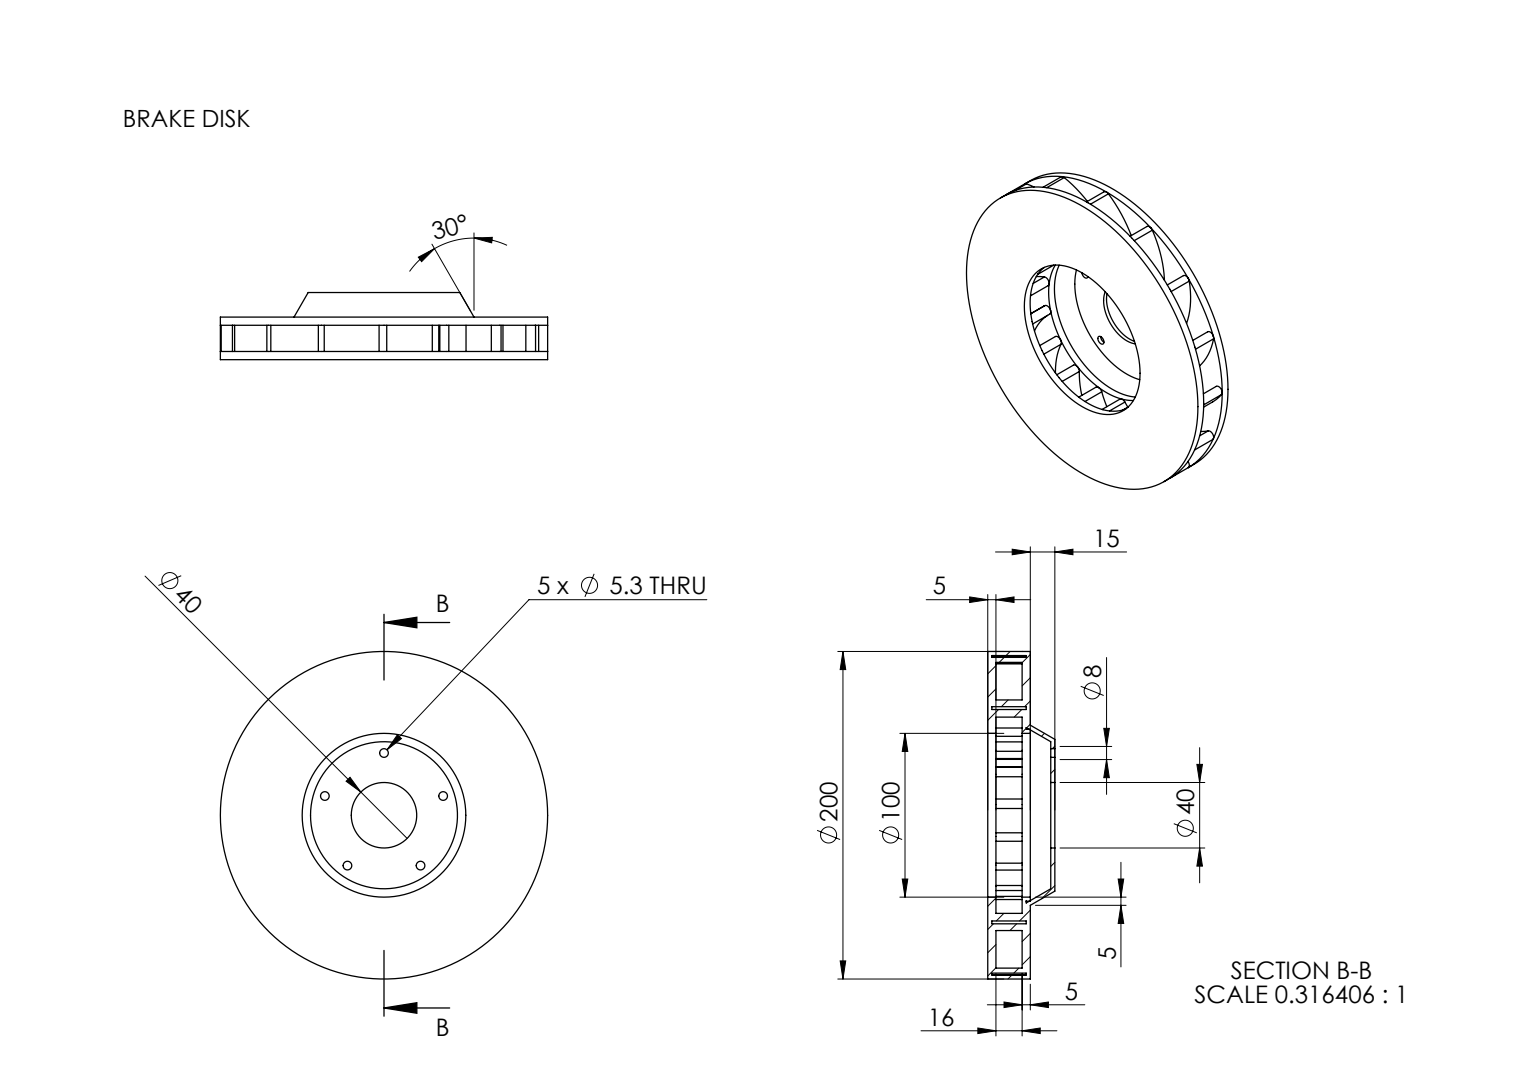
ISO-10303-21;
HEADER;
FILE_DESCRIPTION (('STEP AP214'),
    '1' );
FILE_NAME ('brake disk.step',
    '2026-10-02T06:35:35',
    ( '' ),
    ( '' ),
    'SwSTEP 2.0',
    'SolidWorks 2026',
    '' );
FILE_SCHEMA (( 'AUTOMOTIVE_DESIGN' ));
ENDSEC;

DATA;
#3=DIRECTION ( 'NONE',  ( -1.000000000000000000, 0.000000000000000000, 0.000000000000000000 ) ) ;
#4=ORIENTED_EDGE ( 'NONE', *, *, #5380, .F. ) ;
#6=CIRCLE ( 'NONE', #12861, 63.00000000000000000 ) ;
#7=CARTESIAN_POINT ( 'NONE',  ( 53.06332297728253877, -7.252293700256950082, -10.50000000000000000 ) ) ;
#8=FACE_OUTER_BOUND ( 'NONE', #11130, .T. ) ;
#10=CIRCLE ( 'NONE', #12379, 59.50000000000000711 ) ;
#11=CARTESIAN_POINT ( 'NONE',  ( 0.000000000000000000, 0.000000000000000000, -10.50000000000000000 ) ) ;
#12=AXIS2_PLACEMENT_3D ( 'NONE', #10324, #12760, #3495 ) ;
#13=DIRECTION ( 'NONE',  ( -1.000000000000000000, 0.000000000000000000, 0.000000000000000000 ) ) ;
#14=VERTEX_POINT ( 'NONE', #5600 ) ;
#16=CARTESIAN_POINT ( 'NONE',  ( -9.706953719245875689, -57.06275842387046993, 10.49999999999999822 ) ) ;
#18=AXIS2_PLACEMENT_3D ( 'NONE', #11160, #14736, #14806 ) ;
#19=DIRECTION ( 'NONE',  ( 0.000000000000000000, 0.000000000000000000, 1.000000000000000000 ) ) ;
#20=CIRCLE ( 'NONE', #4639, 50.00000000000000000 ) ;
#25=CARTESIAN_POINT ( 'NONE',  ( -57.06275842387042729, 9.706953719246069312, 10.49999999999999822 ) ) ;
#29=DIRECTION ( 'NONE',  ( 1.000000000000000000, 0.000000000000000000, 0.000000000000000000 ) ) ;
#30=AXIS2_PLACEMENT_3D ( 'NONE', #3946, #7114, #5981 ) ;
#31=DIRECTION ( 'NONE',  ( 1.000000000000000000, 0.000000000000000000, 0.000000000000000000 ) ) ;
#32=DIRECTION ( 'NONE',  ( -1.000000000000000000, 0.000000000000000000, 0.000000000000000000 ) ) ;
#33=AXIS2_PLACEMENT_3D ( 'NONE', #14453, #639, #4058 ) ;
#34=EDGE_LOOP ( 'NONE', ( #1936, #8130, #14973, #10499, #11470, #9709, #14107 ) ) ;
#38=DIRECTION ( 'NONE',  ( -0.000000000000000000, -0.000000000000000000, -1.000000000000000000 ) ) ;
#39=ORIENTED_EDGE ( 'NONE', *, *, #13925, .F. ) ;
#40=AXIS2_PLACEMENT_3D ( 'NONE', #3441, #1165, #12924 ) ;
#41=EDGE_LOOP ( 'NONE', ( #8481, #11440, #8445, #13506, #14760, #3452, #6224, #9398, #1796 ) ) ;
#42=EDGE_CURVE ( 'NONE', #5654, #12729, #7938, .T. ) ;
#43=EDGE_CURVE ( 'NONE', #8906, #2094, #9864, .T. ) ;
#45=AXIS2_PLACEMENT_3D ( 'NONE', #573, #4845, #14470 ) ;
#46=CYLINDRICAL_SURFACE ( 'NONE', #4967, 3.000000000000002665 ) ;
#50=DIRECTION ( 'NONE',  ( 0.000000000000000000, 0.000000000000000000, 1.000000000000000000 ) ) ;
#51=EDGE_LOOP ( 'NONE', ( #11368, #1318, #14890, #12577, #3403 ) ) ;
#53=DIRECTION ( 'NONE',  ( 1.000000000000000000, 0.000000000000000000, 0.000000000000000000 ) ) ;
#54=AXIS2_PLACEMENT_3D ( 'NONE', #13528, #11036, #940 ) ;
#55=ORIENTED_EDGE ( 'NONE', *, *, #8567, .F. ) ;
#56=ORIENTED_EDGE ( 'NONE', *, *, #8508, .F. ) ;
#57=DIRECTION ( 'NONE',  ( 0.000000000000000000, 0.000000000000000000, 1.000000000000000000 ) ) ;
#58=ORIENTED_EDGE ( 'NONE', *, *, #13027, .F. ) ;
#59=AXIS2_PLACEMENT_3D ( 'NONE', #11530, #114, #4460 ) ;
#60=CARTESIAN_POINT ( 'NONE',  ( -69.16568774265545017, 71.53347797788843820, -13.00000000000000178 ) ) ;
#61=CARTESIAN_POINT ( 'NONE',  ( 0.000000000000000000, 0.000000000000000000, -10.50000000000000000 ) ) ;
#62=EDGE_CURVE ( 'NONE', #7405, #1485, #13775, .T. ) ;
#65=CARTESIAN_POINT ( 'NONE',  ( 0.000000000000000000, 0.000000000000000000, -13.00000000000000178 ) ) ;
#66=VECTOR ( 'NONE', #7777, 1000.000000000000000 ) ;
#67=CARTESIAN_POINT ( 'NONE',  ( 66.70695371924546180, 57.06275842387054098, 8.000000000000000000 ) ) ;
#68=CARTESIAN_POINT ( 'NONE',  ( 50.84834283436990177, 14.07862063237912054, -13.00000000000000178 ) ) ;
#70=ORIENTED_EDGE ( 'NONE', *, *, #7162, .T. ) ;
#72=AXIS2_PLACEMENT_3D ( 'NONE', #14916, #10416, #5859 ) ;
#74=LINE ( 'NONE', #12542, #3120 ) ;
#77=AXIS2_PLACEMENT_3D ( 'NONE', #3248, #7868, #12355 ) ;
#78=DIRECTION ( 'NONE',  ( 1.000000000000000000, 0.000000000000000000, 0.000000000000000000 ) ) ;
#79=EDGE_LOOP ( 'NONE', ( #12586, #8672, #6412, #11812, #13520, #7331 ) ) ;
#80=CYLINDRICAL_SURFACE ( 'NONE', #13351, 59.50000000000000000 ) ;
#81=EDGE_CURVE ( 'NONE', #7416, #8383, #7204, .T. ) ;
#83=EDGE_CURVE ( 'NONE', #7502, #10004, #12318, .T. ) ;
#84=DIRECTION ( 'NONE',  ( 0.000000000000000000, 0.000000000000000000, 1.000000000000000000 ) ) ;
#85=CYLINDRICAL_SURFACE ( 'NONE', #14315, 56.99999999999999289 ) ;
#90=ORIENTED_EDGE ( 'NONE', *, *, #1930, .F. ) ;
#96=DIRECTION ( 'NONE',  ( 0.000000000000000000, 0.000000000000000000, -1.000000000000000000 ) ) ;
#98=CIRCLE ( 'NONE', #1556, 2.649999999999992806 ) ;
#100=FACE_OUTER_BOUND ( 'NONE', #3263, .T. ) ;
#102=ORIENTED_EDGE ( 'NONE', *, *, #4360, .F. ) ;
#106=DIRECTION ( 'NONE',  ( -0.000000000000000000, -0.000000000000000000, 1.000000000000000000 ) ) ;
#108=EDGE_LOOP ( 'NONE', ( #5288, #10008 ) ) ;
#109=CIRCLE ( 'NONE', #11524, 3.000000000000004441 ) ;
#110=AXIS2_PLACEMENT_3D ( 'NONE', #13113, #9527, #4007 ) ;
#112=DIRECTION ( 'NONE',  ( 0.000000000000000000, 0.000000000000000000, -1.000000000000000000 ) ) ;
#113=AXIS2_PLACEMENT_3D ( 'NONE', #5450, #3170, #7481 ) ;
#114=DIRECTION ( 'NONE',  ( -0.000000000000000000, -0.000000000000000000, -1.000000000000000000 ) ) ;
#115=ORIENTED_EDGE ( 'NONE', *, *, #13152, .T. ) ;
#116=ORIENTED_EDGE ( 'NONE', *, *, #9973, .T. ) ;
#117=STYLED_ITEM ( 'NONE', ( #11100 ), #4169 ) ;
#118=ORIENTED_EDGE ( 'NONE', *, *, #6384, .T. ) ;
#119=AXIS2_PLACEMENT_3D ( 'NONE', #2152, #13621, #8984 ) ;
#120=DIRECTION ( 'NONE',  ( -1.000000000000000000, 0.000000000000000000, 0.000000000000000000 ) ) ;
#124=CARTESIAN_POINT ( 'NONE',  ( 7.417888187663120192, 52.54657765281190507, -13.00000000000000178 ) ) ;
#125=EDGE_CURVE ( 'NONE', #6463, #5657, #11381, .T. ) ;
#129=ADVANCED_FACE ( 'NONE', ( #13654 ), #8723, .F. ) ;
#130=ORIENTED_EDGE ( 'NONE', *, *, #424, .F. ) ;
#131=EDGE_CURVE ( 'NONE', #9943, #5635, #9786, .T. ) ;
#132=VERTEX_POINT ( 'NONE', #14438 ) ;
#133=EDGE_CURVE ( 'NONE', #4919, #1677, #14989, .T. ) ;
#136=CIRCLE ( 'NONE', #11783, 63.00000000000000000 ) ;
#139=CIRCLE ( 'NONE', #6147, 3.000000000000002665 ) ;
#140=EDGE_LOOP ( 'NONE', ( #7272, #903, #5586, #9223, #6785, #6818 ) ) ;
#142=EDGE_CURVE ( 'NONE', #2335, #4523, #8651, .T. ) ;
#144=VECTOR ( 'NONE', #4829, 1000.000000000000000 ) ;
#145=DIRECTION ( 'NONE',  ( -0.000000000000000000, -0.000000000000000000, 1.000000000000000000 ) ) ;
#146=DIRECTION ( 'NONE',  ( -1.000000000000000000, 0.000000000000000000, 0.000000000000000000 ) ) ;
#147=CIRCLE ( 'NONE', #10081, 0.5000000000000004441 ) ;
#148=DIRECTION ( 'NONE',  ( 1.000000000000000000, 0.000000000000000000, 0.000000000000000000 ) ) ;
#149=SURFACE_STYLE_FILL_AREA ( #5069 ) ;
#151=DIRECTION ( 'NONE',  ( 0.000000000000000000, 0.000000000000000000, 1.000000000000000000 ) ) ;
#152=ORIENTED_EDGE ( 'NONE', *, *, #3887, .F. ) ;
#153=DIRECTION ( 'NONE',  ( -1.000000000000000000, 0.000000000000000000, 0.000000000000000000 ) ) ;
#156=ORIENTED_EDGE ( 'NONE', *, *, #4969, .T. ) ;
#158=ORIENTED_EDGE ( 'NONE', *, *, #13672, .T. ) ;
#160=ORIENTED_EDGE ( 'NONE', *, *, #4028, .F. ) ;
#162=CARTESIAN_POINT ( 'NONE',  ( -52.72775723226775568, 7.383907457638128058, -13.00000000000000178 ) ) ;
#163=DIRECTION ( 'NONE',  ( 1.000000000000000000, 0.000000000000000000, 0.000000000000000000 ) ) ;
#164=CARTESIAN_POINT ( 'NONE',  ( -53.63365512954686665, 9.714003807514082212, 8.000000000000000000 ) ) ;
#165=AXIS2_PLACEMENT_3D ( 'NONE', #7612, #12181, #14531 ) ;
#166=DIRECTION ( 'NONE',  ( -0.000000000000000000, -0.000000000000000000, -1.000000000000000000 ) ) ;
#167=CARTESIAN_POINT ( 'NONE',  ( 36.14014761921570340, 11.74264578624841171, -28.00000000000000000 ) ) ;
#168=ORIENTED_EDGE ( 'NONE', *, *, #2760, .F. ) ;
#169=CARTESIAN_POINT ( 'NONE',  ( 0.000000000000000000, 0.000000000000000000, -10.50000000000000000 ) ) ;
#170=DIRECTION ( 'NONE',  ( 1.000000000000000000, 0.000000000000000000, 0.000000000000000000 ) ) ;
#171=EDGE_CURVE ( 'NONE', #8488, #2518, #8671, .T. ) ;
#172=EDGE_CURVE ( 'NONE', #8464, #345, #2401, .T. ) ;
#174=CARTESIAN_POINT ( 'NONE',  ( 33.48561063518626923, -47.21331623427104063, 10.49999999999999822 ) ) ;
#175=ORIENTED_EDGE ( 'NONE', *, *, #2159, .T. ) ;
#176=CARTESIAN_POINT ( 'NONE',  ( -45.96504489225991819, 23.50071946824089153, -8.000000000000000000 ) ) ;
#178=DIRECTION ( 'NONE',  ( 1.000000000000000000, 0.000000000000000000, -0.000000000000000000 ) ) ;
#180=EDGE_CURVE ( 'NONE', #2333, #2935, #11831, .T. ) ;
#181=CARTESIAN_POINT ( 'NONE',  ( 70.71067811865488295, 70.71067811865464137, 8.000000000000000000 ) ) ;
#182=DIRECTION ( 'NONE',  ( -0.000000000000000000, -0.000000000000000000, -1.000000000000000000 ) ) ;
#184=PLANE ( 'NONE',  #4038 ) ;
#185=DIRECTION ( 'NONE',  ( 1.000000000000000000, 0.000000000000000000, 0.000000000000000000 ) ) ;
#186=ADVANCED_FACE ( 'NONE', ( #285 ), #5969, .F. ) ;
#187=DIRECTION ( 'NONE',  ( 0.000000000000000000, 0.000000000000000000, -1.000000000000000000 ) ) ;
#188=ORIENTED_EDGE ( 'NONE', *, *, #4452, .F. ) ;
#189=ORIENTED_EDGE ( 'NONE', *, *, #647, .F. ) ;
#190=ORIENTED_EDGE ( 'NONE', *, *, #13352, .T. ) ;
#191=DIRECTION ( 'NONE',  ( -0.000000000000000000, -0.000000000000000000, -1.000000000000000000 ) ) ;
#192=DIRECTION ( 'NONE',  ( -0.000000000000000000, -0.000000000000000000, 1.000000000000000000 ) ) ;
#193=DIRECTION ( 'NONE',  ( 0.000000000000000000, 0.000000000000000000, 1.000000000000000000 ) ) ;
#195=CARTESIAN_POINT ( 'NONE',  ( 92.61631465359491244, 37.12029293941346708, -13.00000000000000178 ) ) ;
#196=ORIENTED_EDGE ( 'NONE', *, *, #12416, .F. ) ;
#197=VERTEX_POINT ( 'NONE', #8248 ) ;
#198=VERTEX_POINT ( 'NONE', #2479 ) ;
#199=CARTESIAN_POINT ( 'NONE',  ( 43.30127018922200222, -24.99999999999988276, -8.000000000000000000 ) ) ;
#202=ORIENTED_EDGE ( 'NONE', *, *, #1757, .T. ) ;
#203=VERTEX_POINT ( 'NONE', #9455 ) ;
#204=DIRECTION ( 'NONE',  ( -0.000000000000000000, -0.000000000000000000, -1.000000000000000000 ) ) ;
#206=EDGE_CURVE ( 'NONE', #7611, #11559, #11845, .T. ) ;
#207=CARTESIAN_POINT ( 'NONE',  ( -57.06275842387042729, 9.706953719246069312, -8.000000000000000000 ) ) ;
#208=DIRECTION ( 'NONE',  ( -1.000000000000000000, 0.000000000000000000, 0.000000000000000000 ) ) ;
#209=ADVANCED_FACE ( 'NONE', ( #8178 ), #13040, .T. ) ;
#211=DIRECTION ( 'NONE',  ( 0.000000000000000000, 0.000000000000000000, -1.000000000000000000 ) ) ;
#212=VERTEX_POINT ( 'NONE', #10456 ) ;
#213=LINE ( 'NONE', #4355, #3743 ) ;
#214=CARTESIAN_POINT ( 'NONE',  ( -89.89283556784485540, 37.53686968382331202, 10.49999999999999822 ) ) ;
#215=VERTEX_POINT ( 'NONE', #4771 ) ;
#217=ORIENTED_EDGE ( 'NONE', *, *, #892, .F. ) ;
#218=VERTEX_POINT ( 'NONE', #1279 ) ;
#219=VERTEX_POINT ( 'NONE', #12746 ) ;
#221=DIRECTION ( 'NONE',  ( 0.000000000000000000, 0.000000000000000000, -1.000000000000000000 ) ) ;
#222=AXIS2_PLACEMENT_3D ( 'NONE', #233, #10789, #392 ) ;
#224=EDGE_LOOP ( 'NONE', ( #11298, #11985, #10533, #2386, #7022, #5370 ) ) ;
#225=EDGE_CURVE ( 'NONE', #11976, #1441, #7021, .T. ) ;
#228=CARTESIAN_POINT ( 'NONE',  ( 0.000000000000000000, 0.000000000000000000, 10.50000000000000000 ) ) ;
#229=DIRECTION ( 'NONE',  ( -0.000000000000000000, -0.000000000000000000, 1.000000000000000000 ) ) ;
#232=CIRCLE ( 'NONE', #11153, 59.50000000000000000 ) ;
#233=CARTESIAN_POINT ( 'NONE',  ( 6.917888187663118416, 52.54657765281190507, -13.00000000000000178 ) ) ;
#235=CIRCLE ( 'NONE', #7737, 3.000000000000002665 ) ;
#236=DIRECTION ( 'NONE',  ( 0.000000000000000000, 0.000000000000000000, -1.000000000000000000 ) ) ;
#237=ORIENTED_EDGE ( 'NONE', *, *, #10239, .T. ) ;
#238=VECTOR ( 'NONE', #6357, 1000.000000000000000 ) ;
#239=CARTESIAN_POINT ( 'NONE',  ( 0.000000000000000000, 0.000000000000000000, -13.00000000000000178 ) ) ;
#240=CYLINDRICAL_SURFACE ( 'NONE', #5888, 0.5000000000000004441 ) ;
#241=DIRECTION ( 'NONE',  ( 0.000000000000000000, 0.000000000000000000, 1.000000000000000000 ) ) ;
#242=AXIS2_PLACEMENT_3D ( 'NONE', #11255, #4428, #1840 ) ;
#244=DIRECTION ( 'NONE',  ( 0.000000000000000000, 0.000000000000000000, 1.000000000000000000 ) ) ;
#246=VECTOR ( 'NONE', #11341, 1000.000000000000000 ) ;
#247=CARTESIAN_POINT ( 'NONE',  ( 0.000000000000000000, 0.000000000000000000, -13.00000000000000178 ) ) ;
#248=AXIS2_PLACEMENT_3D ( 'NONE', #2313, #11658, #11591 ) ;
#249=EDGE_LOOP ( 'NONE', ( #12812, #11025, #8242, #14279, #562, #14719, #2020, #11276, #2397 ) ) ;
#250=DIRECTION ( 'NONE',  ( -0.000000000000000000, -0.000000000000000000, 1.000000000000000000 ) ) ;
#251=DIRECTION ( 'NONE',  ( 0.000000000000000000, 0.000000000000000000, -1.000000000000000000 ) ) ;
#252=EDGE_CURVE ( 'NONE', #915, #5997, #13054, .T. ) ;
#256=CIRCLE ( 'NONE', #11911, 100.0000000000000000 ) ;
#258=ORIENTED_EDGE ( 'NONE', *, *, #4361, .T. ) ;
#260=PLANE ( 'NONE',  #2332 ) ;
#262=LINE ( 'NONE', #9512, #1094 ) ;
#263=AXIS2_PLACEMENT_3D ( 'NONE', #3425, #1153, #13759 ) ;
#264=CIRCLE ( 'NONE', #5603, 100.0000000000000000 ) ;
#267=ORIENTED_EDGE ( 'NONE', *, *, #14506, .F. ) ;
#268=AXIS2_PLACEMENT_3D ( 'NONE', #7487, #1663, #9475 ) ;
#269=ORIENTED_EDGE ( 'NONE', *, *, #1652, .T. ) ;
#270=AXIS2_PLACEMENT_3D ( 'NONE', #9018, #6504, #12227 ) ;
#271=DIRECTION ( 'NONE',  ( -0.000000000000000000, -0.000000000000000000, 1.000000000000000000 ) ) ;
#272=AXIS2_PLACEMENT_3D ( 'NONE', #7169, #13184, #425 ) ;
#275=EDGE_CURVE ( 'NONE', #7416, #12316, #7948, .T. ) ;
#279=CYLINDRICAL_SURFACE ( 'NONE', #11305, 0.5000000000000004441 ) ;
#280=ORIENTED_EDGE ( 'NONE', *, *, #6420, .T. ) ;
#281=ORIENTED_EDGE ( 'NONE', *, *, #10347, .F. ) ;
#282=ORIENTED_EDGE ( 'NONE', *, *, #7023, .T. ) ;
#283=ORIENTED_EDGE ( 'NONE', *, *, #14608, .F. ) ;
#284=CARTESIAN_POINT ( 'NONE',  ( -9.706953719245875689, -57.06275842387046993, -8.000000000000000000 ) ) ;
#285=FACE_OUTER_BOUND ( 'NONE', #6940, .T. ) ;
#286=CIRCLE ( 'NONE', #8760, 2.649999999999985700 ) ;
#287=CARTESIAN_POINT ( 'NONE',  ( -42.04772703543551415, -32.26435573746212526, 8.000000000000000000 ) ) ;
#288=EDGE_LOOP ( 'NONE', ( #5939, #663, #3564, #6991, #11925, #8225 ) ) ;
#291=DIRECTION ( 'NONE',  ( -0.000000000000000000, -0.000000000000000000, 1.000000000000000000 ) ) ;
#292=EDGE_LOOP ( 'NONE', ( #2950, #14683, #2755, #9795, #13525 ) ) ;
#295=DIRECTION ( 'NONE',  ( 0.000000000000000000, 0.000000000000000000, -1.000000000000000000 ) ) ;
#296=CARTESIAN_POINT ( 'NONE',  ( 0.000000000000000000, 0.000000000000000000, 0.000000000000000000 ) ) ;
#297=VERTEX_POINT ( 'NONE', #3559 ) ;
#299=DIRECTION ( 'NONE',  ( 0.000000000000000000, 0.000000000000000000, -1.000000000000000000 ) ) ;
#301=CYLINDRICAL_SURFACE ( 'NONE', #14086, 3.000000000000004441 ) ;
#302=EDGE_CURVE ( 'NONE', #8589, #2566, #1412, .T. ) ;
#303=VERTEX_POINT ( 'NONE', #6955 ) ;
#305=ORIENTED_EDGE ( 'NONE', *, *, #10378, .T. ) ;
#311=DIRECTION ( 'NONE',  ( -1.000000000000000000, 0.000000000000000000, 0.000000000000000000 ) ) ;
#312=DIRECTION ( 'NONE',  ( 0.000000000000000000, 0.000000000000000000, 1.000000000000000000 ) ) ;
#314=CARTESIAN_POINT ( 'NONE',  ( -89.61631465359519666, -37.12029293941281338, 8.000000000000000000 ) ) ;
#317=FACE_OUTER_BOUND ( 'NONE', #3117, .T. ) ;
#318=CIRCLE ( 'NONE', #5648, 59.50000000000000000 ) ;
#321=EDGE_CURVE ( 'NONE', #8628, #10615, #10617, .T. ) ;
#322=ADVANCED_FACE ( 'NONE', ( #2789 ), #4156, .F. ) ;
#324=DIRECTION ( 'NONE',  ( -1.000000000000000000, 0.000000000000000000, 0.000000000000000000 ) ) ;
#325=PLANE ( 'NONE',  #8368 ) ;
#327=ORIENTED_EDGE ( 'NONE', *, *, #5681, .F. ) ;
#328=AXIS2_PLACEMENT_3D ( 'NONE', #10103, #12541, #12462 ) ;
#329=ORIENTED_EDGE ( 'NONE', *, *, #3965, .F. ) ;
#333=DIRECTION ( 'NONE',  ( 0.000000000000000000, 0.000000000000000000, 1.000000000000000000 ) ) ;
#334=CIRCLE ( 'NONE', #2033, 56.99999999999999289 ) ;
#336=CARTESIAN_POINT ( 'NONE',  ( -9.706953719245875689, -57.06275842387046993, -13.00000000000000178 ) ) ;
#338=DIRECTION ( 'NONE',  ( 0.000000000000000000, 0.000000000000000000, 1.000000000000000000 ) ) ;
#339=DIRECTION ( 'NONE',  ( 0.000000000000000000, 0.000000000000000000, 1.000000000000000000 ) ) ;
#340=AXIS2_PLACEMENT_3D ( 'NONE', #3361, #10273, #9197 ) ;
#343=CIRCLE ( 'NONE', #13938, 3.000000000000002665 ) ;
#345=VERTEX_POINT ( 'NONE', #11064 ) ;
#346=DIRECTION ( 'NONE',  ( 1.000000000000000000, 0.000000000000000000, 0.000000000000000000 ) ) ;
#347=ORIENTED_EDGE ( 'NONE', *, *, #12989, .T. ) ;
#348=EDGE_CURVE ( 'NONE', #6889, #6138, #12080, .T. ) ;
#351=DIRECTION ( 'NONE',  ( -1.000000000000000000, 0.000000000000000000, 0.000000000000000000 ) ) ;
#353=DIRECTION ( 'NONE',  ( 0.000000000000000000, 0.000000000000000000, 1.000000000000000000 ) ) ;
#354=AXIS2_PLACEMENT_3D ( 'NONE', #14127, #13062, #5918 ) ;
#356=AXIS2_PLACEMENT_3D ( 'NONE', #3246, #11748, #1413 ) ;
#358=EDGE_LOOP ( 'NONE', ( #1201, #1005, #6170, #12433, #283 ) ) ;
#359=DIRECTION ( 'NONE',  ( 0.000000000000000000, 0.000000000000000000, 1.000000000000000000 ) ) ;
#361=DIRECTION ( 'NONE',  ( 0.000000000000000000, 0.000000000000000000, 1.000000000000000000 ) ) ;
#363=EDGE_CURVE ( 'NONE', #10590, #2920, #12567, .T. ) ;
#364=AXIS2_PLACEMENT_3D ( 'NONE', #5973, #204, #2567 ) ;
#365=ADVANCED_FACE ( 'NONE', ( #7410 ), #14399, .T. ) ;
#367=CARTESIAN_POINT ( 'NONE',  ( -30.80502811811232888, -49.00442420935981147, -8.000000000000000000 ) ) ;
#368=CIRCLE ( 'NONE', #4978, 53.55662432702593634 ) ;
#371=CARTESIAN_POINT ( 'NONE',  ( -9.706953719245875689, -57.06275842387046993, -13.00000000000000178 ) ) ;
#374=EDGE_CURVE ( 'NONE', #219, #7084, #3764, .T. ) ;
#375=EDGE_LOOP ( 'NONE', ( #14396, #4852, #5447, #9385 ) ) ;
#378=ORIENTED_EDGE ( 'NONE', *, *, #11049, .T. ) ;
#380=CIRCLE ( 'NONE', #5704, 59.50000000000000000 ) ;
#381=ORIENTED_EDGE ( 'NONE', *, *, #5819, .F. ) ;
#384=CARTESIAN_POINT ( 'NONE',  ( 13.71740939043365337, -51.19406879332061067, -10.50000000000000000 ) ) ;
#386=CIRCLE ( 'NONE', #14206, 0.5000000000000043299 ) ;
#387=DIRECTION ( 'NONE',  ( 1.000000000000000000, 9.130123557772668088E-16, 0.000000000000000000 ) ) ;
#388=CARTESIAN_POINT ( 'NONE',  ( 6.451868917687939131, 52.36539807335604024, -13.00000000000000178 ) ) ;
#390=CARTESIAN_POINT ( 'NONE',  ( 0.000000000000000000, 0.000000000000000000, -10.50000000000000000 ) ) ;
#392=DIRECTION ( 'NONE',  ( 1.000000000000000000, 0.000000000000000000, 0.000000000000000000 ) ) ;
#393=ORIENTED_EDGE ( 'NONE', *, *, #11619, .F. ) ;
#396=ORIENTED_EDGE ( 'NONE', *, *, #13309, .T. ) ;
#399=DIRECTION ( 'NONE',  ( 1.000000000000000000, 0.000000000000000000, 0.000000000000000000 ) ) ;
#400=CARTESIAN_POINT ( 'NONE',  ( 26.24999999999972289, 45.46633369868319363, -10.50000000000000000 ) ) ;
#401=EDGE_LOOP ( 'NONE', ( #4330, #13491, #1579, #14951 ) ) ;
#402=ORIENTED_EDGE ( 'NONE', *, *, #8056, .F. ) ;
#403=AXIS2_PLACEMENT_3D ( 'NONE', #16, #4438, #10272 ) ;
#404=EDGE_CURVE ( 'NONE', #6283, #13552, #12722, .T. ) ;
#406=VERTEX_POINT ( 'NONE', #4008 ) ;
#407=CARTESIAN_POINT ( 'NONE',  ( -45.89934640057513349, 26.50000000000019540, 10.49999999999999822 ) ) ;
#408=EDGE_CURVE ( 'NONE', #8250, #5635, #109, .T. ) ;
#409=DIRECTION ( 'NONE',  ( 1.000000000000000000, 0.000000000000000000, -0.000000000000000000 ) ) ;
#410=ADVANCED_FACE ( 'NONE', ( #6410 ), #1721, .F. ) ;
#413=FACE_OUTER_BOUND ( 'NONE', #6825, .T. ) ;
#414=ORIENTED_EDGE ( 'NONE', *, *, #11571, .T. ) ;
#415=DIRECTION ( 'NONE',  ( 0.000000000000000000, 0.000000000000000000, -1.000000000000000000 ) ) ;
#416=EDGE_CURVE ( 'NONE', #11469, #12633, #6883, .T. ) ;
#417=FACE_OUTER_BOUND ( 'NONE', #10979, .T. ) ;
#418=CARTESIAN_POINT ( 'NONE',  ( -32.06294366074467206, 42.50536573064442081, -13.00000000000000178 ) ) ;
#419=ORIENTED_EDGE ( 'NONE', *, *, #13917, .T. ) ;
#423=DIRECTION ( 'NONE',  ( -0.000000000000000000, -0.000000000000000000, -1.000000000000000000 ) ) ;
#424=EDGE_CURVE ( 'NONE', #5520, #12576, #13268, .T. ) ;
#425=DIRECTION ( 'NONE',  ( 1.000000000000000000, 0.000000000000000000, 0.000000000000000000 ) ) ;
#426=CARTESIAN_POINT ( 'NONE',  ( 26.49999999999971578, 45.89934640057541060, 8.000000000000000000 ) ) ;
#429=ORIENTED_EDGE ( 'NONE', *, *, #374, .T. ) ;
#430=DIRECTION ( 'NONE',  ( 0.000000000000000000, 0.000000000000000000, 1.000000000000000000 ) ) ;
#431=DIRECTION ( 'NONE',  ( 0.000000000000000000, 0.000000000000000000, 1.000000000000000000 ) ) ;
#432=LINE ( 'NONE', #14181, #7837 ) ;
#433=ORIENTED_EDGE ( 'NONE', *, *, #10895, .F. ) ;
#435=ORIENTED_EDGE ( 'NONE', *, *, #12207, .T. ) ;
#436=CARTESIAN_POINT ( 'NONE',  ( -12.86891638962156215, 56.43380494353993271, -13.00000000000000178 ) ) ;
#437=ORIENTED_EDGE ( 'NONE', *, *, #14604, .T. ) ;
#439=DIRECTION ( 'NONE',  ( 0.000000000000000000, 0.000000000000000000, 1.000000000000000000 ) ) ;
#440=FILL_AREA_STYLE_COLOUR ( '', #7271 ) ;
#441=EDGE_CURVE ( 'NONE', #2510, #5889, #6160, .T. ) ;
#442=DIRECTION ( 'NONE',  ( 0.000000000000000000, 0.000000000000000000, 1.000000000000000000 ) ) ;
#446=DIRECTION ( 'NONE',  ( 1.000000000000000000, 0.000000000000000000, 0.000000000000000000 ) ) ;
#447=ADVANCED_FACE ( 'NONE', ( #10901 ), #4998, .F. ) ;
#448=ORIENTED_EDGE ( 'NONE', *, *, #10981, .T. ) ;
#449=EDGE_LOOP ( 'NONE', ( #13543, #13399, #11232, #10086 ) ) ;
#451=EDGE_CURVE ( 'NONE', #5954, #7016, #6898, .T. ) ;
#452=VERTEX_POINT ( 'NONE', #4459 ) ;
#458=EDGE_CURVE ( 'NONE', #8255, #4053, #4312, .T. ) ;
#459=ORIENTED_EDGE ( 'NONE', *, *, #7753, .T. ) ;
#461=EDGE_LOOP ( 'NONE', ( #5076, #2101 ) ) ;
#462=DIRECTION ( 'NONE',  ( 0.000000000000000000, 0.000000000000000000, 1.000000000000000000 ) ) ;
#464=CARTESIAN_POINT ( 'NONE',  ( -0.2790467552932288098, -97.41488903138106537, -13.00000000000000178 ) ) ;
#466=CYLINDRICAL_SURFACE ( 'NONE', #5882, 0.5000000000000004441 ) ;
#468=LINE ( 'NONE', #10724, #10763 ) ;
#469=VERTEX_POINT ( 'NONE', #8918 ) ;
#472=ORIENTED_EDGE ( 'NONE', *, *, #3041, .F. ) ;
#473=DIRECTION ( 'NONE',  ( -1.000000000000000000, 0.000000000000000000, 0.000000000000000000 ) ) ;
#476=DIRECTION ( 'NONE',  ( 0.000000000000000000, 0.000000000000000000, 1.000000000000000000 ) ) ;
#477=CARTESIAN_POINT ( 'NONE',  ( -32.26435573746199736, 42.04772703543562073, -13.00000000000000178 ) ) ;
#480=DIRECTION ( 'NONE',  ( 0.000000000000000000, 0.000000000000000000, -1.000000000000000000 ) ) ;
#481=DIRECTION ( 'NONE',  ( 1.000000000000000000, 0.000000000000000000, 0.000000000000000000 ) ) ;
#482=CIRCLE ( 'NONE', #5802, 3.000000000000004441 ) ;
#483=FACE_OUTER_BOUND ( 'NONE', #10528, .T. ) ;
#484=CIRCLE ( 'NONE', #8961, 53.55662432702593634 ) ;
#486=CIRCLE ( 'NONE', #10422, 3.000000000000002665 ) ;
#487=VECTOR ( 'NONE', #2049, 1000.000000000000000 ) ;
#488=EDGE_LOOP ( 'NONE', ( #55, #3617, #4993, #56, #14251, #1002 ) ) ;
#489=DIRECTION ( 'NONE',  ( 0.000000000000000000, 0.000000000000000000, 1.000000000000000000 ) ) ;
#490=VERTEX_POINT ( 'NONE', #9989 ) ;
#491=CARTESIAN_POINT ( 'NONE',  ( -50.84834283437000835, -14.07862063237876704, -10.50000000000000000 ) ) ;
#492=CARTESIAN_POINT ( 'NONE',  ( 6.917888187663118416, 52.54657765281190507, -8.000000000000000000 ) ) ;
#493=ORIENTED_EDGE ( 'NONE', *, *, #10102, .F. ) ;
#494=AXIS2_PLACEMENT_3D ( 'NONE', #3812, #6062, #12011 ) ;
#498=DIRECTION ( 'NONE',  ( 0.000000000000000000, 0.000000000000000000, -1.000000000000000000 ) ) ;
#499=CIRCLE ( 'NONE', #8254, 100.0000000000000000 ) ;
#501=ORIENTED_EDGE ( 'NONE', *, *, #6565, .F. ) ;
#502=( GEOMETRIC_REPRESENTATION_CONTEXT ( 3 ) GLOBAL_UNCERTAINTY_ASSIGNED_CONTEXT ( ( #12183 ) ) GLOBAL_UNIT_ASSIGNED_CONTEXT ( ( #14644, #1878, #7565 ) ) REPRESENTATION_CONTEXT ( 'NONE', 'WORKASPACE' ) );
#503=DIRECTION ( 'NONE',  ( 1.000000000000000000, 0.000000000000000000, 0.000000000000000000 ) ) ;
#504=DIRECTION ( 'NONE',  ( -1.000000000000000000, 0.000000000000000000, 0.000000000000000000 ) ) ;
#505=CARTESIAN_POINT ( 'NONE',  ( -39.04772703543551415, -32.26435573746212526, -13.00000000000000178 ) ) ;
#507=EDGE_CURVE ( 'NONE', #1441, #8710, #8120, .T. ) ;
#509=AXIS2_PLACEMENT_3D ( 'NONE', #5543, #4271, #3272 ) ;
#510=AXIS2_PLACEMENT_3D ( 'NONE', #2408, #4557, #10392 ) ;
#511=VERTEX_POINT ( 'NONE', #12427 ) ;
#512=CARTESIAN_POINT ( 'NONE',  ( 49.00442420935993226, -30.80502811811213704, -10.50000000000000000 ) ) ;
#516=CYLINDRICAL_SURFACE ( 'NONE', #8350, 0.5000000000000004441 ) ;
#519=ORIENTED_EDGE ( 'NONE', *, *, #12444, .F. ) ;
#520=CARTESIAN_POINT ( 'NONE',  ( -89.61631465359519666, -37.12029293941281338, -8.000000000000000000 ) ) ;
#521=CIRCLE ( 'NONE', #9000, 0.5000000000000073275 ) ;
#522=LINE ( 'NONE', #1661, #13817 ) ;
#523=ORIENTED_EDGE ( 'NONE', *, *, #3292, .T. ) ;
#524=CARTESIAN_POINT ( 'NONE',  ( -12.86891638962156215, 56.43380494353993271, 8.000000000000000000 ) ) ;
#526=ORIENTED_EDGE ( 'NONE', *, *, #8016, .F. ) ;
#528=CARTESIAN_POINT ( 'NONE',  ( -32.26435573746199736, 42.04772703543562073, -10.50000000000000000 ) ) ;
#533=VECTOR ( 'NONE', #12822, 1000.000000000000000 ) ;
#534=LINE ( 'NONE', #6277, #10550 ) ;
#535=DIRECTION ( 'NONE',  ( 0.000000000000000000, 0.000000000000000000, -1.000000000000000000 ) ) ;
#536=DIRECTION ( 'NONE',  ( 0.000000000000000000, 0.000000000000000000, 1.000000000000000000 ) ) ;
#538=ORIENTED_EDGE ( 'NONE', *, *, #13672, .F. ) ;
#539=EDGE_CURVE ( 'NONE', #11742, #10704, #3490, .T. ) ;
#540=ORIENTED_EDGE ( 'NONE', *, *, #9437, .T. ) ;
#542=CARTESIAN_POINT ( 'NONE',  ( 0.000000000000000000, 0.000000000000000000, 8.000000000000000000 ) ) ;
#545=CARTESIAN_POINT ( 'NONE',  ( 52.50000000000000711, -6.429395695523604744E-15, -13.00000000000000178 ) ) ;
#546=EDGE_CURVE ( 'NONE', #8869, #1076, #7933, .T. ) ;
#547=DIRECTION ( 'NONE',  ( 0.000000000000000000, 0.000000000000000000, 1.000000000000000000 ) ) ;
#548=ADVANCED_FACE ( 'NONE', ( #14712 ), #5581, .F. ) ;
#549=EDGE_LOOP ( 'NONE', ( #11916, #5570, #5078, #10453 ) ) ;
#553=CIRCLE ( 'NONE', #2254, 53.55662432702593634 ) ;
#554=DIRECTION ( 'NONE',  ( 0.000000000000000000, 0.000000000000000000, -1.000000000000000000 ) ) ;
#555=CARTESIAN_POINT ( 'NONE',  ( -99.48933418828642061, 1.674280531760366397, -13.00000000000000178 ) ) ;
#556=CARTESIAN_POINT ( 'NONE',  ( -10.71740939043329099, 51.19406879332069593, -8.000000000000000000 ) ) ;
#557=DIRECTION ( 'NONE',  ( 0.000000000000000000, 0.000000000000000000, 1.000000000000000000 ) ) ;
#558=CARTESIAN_POINT ( 'NONE',  ( -49.54657765281192638, 6.917888187662934563, -13.00000000000000178 ) ) ;
#559=EDGE_CURVE ( 'NONE', #13798, #2876, #5911, .T. ) ;
#561=AXIS2_PLACEMENT_3D ( 'NONE', #11375, #4319, #5377 ) ;
#562=ORIENTED_EDGE ( 'NONE', *, *, #918, .T. ) ;
#563=DIRECTION ( 'NONE',  ( 1.000000000000000000, 0.000000000000000000, -0.000000000000000000 ) ) ;
#565=CIRCLE ( 'NONE', #11245, 3.000000000000002665 ) ;
#568=ORIENTED_EDGE ( 'NONE', *, *, #9060, .T. ) ;
#571=VERTEX_POINT ( 'NONE', #13948 ) ;
#572=CARTESIAN_POINT ( 'NONE',  ( -45.89934640057513349, 26.50000000000019540, -13.00000000000000178 ) ) ;
#573=CARTESIAN_POINT ( 'NONE',  ( 0.000000000000000000, 0.000000000000000000, 10.50000000000000000 ) ) ;
#574=AXIS2_PLACEMENT_3D ( 'NONE', #13413, #6560, #8919 ) ;
#580=ORIENTED_EDGE ( 'NONE', *, *, #4644, .T. ) ;
#581=AXIS2_PLACEMENT_3D ( 'NONE', #4135, #2990, #8826 ) ;
#582=CARTESIAN_POINT ( 'NONE',  ( 33.48561063518626923, -47.21331623427104063, -10.50000000000000000 ) ) ;
#583=CARTESIAN_POINT ( 'NONE',  ( -2.449293598294700991E-16, 97.00000000000000000, -8.000000000000000000 ) ) ;
#585=CARTESIAN_POINT ( 'NONE',  ( 92.38795325112850776, -38.26834323650940206, -8.000000000000000000 ) ) ;
#586=ORIENTED_EDGE ( 'NONE', *, *, #14556, .F. ) ;
#587=ORIENTED_EDGE ( 'NONE', *, *, #12141, .T. ) ;
#588=DIRECTION ( 'NONE',  ( 0.000000000000000000, 0.000000000000000000, -1.000000000000000000 ) ) ;
#589=ORIENTED_EDGE ( 'NONE', *, *, #14748, .F. ) ;
#590=AXIS2_PLACEMENT_3D ( 'NONE', #2229, #4657, #11799 ) ;
#591=CIRCLE ( 'NONE', #10537, 57.00000000000000000 ) ;
#592=CYLINDRICAL_SURFACE ( 'NONE', #2055, 60.50000000000000000 ) ;
#593=EDGE_CURVE ( 'NONE', #13762, #8214, #2527, .T. ) ;
#594=AXIS2_PLACEMENT_3D ( 'NONE', #4541, #9080, #9230 ) ;
#595=EDGE_CURVE ( 'NONE', #13877, #3975, #10764, .T. ) ;
#596=CARTESIAN_POINT ( 'NONE',  ( -49.00442420935969778, 30.80502811811250297, -8.000000000000000000 ) ) ;
#598=ADVANCED_FACE ( 'NONE', ( #5949 ), #10588, .T. ) ;
#600=DIRECTION ( 'NONE',  ( -0.000000000000000000, -0.000000000000000000, -1.000000000000000000 ) ) ;
#601=EDGE_LOOP ( 'NONE', ( #6163, #9721, #13299, #11953, #1874, #3782 ) ) ;
#602=EDGE_CURVE ( 'NONE', #14931, #14224, #3501, .T. ) ;
#603=DIRECTION ( 'NONE',  ( 1.000000000000000000, 0.000000000000000000, 0.000000000000000000 ) ) ;
#605=CIRCLE ( 'NONE', #4490, 0.5000000000000004441 ) ;
#606=VECTOR ( 'NONE', #13411, 1000.000000000000000 ) ;
#607=CIRCLE ( 'NONE', #6899, 50.00000000000000000 ) ;
#608=VECTOR ( 'NONE', #7160, 1000.000000000000000 ) ;
#611=AXIS2_PLACEMENT_3D ( 'NONE', #784, #938, #10032 ) ;
#612=ORIENTED_EDGE ( 'NONE', *, *, #6268, .F. ) ;
#614=CARTESIAN_POINT ( 'NONE',  ( -45.96504489225991819, 23.50071946824089153, -13.00000000000000178 ) ) ;
#616=DIRECTION ( 'NONE',  ( -1.000000000000000000, 1.749300984178292964E-15, 0.000000000000000000 ) ) ;
#617=CARTESIAN_POINT ( 'NONE',  ( -39.61975340586619865, -91.27544013909722764, -8.000000000000000000 ) ) ;
#618=FACE_OUTER_BOUND ( 'NONE', #7850, .T. ) ;
#619=EDGE_CURVE ( 'NONE', #5663, #6408, #262, .T. ) ;
#620=AXIS2_PLACEMENT_3D ( 'NONE', #14211, #2814, #7278 ) ;
#621=FACE_OUTER_BOUND ( 'NONE', #249, .T. ) ;
#622=ORIENTED_EDGE ( 'NONE', *, *, #8927, .F. ) ;
#624=VECTOR ( 'NONE', #11823, 1000.000000000000000 ) ;
#626=DIRECTION ( 'NONE',  ( 1.000000000000000000, 0.000000000000000000, 0.000000000000000000 ) ) ;
#630=EDGE_LOOP ( 'NONE', ( #6480, #10245, #8845, #11971, #6286 ) ) ;
#632=ORIENTED_EDGE ( 'NONE', *, *, #5312, .F. ) ;
#633=CARTESIAN_POINT ( 'NONE',  ( -34.12029293941441210, -89.61631465359452875, -13.00000000000000178 ) ) ;
#634=ORIENTED_EDGE ( 'NONE', *, *, #8025, .T. ) ;
#637=DIRECTION ( 'NONE',  ( 0.000000000000000000, 0.000000000000000000, 1.000000000000000000 ) ) ;
#639=DIRECTION ( 'NONE',  ( 0.000000000000000000, 0.000000000000000000, 1.000000000000000000 ) ) ;
#640=CARTESIAN_POINT ( 'NONE',  ( 68.58935777509475429, -68.58935777509547904, -13.00000000000000178 ) ) ;
#642=EDGE_CURVE ( 'NONE', #4677, #13856, #12948, .T. ) ;
#644=ADVANCED_FACE ( 'NONE', ( #9293 ), #3542, .F. ) ;
#645=LINE ( 'NONE', #13535, #6936 ) ;
#647=EDGE_CURVE ( 'NONE', #11532, #9553, #13946, .T. ) ;
#648=CARTESIAN_POINT ( 'NONE',  ( -50.69406879332065330, -13.71740939043347041, 10.49999999999999822 ) ) ;
#649=AXIS2_PLACEMENT_3D ( 'NONE', #4532, #12650, #12572 ) ;
#651=EDGE_CURVE ( 'NONE', #7439, #5954, #12735, .T. ) ;
#652=DIRECTION ( 'NONE',  ( -1.000000000000000000, 0.000000000000000000, 0.000000000000000000 ) ) ;
#653=ORIENTED_EDGE ( 'NONE', *, *, #14248, .F. ) ;
#654=CIRCLE ( 'NONE', #3811, 60.50000000000000000 ) ;
#655=CARTESIAN_POINT ( 'NONE',  ( 0.000000000000000000, 0.000000000000000000, -10.50000000000000000 ) ) ;
#656=CARTESIAN_POINT ( 'NONE',  ( -56.43380494354004639, -12.86891638962099549, -10.50000000000000000 ) ) ;
#662=CIRCLE ( 'NONE', #12537, 60.50000000000000000 ) ;
#663=ORIENTED_EDGE ( 'NONE', *, *, #14844, .F. ) ;
#665=EDGE_CURVE ( 'NONE', #7876, #8214, #5795, .T. ) ;
#668=DIRECTION ( 'NONE',  ( 0.000000000000000000, 0.000000000000000000, 1.000000000000000000 ) ) ;
#669=VERTEX_POINT ( 'NONE', #7079 ) ;
#670=ORIENTED_EDGE ( 'NONE', *, *, #8944, .T. ) ;
#671=ORIENTED_EDGE ( 'NONE', *, *, #1084, .F. ) ;
#677=CARTESIAN_POINT ( 'NONE',  ( 0.000000000000000000, 0.000000000000000000, -25.50000000000000355 ) ) ;
#678=CARTESIAN_POINT ( 'NONE',  ( 0.000000000000000000, 0.000000000000000000, -10.50000000000000000 ) ) ;
#680=DIRECTION ( 'NONE',  ( -1.000000000000000000, 2.312964634635740689E-15, 0.000000000000000000 ) ) ;
#682=ORIENTED_EDGE ( 'NONE', *, *, #13960, .F. ) ;
#683=ORIENTED_EDGE ( 'NONE', *, *, #7014, .T. ) ;
#689=DIRECTION ( 'NONE',  ( -0.000000000000000000, -0.000000000000000000, 1.000000000000000000 ) ) ;
#690=DIRECTION ( 'NONE',  ( 1.000000000000000000, 0.000000000000000000, 0.000000000000000000 ) ) ;
#691=CARTESIAN_POINT ( 'NONE',  ( 97.41488903138106537, -0.2790467552935826934, 10.49999999999999822 ) ) ;
#695=DIRECTION ( 'NONE',  ( 0.000000000000000000, 0.000000000000000000, 1.000000000000000000 ) ) ;
#696=CARTESIAN_POINT ( 'NONE',  ( -13.71740939043329277, 51.19406879332069593, -13.00000000000000178 ) ) ;
#700=EDGE_CURVE ( 'NONE', #197, #2566, #14081, .T. ) ;
#702=ORIENTED_EDGE ( 'NONE', *, *, #1068, .F. ) ;
#703=DIRECTION ( 'NONE',  ( 0.000000000000000000, 0.000000000000000000, 1.000000000000000000 ) ) ;
#704=ORIENTED_EDGE ( 'NONE', *, *, #2823, .T. ) ;
#706=CARTESIAN_POINT ( 'NONE',  ( -68.08935777509570642, -68.58935777509452691, 10.49999999999999822 ) ) ;
#707=DIRECTION ( 'NONE',  ( 1.000000000000000000, 0.000000000000000000, -0.000000000000000000 ) ) ;
#708=CARTESIAN_POINT ( 'NONE',  ( 97.00000000000000000, -3.384287605079545030E-13, -13.00000000000000178 ) ) ;
#709=CARTESIAN_POINT ( 'NONE',  ( -56.43380494354004639, -12.86891638962099549, -10.50000000000000000 ) ) ;
#710=VECTOR ( 'NONE', #9042, 1000.000000000000000 ) ;
#711=CARTESIAN_POINT ( 'NONE',  ( 45.96504489226007450, -23.50071946824056823, 8.000000000000000000 ) ) ;
#712=ORIENTED_EDGE ( 'NONE', *, *, #2162, .T. ) ;
#713=DIRECTION ( 'NONE',  ( -1.000000000000000000, 0.000000000000000000, 0.000000000000000000 ) ) ;
#716=ORIENTED_EDGE ( 'NONE', *, *, #2095, .T. ) ;
#718=ADVANCED_FACE ( 'NONE', ( #2614 ), #6307, .T. ) ;
#719=VECTOR ( 'NONE', #151, 1000.000000000000000 ) ;
#723=DIRECTION ( 'NONE',  ( 0.000000000000000000, 0.000000000000000000, 1.000000000000000000 ) ) ;
#724=ADVANCED_FACE ( 'NONE', ( #7388 ), #9813, .F. ) ;
#726=CARTESIAN_POINT ( 'NONE',  ( 34.62083247296202160, 87.95718916809205723, 8.000000000000000000 ) ) ;
#728=ORIENTED_EDGE ( 'NONE', *, *, #11280, .F. ) ;
#731=EDGE_LOOP ( 'NONE', ( #3868, #9736, #5381, #217, #12088 ) ) ;
#732=VECTOR ( 'NONE', #5789, 1000.000000000000000 ) ;
#733=EDGE_CURVE ( 'NONE', #11315, #4753, #8530, .T. ) ;
#734=CARTESIAN_POINT ( 'NONE',  ( -96.58511096861892042, -0.2790467552922097916, -13.00000000000000178 ) ) ;
#735=AXIS2_PLACEMENT_3D ( 'NONE', #8739, #10180, #785 ) ;
#737=CIRCLE ( 'NONE', #7019, 3.000000000000002665 ) ;
#738=DIRECTION ( 'NONE',  ( 1.000000000000000000, 0.000000000000000000, 0.000000000000000000 ) ) ;
#740=ORIENTED_EDGE ( 'NONE', *, *, #5593, .F. ) ;
#741=ADVANCED_FACE ( 'NONE', ( #14379 ), #10736, .F. ) ;
#742=ORIENTED_EDGE ( 'NONE', *, *, #5549, .F. ) ;
#743=AXIS2_PLACEMENT_3D ( 'NONE', #8201, #3353, #9406 ) ;
#744=EDGE_CURVE ( 'NONE', #1887, #14718, #1554, .T. ) ;
#745=AXIS2_PLACEMENT_3D ( 'NONE', #14612, #4209, #7608 ) ;
#747=VECTOR ( 'NONE', #10628, 1000.000000000000000 ) ;
#748=AXIS2_PLACEMENT_3D ( 'NONE', #65, #12824, #6815 ) ;
#749=DIRECTION ( 'NONE',  ( 0.000000000000000000, 0.000000000000000000, 1.000000000000000000 ) ) ;
#751=CARTESIAN_POINT ( 'NONE',  ( 42.04772703543530099, 32.26435573746242369, -10.50000000000000000 ) ) ;
#752=ORIENTED_EDGE ( 'NONE', *, *, #5151, .T. ) ;
#753=CARTESIAN_POINT ( 'NONE',  ( 50.00000000000000000, -6.123233995736766085E-15, -13.00000000000000178 ) ) ;
#757=FACE_OUTER_BOUND ( 'NONE', #7860, .T. ) ;
#758=AXIS2_PLACEMENT_3D ( 'NONE', #11388, #9323, #6891 ) ;
#760=AXIS2_PLACEMENT_3D ( 'NONE', #9897, #8613, #7466 ) ;
#763=DIRECTION ( 'NONE',  ( 0.000000000000000000, 0.000000000000000000, -1.000000000000000000 ) ) ;
#764=AXIS2_PLACEMENT_3D ( 'NONE', #3724, #299, #9545 ) ;
#765=UNCERTAINTY_MEASURE_WITH_UNIT (LENGTH_MEASURE( 1.000000000000000082E-05 ), #9684, 'distance_accuracy_value', 'NONE');
#766=CARTESIAN_POINT ( 'NONE',  ( 26.01305530232562546, 46.81487971942612347, -10.50000000000000000 ) ) ;
#767=LINE ( 'NONE', #13582, #7256 ) ;
#768=CIRCLE ( 'NONE', #6284, 56.99999999999999289 ) ;
#769=CARTESIAN_POINT ( 'NONE',  ( 12.86891638962116247, -56.43380494354001087, 10.49999999999999822 ) ) ;
#770=AXIS2_PLACEMENT_3D ( 'NONE', #14698, #10278, #9977 ) ;
#773=DIRECTION ( 'NONE',  ( 0.000000000000000000, 0.000000000000000000, 1.000000000000000000 ) ) ;
#774=PLANE ( 'NONE',  #6790 ) ;
#775=AXIS2_PLACEMENT_3D ( 'NONE', #14759, #8899, #5996 ) ;
#780=ORIENTED_EDGE ( 'NONE', *, *, #9429, .T. ) ;
#781=DIRECTION ( 'NONE',  ( 0.000000000000000000, 0.000000000000000000, 1.000000000000000000 ) ) ;
#782=EDGE_LOOP ( 'NONE', ( #5644, #459, #8549, #7892 ) ) ;
#784=CARTESIAN_POINT ( 'NONE',  ( 0.000000000000000000, 0.000000000000000000, -8.000000000000000000 ) ) ;
#785=DIRECTION ( 'NONE',  ( 1.000000000000000000, 0.000000000000000000, 0.000000000000000000 ) ) ;
#787=CIRCLE ( 'NONE', #2439, 53.55662432702593634 ) ;
#788=CYLINDRICAL_SURFACE ( 'NONE', #4138, 0.5000000000000038858 ) ;
#789=ADVANCED_FACE ( 'NONE', ( #417 ), #5271, .F. ) ;
#790=DIRECTION ( 'NONE',  ( 1.000000000000000000, 0.000000000000000000, 0.000000000000000000 ) ) ;
#791=ADVANCED_FACE ( 'NONE', ( #3767 ), #10878, .F. ) ;
#793=ORIENTED_EDGE ( 'NONE', *, *, #6481, .F. ) ;
#794=DIRECTION ( 'NONE',  ( 1.000000000000000000, 0.000000000000000000, 0.000000000000000000 ) ) ;
#795=ORIENTED_EDGE ( 'NONE', *, *, #10804, .F. ) ;
#797=DIRECTION ( 'NONE',  ( 0.000000000000000000, 0.000000000000000000, 1.000000000000000000 ) ) ;
#799=DIRECTION ( 'NONE',  ( 0.000000000000000000, 0.000000000000000000, 1.000000000000000000 ) ) ;
#800=EDGE_CURVE ( 'NONE', #13568, #2920, #2306, .T. ) ;
#802=ORIENTED_EDGE ( 'NONE', *, *, #11867, .T. ) ;
#805=CIRCLE ( 'NONE', #4679, 0.5000000000000004441 ) ;
#807=CARTESIAN_POINT ( 'NONE',  ( -42.04772703543551415, -32.26435573746212526, -13.00000000000000178 ) ) ;
#808=LINE ( 'NONE', #12276, #11652 ) ;
#809=CARTESIAN_POINT ( 'NONE',  ( 12.86891638962116247, -56.43380494354001087, -10.50000000000000000 ) ) ;
#813=AXIS2_PLACEMENT_3D ( 'NONE', #14533, #3362, #9132 ) ;
#814=DIRECTION ( 'NONE',  ( 0.000000000000000000, 0.000000000000000000, 1.000000000000000000 ) ) ;
#816=AXIS2_PLACEMENT_3D ( 'NONE', #13154, #13008, #2599 ) ;
#817=EDGE_CURVE ( 'NONE', #5666, #5951, #861, .T. ) ;
#823=CIRCLE ( 'NONE', #9290, 3.000000000000002665 ) ;
#824=PLANE ( 'NONE',  #113 ) ;
#825=CARTESIAN_POINT ( 'NONE',  ( 4.121772567811984089, 51.45950017607689375, -13.00000000000000178 ) ) ;
#826=FACE_OUTER_BOUND ( 'NONE', #6542, .T. ) ;
#828=AXIS2_PLACEMENT_3D ( 'NONE', #12344, #8988, #11286 ) ;
#829=EDGE_LOOP ( 'NONE', ( #9264, #5861, #13271, #12662, #11486, #14467, #7990, #3983, #7476 ) ) ;
#830=FACE_OUTER_BOUND ( 'NONE', #1962, .T. ) ;
#832=ORIENTED_EDGE ( 'NONE', *, *, #7672, .F. ) ;
#834=ADVANCED_FACE ( 'NONE', ( #2693 ), #3913, .F. ) ;
#836=VERTEX_POINT ( 'NONE', #1698 ) ;
#837=EDGE_LOOP ( 'NONE', ( #2974, #13482 ) ) ;
#838=AXIS2_PLACEMENT_3D ( 'NONE', #6617, #7914, #11421 ) ;
#839=DIRECTION ( 'NONE',  ( 1.000000000000000000, 0.000000000000000000, 0.000000000000000000 ) ) ;
#840=CIRCLE ( 'NONE', #5187, 59.49999999999999289 ) ;
#841=CIRCLE ( 'NONE', #3261, 3.000000000000002665 ) ;
#843=FACE_OUTER_BOUND ( 'NONE', #79, .T. ) ;
#848=ORIENTED_EDGE ( 'NONE', *, *, #180, .T. ) ;
#849=VECTOR ( 'NONE', #15018, 1000.000000000000000 ) ;
#850=AXIS2_PLACEMENT_3D ( 'NONE', #12106, #9589, #11046 ) ;
#851=CARTESIAN_POINT ( 'NONE',  ( 0.000000000000000000, 0.000000000000000000, -10.50000000000000000 ) ) ;
#852=CIRCLE ( 'NONE', #12476, 52.50000000000000711 ) ;
#853=EDGE_CURVE ( 'NONE', #13570, #6495, #9094, .T. ) ;
#855=FACE_OUTER_BOUND ( 'NONE', #10621, .T. ) ;
#856=EDGE_LOOP ( 'NONE', ( #12786, #6236, #14465, #13367, #7872, #10379 ) ) ;
#860=ORIENTED_EDGE ( 'NONE', *, *, #12331, .T. ) ;
#861=CIRCLE ( 'NONE', #14198, 0.5000000000000004441 ) ;
#862=CYLINDRICAL_SURFACE ( 'NONE', #12376, 3.000000000000002665 ) ;
#864=ORIENTED_EDGE ( 'NONE', *, *, #408, .F. ) ;
#866=LINE ( 'NONE', #6604, #1467 ) ;
#867=FACE_OUTER_BOUND ( 'NONE', #2559, .T. ) ;
#869=FACE_OUTER_BOUND ( 'NONE', #12218, .T. ) ;
#870=DIRECTION ( 'NONE',  ( -0.000000000000000000, -0.000000000000000000, 1.000000000000000000 ) ) ;
#871=CARTESIAN_POINT ( 'NONE',  ( 68.58935777509523746, 68.58935777509499587, 8.000000000000000000 ) ) ;
#872=AXIS2_PLACEMENT_3D ( 'NONE', #6826, #11629, #4643 ) ;
#873=ORIENTED_EDGE ( 'NONE', *, *, #14833, .F. ) ;
#874=DIRECTION ( 'NONE',  ( 1.000000000000000000, 0.000000000000000000, 0.000000000000000000 ) ) ;
#875=CARTESIAN_POINT ( 'NONE',  ( 36.14014761921570340, 11.74264578624841171, -28.00000000000000000 ) ) ;
#877=VERTEX_POINT ( 'NONE', #6466 ) ;
#880=EDGE_CURVE ( 'NONE', #198, #2094, #14679, .T. ) ;
#883=EDGE_CURVE ( 'NONE', #12576, #13345, #3048, .T. ) ;
#884=ORIENTED_EDGE ( 'NONE', *, *, #9126, .F. ) ;
#886=PLANE ( 'NONE',  #14118 ) ;
#887=ORIENTED_EDGE ( 'NONE', *, *, #9762, .F. ) ;
#890=SHAPE_DEFINITION_REPRESENTATION ( #8756, #8100 ) ;
#891=ORIENTED_EDGE ( 'NONE', *, *, #5512, .T. ) ;
#892=EDGE_CURVE ( 'NONE', #6431, #4070, #4988, .T. ) ;
#893=ORIENTED_EDGE ( 'NONE', *, *, #1747, .T. ) ;
#894=ORIENTED_EDGE ( 'NONE', *, *, #507, .T. ) ;
#895=AXIS2_PLACEMENT_3D ( 'NONE', #10587, #2460, #13023 ) ;
#898=PRODUCT_DEFINITION ( 'UNKNOWN', '', #7251, #8798 ) ;
#899=FACE_OUTER_BOUND ( 'NONE', #14602, .T. ) ;
#900=VERTEX_POINT ( 'NONE', #11345 ) ;
#901=ORIENTED_EDGE ( 'NONE', *, *, #9138, .F. ) ;
#903=ORIENTED_EDGE ( 'NONE', *, *, #8788, .T. ) ;
#904=AXIS2_PLACEMENT_3D ( 'NONE', #239, #2746, #2670 ) ;
#906=DIRECTION ( 'NONE',  ( -0.000000000000000000, -0.000000000000000000, -1.000000000000000000 ) ) ;
#907=FACE_OUTER_BOUND ( 'NONE', #14733, .T. ) ;
#909=PLANE ( 'NONE',  #14468 ) ;
#913=DIRECTION ( 'NONE',  ( 0.000000000000000000, 0.000000000000000000, 1.000000000000000000 ) ) ;
#914=VERTEX_POINT ( 'NONE', #6759 ) ;
#915=VERTEX_POINT ( 'NONE', #9970 ) ;
#916=CARTESIAN_POINT ( 'NONE',  ( 68.58935777509523746, 68.58935777509499587, 8.000000000000000000 ) ) ;
#917=CARTESIAN_POINT ( 'NONE',  ( 92.38795325112879198, 38.26834323650871994, -8.000000000000000000 ) ) ;
#918=EDGE_CURVE ( 'NONE', #11991, #13011, #1582, .T. ) ;
#920=ADVANCED_FACE ( 'NONE', ( #5564 ), #14693, .F. ) ;
#922=DIRECTION ( 'NONE',  ( 0.000000000000000000, 0.000000000000000000, 1.000000000000000000 ) ) ;
#924=DIRECTION ( 'NONE',  ( -1.000000000000000000, 4.440892098500625373E-15, 0.000000000000000000 ) ) ;
#925=ORIENTED_EDGE ( 'NONE', *, *, #1390, .T. ) ;
#926=FACE_OUTER_BOUND ( 'NONE', #7857, .T. ) ;
#927=EDGE_CURVE ( 'NONE', #10678, #6180, #11510, .T. ) ;
#928=FACE_OUTER_BOUND ( 'NONE', #13623, .T. ) ;
#930=ORIENTED_EDGE ( 'NONE', *, *, #9961, .F. ) ;
#931=CYLINDRICAL_SURFACE ( 'NONE', #8853, 60.50000000000000000 ) ;
#932=ORIENTED_EDGE ( 'NONE', *, *, #14579, .T. ) ;
#934=VECTOR ( 'NONE', #3788, 1000.000000000000000 ) ;
#935=ORIENTED_EDGE ( 'NONE', *, *, #10386, .T. ) ;
#936=DIRECTION ( 'NONE',  ( 1.000000000000000000, 0.000000000000000000, -0.000000000000000000 ) ) ;
#937=EDGE_CURVE ( 'NONE', #3633, #12431, #11256, .T. ) ;
#938=DIRECTION ( 'NONE',  ( 0.000000000000000000, 0.000000000000000000, -1.000000000000000000 ) ) ;
#939=CARTESIAN_POINT ( 'NONE',  ( -41.59008834022669987, -32.46576781417940794, 10.49999999999999822 ) ) ;
#940=DIRECTION ( 'NONE',  ( 1.000000000000000000, 0.000000000000000000, 0.000000000000000000 ) ) ;
#941=DIRECTION ( 'NONE',  ( 0.000000000000000000, 0.000000000000000000, 1.000000000000000000 ) ) ;
#946=DIRECTION ( 'NONE',  ( 0.000000000000000000, 0.000000000000000000, 1.000000000000000000 ) ) ;
#947=CARTESIAN_POINT ( 'NONE',  ( 26.49999999999971578, 45.89934640057541060, -13.00000000000000178 ) ) ;
#948=AXIS2_PLACEMENT_3D ( 'NONE', #8124, #11226, #14645 ) ;
#949=ORIENTED_EDGE ( 'NONE', *, *, #12444, .T. ) ;
#951=ORIENTED_EDGE ( 'NONE', *, *, #10472, .F. ) ;
#953=ORIENTED_EDGE ( 'NONE', *, *, #11366, .F. ) ;
#954=DIRECTION ( 'NONE',  ( -1.000000000000000000, 0.000000000000000000, 0.000000000000000000 ) ) ;
#955=DIRECTION ( 'NONE',  ( 0.000000000000000000, 0.000000000000000000, -1.000000000000000000 ) ) ;
#956=CARTESIAN_POINT ( 'NONE',  ( -34.62083247296263266, -87.95718916809180143, -13.00000000000000178 ) ) ;
#957=LINE ( 'NONE', #5726, #4707 ) ;
#958=ORIENTED_EDGE ( 'NONE', *, *, #4574, .T. ) ;
#959=ORIENTED_EDGE ( 'NONE', *, *, #424, .T. ) ;
#961=DIRECTION ( 'NONE',  ( 0.000000000000000000, 0.000000000000000000, 1.000000000000000000 ) ) ;
#964=VERTEX_POINT ( 'NONE', #10043 ) ;
#965=CIRCLE ( 'NONE', #13557, 3.000000000000002665 ) ;
#966=ORIENTED_EDGE ( 'NONE', *, *, #7536, .T. ) ;
#967=VERTEX_POINT ( 'NONE', #5423 ) ;
#968=CARTESIAN_POINT ( 'NONE',  ( -47.21331623427138879, -33.48561063518577896, -8.000000000000000000 ) ) ;
#969=DIRECTION ( 'NONE',  ( 1.000000000000000000, 1.687538997430237941E-13, 0.000000000000000000 ) ) ;
#974=CYLINDRICAL_SURFACE ( 'NONE', #6077, 56.99999999999999289 ) ;
#976=ADVANCED_FACE ( 'NONE', ( #14532 ), #10189, .F. ) ;
#977=AXIS2_PLACEMENT_3D ( 'NONE', #8876, #11243, #3047 ) ;
#980=DIRECTION ( 'NONE',  ( 1.000000000000000000, 0.000000000000000000, 0.000000000000000000 ) ) ;
#981=DIRECTION ( 'NONE',  ( 0.000000000000000000, 0.000000000000000000, 1.000000000000000000 ) ) ;
#982=EDGE_LOOP ( 'NONE', ( #3565, #4421, #12085, #3961, #2352 ) ) ;
#983=AXIS2_PLACEMENT_3D ( 'NONE', #5104, #3827, #13300 ) ;
#984=ORIENTED_EDGE ( 'NONE', *, *, #8096, .T. ) ;
#985=DIRECTION ( 'NONE',  ( 0.000000000000000000, 0.000000000000000000, 1.000000000000000000 ) ) ;
#987=AXIS2_PLACEMENT_3D ( 'NONE', #4430, #6526, #9040 ) ;
#989=ORIENTED_EDGE ( 'NONE', *, *, #651, .T. ) ;
#990=DIRECTION ( 'NONE',  ( -0.000000000000000000, -0.000000000000000000, 1.000000000000000000 ) ) ;
#991=DIRECTION ( 'NONE',  ( 0.000000000000000000, 0.000000000000000000, 1.000000000000000000 ) ) ;
#992=DIRECTION ( 'NONE',  ( 1.000000000000000000, 0.000000000000000000, -0.000000000000000000 ) ) ;
#996=ORIENTED_EDGE ( 'NONE', *, *, #8709, .F. ) ;
#997=DIRECTION ( 'NONE',  ( 0.000000000000000000, 0.000000000000000000, 1.000000000000000000 ) ) ;
#998=CIRCLE ( 'NONE', #11917, 60.49999999999999289 ) ;
#999=CARTESIAN_POINT ( 'NONE',  ( -12.94095225512575809, 48.29629131445349088, -8.000000000000000000 ) ) ;
#1000=DIRECTION ( 'NONE',  ( -1.000000000000000000, 0.000000000000000000, 0.000000000000000000 ) ) ;
#1001=EDGE_CURVE ( 'NONE', #10819, #13762, #13999, .T. ) ;
#1002=ORIENTED_EDGE ( 'NONE', *, *, #1299, .F. ) ;
#1003=FACE_OUTER_BOUND ( 'NONE', #11210, .T. ) ;
#1004=AXIS2_PLACEMENT_3D ( 'NONE', #11704, #10399, #6901 ) ;
#1005=ORIENTED_EDGE ( 'NONE', *, *, #546, .T. ) ;
#1006=AXIS2_PLACEMENT_3D ( 'NONE', #3634, #3567, #8184 ) ;
#1007=DIRECTION ( 'NONE',  ( 1.000000000000000000, 0.000000000000000000, 0.000000000000000000 ) ) ;
#1008=EDGE_CURVE ( 'NONE', #12422, #9491, #11751, .T. ) ;
#1009=LINE ( 'NONE', #6455, #5344 ) ;
#1010=CIRCLE ( 'NONE', #5121, 3.000000000000002665 ) ;
#1012=CARTESIAN_POINT ( 'NONE',  ( -33.48561063518626923, 47.21331623427104063, -10.50000000000000000 ) ) ;
#1013=CARTESIAN_POINT ( 'NONE',  ( -48.29629131445345536, -12.94095225512591618, -8.000000000000000000 ) ) ;
#1014=CARTESIAN_POINT ( 'NONE',  ( -68.58935777509427112, 68.58935777509594800, -10.50000000000000000 ) ) ;
#1016=DIRECTION ( 'NONE',  ( 1.000000000000000000, 0.000000000000000000, 0.000000000000000000 ) ) ;
#1017=AXIS2_PLACEMENT_3D ( 'NONE', #9379, #8526, #13310 ) ;
#1018=ORIENTED_EDGE ( 'NONE', *, *, #9654, .T. ) ;
#1019=DIRECTION ( 'NONE',  ( 0.000000000000000000, 0.000000000000000000, 1.000000000000000000 ) ) ;
#1020=DIRECTION ( 'NONE',  ( -0.000000000000000000, -0.000000000000000000, -1.000000000000000000 ) ) ;
#1024=DIRECTION ( 'NONE',  ( 1.000000000000000000, 0.000000000000000000, 0.000000000000000000 ) ) ;
#1028=ORIENTED_EDGE ( 'NONE', *, *, #2126, .T. ) ;
#1029=DIRECTION ( 'NONE',  ( -1.000000000000000000, 0.000000000000000000, 0.000000000000000000 ) ) ;
#1031=CIRCLE ( 'NONE', #2237, 56.99999999999999289 ) ;
#1032=DIRECTION ( 'NONE',  ( 1.000000000000000000, 0.000000000000000000, 0.000000000000000000 ) ) ;
#1034=EDGE_CURVE ( 'NONE', #511, #2333, #1078, .T. ) ;
#1036=AXIS2_PLACEMENT_3D ( 'NONE', #8185, #4073, #7031 ) ;
#1037=CARTESIAN_POINT ( 'NONE',  ( -36.62029293941440500, -89.61631465359452875, 10.49999999999999822 ) ) ;
#1038=ORIENTED_EDGE ( 'NONE', *, *, #14260, .F. ) ;
#1043=DIRECTION ( 'NONE',  ( 1.000000000000000000, 0.000000000000000000, 0.000000000000000000 ) ) ;
#1044=DIRECTION ( 'NONE',  ( 1.000000000000000000, 0.000000000000000000, 0.000000000000000000 ) ) ;
#1045=ORIENTED_EDGE ( 'NONE', *, *, #3414, .F. ) ;
#1046=AXIS2_PLACEMENT_3D ( 'NONE', #3307, #13941, #11731 ) ;
#1047=ORIENTED_EDGE ( 'NONE', *, *, #10839, .F. ) ;
#1048=ORIENTED_EDGE ( 'NONE', *, *, #4644, .F. ) ;
#1050=ADVANCED_FACE ( 'NONE', ( #5639 ), #8067, .T. ) ;
#1051=VECTOR ( 'NONE', #10496, 1000.000000000000000 ) ;
#1054=DIRECTION ( 'NONE',  ( 1.000000000000000000, 0.000000000000000000, 0.000000000000000000 ) ) ;
#1055=VERTEX_POINT ( 'NONE', #12627 ) ;
#1056=CARTESIAN_POINT ( 'NONE',  ( -37.02125851216292318, 90.10640870805768543, 10.49999999999999822 ) ) ;
#1059=CARTESIAN_POINT ( 'NONE',  ( 31.05588327715837238, -44.79355920668822222, -8.000000000000000000 ) ) ;
#1060=DIRECTION ( 'NONE',  ( 1.000000000000000000, 0.000000000000000000, 0.000000000000000000 ) ) ;
#1061=CIRCLE ( 'NONE', #7341, 0.5000000000000004441 ) ;
#1062=ORIENTED_EDGE ( 'NONE', *, *, #5722, .T. ) ;
#1063=VECTOR ( 'NONE', #7099, 1000.000000000000000 ) ;
#1064=ORIENTED_EDGE ( 'NONE', *, *, #4462, .F. ) ;
#1066=EDGE_CURVE ( 'NONE', #6492, #1186, #13431, .T. ) ;
#1067=EDGE_CURVE ( 'NONE', #4053, #6451, #6872, .T. ) ;
#1068=EDGE_CURVE ( 'NONE', #3184, #14306, #10255, .T. ) ;
#1069=CARTESIAN_POINT ( 'NONE',  ( -56.43380494354004639, -12.86891638962099549, -13.00000000000000178 ) ) ;
#1070=DIRECTION ( 'NONE',  ( 0.000000000000000000, 0.000000000000000000, 1.000000000000000000 ) ) ;
#1071=CIRCLE ( 'NONE', #9763, 63.00000000000000000 ) ;
#1072=DIRECTION ( 'NONE',  ( 1.000000000000000000, 0.000000000000000000, -0.000000000000000000 ) ) ;
#1073=DIRECTION ( 'NONE',  ( 0.000000000000000000, 0.000000000000000000, 1.000000000000000000 ) ) ;
#1076=VERTEX_POINT ( 'NONE', #6921 ) ;
#1077=LINE ( 'NONE', #9109, #4160 ) ;
#1078=CIRCLE ( 'NONE', #590, 0.5000000000000073275 ) ;
#1080=CARTESIAN_POINT ( 'NONE',  ( 1.836970198721029747E-14, -100.0000000000000000, 8.000000000000000000 ) ) ;
#1082=AXIS2_PLACEMENT_3D ( 'NONE', #12825, #7037, #8342 ) ;
#1083=ORIENTED_EDGE ( 'NONE', *, *, #12114, .T. ) ;
#1084=EDGE_CURVE ( 'NONE', #7921, #9052, #5933, .T. ) ;
#1085=DIRECTION ( 'NONE',  ( 1.000000000000000000, 0.000000000000000000, 0.000000000000000000 ) ) ;
#1088=EDGE_CURVE ( 'NONE', #2988, #1331, #9981, .T. ) ;
#1089=CARTESIAN_POINT ( 'NONE',  ( -6.451868917687557214, -52.36539807335606156, -13.00000000000000178 ) ) ;
#1090=DIRECTION ( 'NONE',  ( 0.000000000000000000, 0.000000000000000000, 1.000000000000000000 ) ) ;
#1093=CIRCLE ( 'NONE', #14668, 3.000000000000002665 ) ;
#1094=VECTOR ( 'NONE', #12798, 1000.000000000000000 ) ;
#1095=CIRCLE ( 'NONE', #12238, 3.000000000000002665 ) ;
#1097=CARTESIAN_POINT ( 'NONE',  ( 69.08004447556065486, 68.68541276968852571, 10.49999999999999822 ) ) ;
#1098=ORIENTED_EDGE ( 'NONE', *, *, #13042, .T. ) ;
#1100=CARTESIAN_POINT ( 'NONE',  ( -42.04772703543551415, -32.26435573746212526, 10.49999999999999822 ) ) ;
#1101=DIRECTION ( 'NONE',  ( 0.000000000000000000, 0.000000000000000000, -1.000000000000000000 ) ) ;
#1102=AXIS2_PLACEMENT_3D ( 'NONE', #1355, #1573, #7176 ) ;
#1103=VECTOR ( 'NONE', #3208, 1000.000000000000000 ) ;
#1104=DIRECTION ( 'NONE',  ( -1.000000000000000000, 0.000000000000000000, 0.000000000000000000 ) ) ;
#1105=ORIENTED_EDGE ( 'NONE', *, *, #8346, .F. ) ;
#1106=CARTESIAN_POINT ( 'NONE',  ( 12.86891638962116247, -56.43380494354001087, 10.49999999999999822 ) ) ;
#1107=VERTEX_POINT ( 'NONE', #11720 ) ;
#1108=DIRECTION ( 'NONE',  ( 0.000000000000000000, 0.000000000000000000, 1.000000000000000000 ) ) ;
#1109=CARTESIAN_POINT ( 'NONE',  ( 26.99988008862626643, 45.88839665196127271, -10.50000000000000000 ) ) ;
#1110=EDGE_CURVE ( 'NONE', #4909, #8032, #8144, .T. ) ;
#1113=EDGE_CURVE ( 'NONE', #10850, #5953, #3446, .T. ) ;
#1114=DIRECTION ( 'NONE',  ( -0.000000000000000000, -0.000000000000000000, 1.000000000000000000 ) ) ;
#1115=VERTEX_POINT ( 'NONE', #10494 ) ;
#1116=AXIS2_PLACEMENT_3D ( 'NONE', #9933, #12534, #1823 ) ;
#1119=ORIENTED_EDGE ( 'NONE', *, *, #10981, .F. ) ;
#1120=DIRECTION ( 'NONE',  ( -1.000000000000000000, 0.000000000000000000, 0.000000000000000000 ) ) ;
#1121=DIRECTION ( 'NONE',  ( 0.000000000000000000, 0.000000000000000000, 1.000000000000000000 ) ) ;
#1123=CIRCLE ( 'NONE', #2560, 0.5000000000000043299 ) ;
#1124=VERTEX_POINT ( 'NONE', #14065 ) ;
#1126=AXIS2_PLACEMENT_3D ( 'NONE', #7045, #5916, #10624 ) ;
#1127=EDGE_LOOP ( 'NONE', ( #6521, #13064, #2206, #269, #930 ) ) ;
#1130=CARTESIAN_POINT ( 'NONE',  ( 52.50000000000000711, -6.429395695523604744E-15, -10.50000000000000000 ) ) ;
#1131=EDGE_CURVE ( 'NONE', #11551, #469, #6076, .T. ) ;
#1132=DIRECTION ( 'NONE',  ( -1.000000000000000000, 0.000000000000000000, 0.000000000000000000 ) ) ;
#1134=CARTESIAN_POINT ( 'NONE',  ( 89.89283556784508278, -37.53686968382275779, 10.49999999999999822 ) ) ;
#1135=ORIENTED_EDGE ( 'NONE', *, *, #927, .F. ) ;
#1136=DIRECTION ( 'NONE',  ( 1.000000000000000000, 0.000000000000000000, -0.000000000000000000 ) ) ;
#1138=ORIENTED_EDGE ( 'NONE', *, *, #13360, .F. ) ;
#1139=DIRECTION ( 'NONE',  ( -1.000000000000000000, 0.000000000000000000, 0.000000000000000000 ) ) ;
#1141=ORIENTED_EDGE ( 'NONE', *, *, #1629, .T. ) ;
#1143=CARTESIAN_POINT ( 'NONE',  ( -52.36539807335606156, 6.451868917687758831, -13.00000000000000178 ) ) ;
#1144=VERTEX_POINT ( 'NONE', #10863 ) ;
#1145=CARTESIAN_POINT ( 'NONE',  ( -38.79014761921587962, 11.74264578624790190, -25.50000000000000355 ) ) ;
#1146=DIRECTION ( 'NONE',  ( 1.000000000000000000, 0.000000000000000000, 0.000000000000000000 ) ) ;
#1148=CARTESIAN_POINT ( 'NONE',  ( 37.53686968382241673, 89.89283556784525331, 10.49999999999999822 ) ) ;
#1149=ORIENTED_EDGE ( 'NONE', *, *, #602, .F. ) ;
#1150=DIRECTION ( 'NONE',  ( 0.000000000000000000, 0.000000000000000000, -1.000000000000000000 ) ) ;
#1151=ORIENTED_EDGE ( 'NONE', *, *, #5739, .F. ) ;
#1152=ADVANCED_FACE ( 'NONE', ( #1615 ), #7441, .F. ) ;
#1153=DIRECTION ( 'NONE',  ( -0.000000000000000000, -0.000000000000000000, 1.000000000000000000 ) ) ;
#1154=EDGE_CURVE ( 'NONE', #3918, #406, #14383, .T. ) ;
#1155=VERTEX_POINT ( 'NONE', #13077 ) ;
#1156=DIRECTION ( 'NONE',  ( 1.000000000000000000, 9.329605248950895679E-16, 0.000000000000000000 ) ) ;
#1157=FACE_OUTER_BOUND ( 'NONE', #14377, .T. ) ;
#1161=DIRECTION ( 'NONE',  ( -1.000000000000000000, 0.000000000000000000, 0.000000000000000000 ) ) ;
#1163=CARTESIAN_POINT ( 'NONE',  ( 49.00442420935993226, -30.80502811811213704, -13.00000000000000178 ) ) ;
#1164=EDGE_CURVE ( 'NONE', #13227, #8073, #318, .T. ) ;
#1165=DIRECTION ( 'NONE',  ( 0.000000000000000000, 0.000000000000000000, -1.000000000000000000 ) ) ;
#1167=EDGE_CURVE ( 'NONE', #11760, #6451, #6288, .T. ) ;
#1170=DIRECTION ( 'NONE',  ( 1.000000000000000000, 0.000000000000000000, 0.000000000000000000 ) ) ;
#1171=PLANE ( 'NONE',  #14865 ) ;
#1173=ORIENTED_EDGE ( 'NONE', *, *, #11745, .T. ) ;
#1175=EDGE_LOOP ( 'NONE', ( #12279, #493, #10132, #8231 ) ) ;
#1178=CARTESIAN_POINT ( 'NONE',  ( 0.2790467552932288098, 97.41488903138106537, -10.50000000000000000 ) ) ;
#1179=CARTESIAN_POINT ( 'NONE',  ( 30.80502811811196295, 49.00442420936003174, 10.49999999999999822 ) ) ;
#1180=ORIENTED_EDGE ( 'NONE', *, *, #14238, .T. ) ;
#1183=FACE_OUTER_BOUND ( 'NONE', #2396, .T. ) ;
#1186=VERTEX_POINT ( 'NONE', #6155 ) ;
#1187=ORIENTED_EDGE ( 'NONE', *, *, #10479, .T. ) ;
#1188=EDGE_CURVE ( 'NONE', #132, #5666, #11485, .T. ) ;
#1189=DIRECTION ( 'NONE',  ( -1.000000000000000000, 0.000000000000000000, 0.000000000000000000 ) ) ;
#1193=ADVANCED_FACE ( 'NONE', ( #8656 ), #240, .F. ) ;
#1194=DIRECTION ( 'NONE',  ( -1.000000000000000000, 0.000000000000000000, 0.000000000000000000 ) ) ;
#1195=EDGE_LOOP ( 'NONE', ( #10370, #3333, #13617, #10087, #10514, #11394 ) ) ;
#1198=CARTESIAN_POINT ( 'NONE',  ( 1.674280531759317014, -94.51066581171355097, 8.000000000000000000 ) ) ;
#1200=DIRECTION ( 'NONE',  ( 0.000000000000000000, 0.000000000000000000, 1.000000000000000000 ) ) ;
#1201=ORIENTED_EDGE ( 'NONE', *, *, #6664, .F. ) ;
#1205=DIRECTION ( 'NONE',  ( 0.000000000000000000, 0.000000000000000000, 1.000000000000000000 ) ) ;
#1206=ORIENTED_EDGE ( 'NONE', *, *, #2111, .T. ) ;
#1207=VERTEX_POINT ( 'NONE', #8367 ) ;
#1210=CARTESIAN_POINT ( 'NONE',  ( -10.71740939043329099, 51.19406879332069593, -13.00000000000000178 ) ) ;
#1211=DIRECTION ( 'NONE',  ( -0.000000000000000000, -0.000000000000000000, 1.000000000000000000 ) ) ;
#1213=CARTESIAN_POINT ( 'NONE',  ( 0.5000000000000045519, -97.00000000000000000, -10.50000000000000000 ) ) ;
#1214=EDGE_LOOP ( 'NONE', ( #2822, #10967, #11441, #6951, #1083, #5063, #11913, #14182, #10277, #10821 ) ) ;
#1215=LINE ( 'NONE', #5836, #7523 ) ;
#1216=CIRCLE ( 'NONE', #6280, 3.000000000000002665 ) ;
#1217=AXIS2_PLACEMENT_3D ( 'NONE', #2379, #11733, #5945 ) ;
#1218=DIRECTION ( 'NONE',  ( 0.000000000000000000, 0.000000000000000000, 1.000000000000000000 ) ) ;
#1221=ORIENTED_EDGE ( 'NONE', *, *, #12597, .F. ) ;
#1222=CARTESIAN_POINT ( 'NONE',  ( 0.000000000000000000, 0.000000000000000000, -10.50000000000000000 ) ) ;
#1223=DIRECTION ( 'NONE',  ( 0.000000000000000000, 0.000000000000000000, 1.000000000000000000 ) ) ;
#1224=CIRCLE ( 'NONE', #3896, 2.649999999999992806 ) ;
#1228=CIRCLE ( 'NONE', #6295, 52.50000000000000711 ) ;
#1233=DIRECTION ( 'NONE',  ( -1.000000000000000000, 0.000000000000000000, 0.000000000000000000 ) ) ;
#1235=VECTOR ( 'NONE', #13228, 1000.000000000000000 ) ;
#1236=DIRECTION ( 'NONE',  ( 0.000000000000000000, 0.000000000000000000, 1.000000000000000000 ) ) ;
#1237=DIRECTION ( 'NONE',  ( -0.000000000000000000, -0.000000000000000000, -1.000000000000000000 ) ) ;
#1238=CARTESIAN_POINT ( 'NONE',  ( 42.50536573064410106, 32.06294366074510549, -13.00000000000000178 ) ) ;
#1239=AXIS2_PLACEMENT_3D ( 'NONE', #1714, #10749, #12053 ) ;
#1240=DIRECTION ( 'NONE',  ( -1.000000000000000000, 0.000000000000000000, 0.000000000000000000 ) ) ;
#1241=VECTOR ( 'NONE', #9615, 1000.000000000000000 ) ;
#1242=ORIENTED_EDGE ( 'NONE', *, *, #5414, .T. ) ;
#1243=EDGE_CURVE ( 'NONE', #10452, #4454, #7337, .T. ) ;
#1244=CARTESIAN_POINT ( 'NONE',  ( -52.54657765281192638, 6.917888187662934563, 8.000000000000000000 ) ) ;
#1245=ORIENTED_EDGE ( 'NONE', *, *, #1497, .T. ) ;
#1246=EDGE_CURVE ( 'NONE', #5385, #6488, #9711, .T. ) ;
#1247=DIRECTION ( 'NONE',  ( -0.000000000000000000, -0.000000000000000000, 1.000000000000000000 ) ) ;
#1248=EDGE_CURVE ( 'NONE', #7084, #6551, #10502, .T. ) ;
#1249=DIRECTION ( 'NONE',  ( 0.000000000000000000, 0.000000000000000000, -1.000000000000000000 ) ) ;
#1251=AXIS2_PLACEMENT_3D ( 'NONE', #2176, #4398, #4475 ) ;
#1253=DIRECTION ( 'NONE',  ( 1.000000000000000000, 0.000000000000000000, 0.000000000000000000 ) ) ;
#1254=ADVANCED_FACE ( 'NONE', ( #3967 ), #1900, .F. ) ;
#1255=VECTOR ( 'NONE', #2315, 1000.000000000000000 ) ;
#1256=ORIENTED_EDGE ( 'NONE', *, *, #12226, .T. ) ;
#1257=AXIS2_PLACEMENT_3D ( 'NONE', #247, #8215, #8072 ) ;
#1258=CARTESIAN_POINT ( 'NONE',  ( -97.00000000000000000, 1.015776140243522349E-12, 8.000000000000000000 ) ) ;
#1260=CARTESIAN_POINT ( 'NONE',  ( 38.26834323650840020, -92.38795325112891987, -8.000000000000000000 ) ) ;
#1261=ORIENTED_EDGE ( 'NONE', *, *, #13537, .T. ) ;
#1262=AXIS2_PLACEMENT_3D ( 'NONE', #11581, #9413, #13926 ) ;
#1264=VERTEX_POINT ( 'NONE', #10169 ) ;
#1265=AXIS2_PLACEMENT_3D ( 'NONE', #61, #11555, #4558 ) ;
#1266=CARTESIAN_POINT ( 'NONE',  ( -92.38795325112826617, 38.26834323650999181, 8.000000000000000000 ) ) ;
#1270=DIRECTION ( 'NONE',  ( 0.000000000000000000, 0.000000000000000000, 1.000000000000000000 ) ) ;
#1271=ORIENTED_EDGE ( 'NONE', *, *, #7692, .T. ) ;
#1272=DIRECTION ( 'NONE',  ( -0.000000000000000000, -0.000000000000000000, -1.000000000000000000 ) ) ;
#1274=ORIENTED_EDGE ( 'NONE', *, *, #11236, .T. ) ;
#1275=AXIS2_PLACEMENT_3D ( 'NONE', #5796, #12652, #14860 ) ;
#1277=VERTEX_POINT ( 'NONE', #11330 ) ;
#1278=DIRECTION ( 'NONE',  ( 0.000000000000000000, 0.000000000000000000, -1.000000000000000000 ) ) ;
#1279=CARTESIAN_POINT ( 'NONE',  ( -39.66766701456180755, -30.43807145043597373, -8.000000000000000000 ) ) ;
#1280=CIRCLE ( 'NONE', #2973, 50.00000000000000000 ) ;
#1281=ORIENTED_EDGE ( 'NONE', *, *, #2771, .T. ) ;
#1282=VERTEX_POINT ( 'NONE', #14597 ) ;
#1283=CARTESIAN_POINT ( 'NONE',  ( -37.12029293941250074, 89.61631465359532456, 8.000000000000000000 ) ) ;
#1284=ORIENTED_EDGE ( 'NONE', *, *, #43, .F. ) ;
#1286=CARTESIAN_POINT ( 'NONE',  ( 30.80502811811196295, 49.00442420936003174, 8.000000000000000000 ) ) ;
#1287=FACE_OUTER_BOUND ( 'NONE', #9145, .T. ) ;
#1289=EDGE_CURVE ( 'NONE', #5235, #3918, #3659, .T. ) ;
#1291=VECTOR ( 'NONE', #5295, 1000.000000000000000 ) ;
#1295=ORIENTED_EDGE ( 'NONE', *, *, #2095, .F. ) ;
#1297=AXIS2_PLACEMENT_3D ( 'NONE', #9572, #1395, #5100 ) ;
#1299=EDGE_CURVE ( 'NONE', #12729, #12788, #5591, .T. ) ;
#1300=VECTOR ( 'NONE', #6477, 1000.000000000000000 ) ;
#1301=DIRECTION ( 'NONE',  ( 0.000000000000000000, 0.000000000000000000, 1.000000000000000000 ) ) ;
#1309=EDGE_CURVE ( 'NONE', #2752, #915, #12866, .T. ) ;
#1310=CIRCLE ( 'NONE', #3500, 60.50000000000000000 ) ;
#1311=DIRECTION ( 'NONE',  ( 0.000000000000000000, 0.000000000000000000, 1.000000000000000000 ) ) ;
#1312=VECTOR ( 'NONE', #6383, 1000.000000000000000 ) ;
#1313=ORIENTED_EDGE ( 'NONE', *, *, #7794, .T. ) ;
#1314=DIRECTION ( 'NONE',  ( 0.000000000000000000, 0.000000000000000000, 1.000000000000000000 ) ) ;
#1317=FACE_OUTER_BOUND ( 'NONE', #9566, .T. ) ;
#1318=ORIENTED_EDGE ( 'NONE', *, *, #9870, .T. ) ;
#1319=AXIS2_PLACEMENT_3D ( 'NONE', #8752, #3075, #12405 ) ;
#1323=AXIS2_PLACEMENT_3D ( 'NONE', #11820, #9877, #9374 ) ;
#1324=ORIENTED_EDGE ( 'NONE', *, *, #10190, .T. ) ;
#1328=FACE_OUTER_BOUND ( 'NONE', #2402, .T. ) ;
#1330=CIRCLE ( 'NONE', #11761, 3.000000000000002665 ) ;
#1331=VERTEX_POINT ( 'NONE', #13372 ) ;
#1332=VECTOR ( 'NONE', #11907, 1000.000000000000000 ) ;
#1333=CARTESIAN_POINT ( 'NONE',  ( -42.04772703543551415, -32.26435573746212526, -8.000000000000000000 ) ) ;
#1337=ADVANCED_FACE ( 'NONE', ( #855 ), #774, .T. ) ;
#1338=VERTEX_POINT ( 'NONE', #13591 ) ;
#1339=ADVANCED_FACE ( 'NONE', ( #11098 ), #7816, .T. ) ;
#1340=ORIENTED_EDGE ( 'NONE', *, *, #10068, .F. ) ;
#1342=EDGE_LOOP ( 'NONE', ( #5577, #448 ) ) ;
#1343=AXIS2_PLACEMENT_3D ( 'NONE', #2632, #359, #7409 ) ;
#1344=CARTESIAN_POINT ( 'NONE',  ( 30.80502811811196295, 49.00442420936003174, -10.50000000000000000 ) ) ;
#1346=CARTESIAN_POINT ( 'NONE',  ( -25.99999999999971223, -45.89934640057541060, -10.50000000000000000 ) ) ;
#1349=CARTESIAN_POINT ( 'NONE',  ( 32.39328945492017198, -42.64958156413663914, -10.50000000000000000 ) ) ;
#1350=EDGE_LOOP ( 'NONE', ( #12664, #5339, #9575, #4664, #14640 ) ) ;
#1351=DIRECTION ( 'NONE',  ( 0.000000000000000000, 0.000000000000000000, -1.000000000000000000 ) ) ;
#1352=ORIENTED_EDGE ( 'NONE', *, *, #14789, .F. ) ;
#1354=ORIENTED_EDGE ( 'NONE', *, *, #1522, .F. ) ;
#1355=CARTESIAN_POINT ( 'NONE',  ( 32.26435573746228158, -42.04772703543541468, -10.50000000000000000 ) ) ;
#1356=DIRECTION ( 'NONE',  ( -1.000000000000000000, 0.000000000000000000, 0.000000000000000000 ) ) ;
#1357=AXIS2_PLACEMENT_3D ( 'NONE', #14345, #1744, #1888 ) ;
#1358=DIRECTION ( 'NONE',  ( -1.000000000000000000, 0.000000000000000000, 0.000000000000000000 ) ) ;
#1359=ADVANCED_FACE ( 'NONE', ( #14672 ), #12463, .T. ) ;
#1360=ORIENTED_EDGE ( 'NONE', *, *, #559, .F. ) ;
#1363=ORIENTED_EDGE ( 'NONE', *, *, #5786, .F. ) ;
#1364=FACE_OUTER_BOUND ( 'NONE', #7802, .T. ) ;
#1365=FACE_OUTER_BOUND ( 'NONE', #5975, .T. ) ;
#1366=VECTOR ( 'NONE', #1205, 1000.000000000000000 ) ;
#1367=PLANE ( 'NONE',  #7399 ) ;
#1368=CARTESIAN_POINT ( 'NONE',  ( -47.21331623427138879, -33.48561063518577896, -13.00000000000000178 ) ) ;
#1369=DIRECTION ( 'NONE',  ( 0.000000000000000000, 0.000000000000000000, 1.000000000000000000 ) ) ;
#1373=ORIENTED_EDGE ( 'NONE', *, *, #8469, .F. ) ;
#1374=AXIS2_PLACEMENT_3D ( 'NONE', #10651, #338, #7159 ) ;
#1375=ORIENTED_EDGE ( 'NONE', *, *, #3011, .T. ) ;
#1376=EDGE_CURVE ( 'NONE', #10004, #13345, #9463, .T. ) ;
#1377=ORIENTED_EDGE ( 'NONE', *, *, #11829, .T. ) ;
#1379=CARTESIAN_POINT ( 'NONE',  ( 20.00000000000000000, 2.449293598294706513E-15, 13.00000000000000178 ) ) ;
#1381=VERTEX_POINT ( 'NONE', #13829 ) ;
#1383=DIRECTION ( 'NONE',  ( 0.000000000000000000, 0.000000000000000000, -1.000000000000000000 ) ) ;
#1384=AXIS2_PLACEMENT_3D ( 'NONE', #5807, #10597, #4765 ) ;
#1385=LINE ( 'NONE', #12014, #5359 ) ;
#1387=AXIS2_PLACEMENT_3D ( 'NONE', #12025, #13293, #10862 ) ;
#1389=ORIENTED_EDGE ( 'NONE', *, *, #14735, .T. ) ;
#1390=EDGE_CURVE ( 'NONE', #12633, #3199, #2202, .T. ) ;
#1391=CARTESIAN_POINT ( 'NONE',  ( 2.449293598294700991E-16, -97.00000000000000000, -8.000000000000000000 ) ) ;
#1393=DIRECTION ( 'NONE',  ( -1.000000000000000000, 0.000000000000000000, 0.000000000000000000 ) ) ;
#1395=DIRECTION ( 'NONE',  ( 0.000000000000000000, 0.000000000000000000, 1.000000000000000000 ) ) ;
#1396=EDGE_CURVE ( 'NONE', #6857, #10287, #13355, .T. ) ;
#1398=EDGE_CURVE ( 'NONE', #2051, #7460, #2433, .T. ) ;
#1399=ORIENTED_EDGE ( 'NONE', *, *, #6844, .F. ) ;
#1400=DIRECTION ( 'NONE',  ( 0.000000000000000000, 0.000000000000000000, 1.000000000000000000 ) ) ;
#1401=VERTEX_POINT ( 'NONE', #6903 ) ;
#1402=CYLINDRICAL_SURFACE ( 'NONE', #14803, 52.50000000000000711 ) ;
#1403=DIRECTION ( 'NONE',  ( -0.000000000000000000, -0.000000000000000000, 1.000000000000000000 ) ) ;
#1404=DIRECTION ( 'NONE',  ( 1.000000000000000000, 0.000000000000000000, 0.000000000000000000 ) ) ;
#1407=DIRECTION ( 'NONE',  ( -1.000000000000000000, 0.000000000000000000, 0.000000000000000000 ) ) ;
#1408=DIRECTION ( 'NONE',  ( -1.000000000000000000, 0.000000000000000000, 0.000000000000000000 ) ) ;
#1409=CARTESIAN_POINT ( 'NONE',  ( -36.62029293941440500, -89.61631465359452875, -10.50000000000000000 ) ) ;
#1410=ORIENTED_EDGE ( 'NONE', *, *, #7578, .T. ) ;
#1411=EDGE_LOOP ( 'NONE', ( #2059, #8484, #7620, #10464, #10607, #1739 ) ) ;
#1412=CIRCLE ( 'NONE', #2135, 59.50000000000000000 ) ;
#1413=DIRECTION ( 'NONE',  ( 1.000000000000000000, 0.000000000000000000, 0.000000000000000000 ) ) ;
#1417=ADVANCED_FACE ( 'NONE', ( #8194 ), #12831, .F. ) ;
#1418=FACE_OUTER_BOUND ( 'NONE', #12269, .T. ) ;
#1419=ORIENTED_EDGE ( 'NONE', *, *, #11505, .F. ) ;
#1420=ORIENTED_EDGE ( 'NONE', *, *, #10091, .T. ) ;
#1424=CARTESIAN_POINT ( 'NONE',  ( 12.86891638962116247, -56.43380494354001087, -13.00000000000000178 ) ) ;
#1427=FACE_OUTER_BOUND ( 'NONE', #7018, .T. ) ;
#1431=EDGE_CURVE ( 'NONE', #5810, #5135, #74, .T. ) ;
#1433=DIRECTION ( 'NONE',  ( -0.000000000000000000, -0.000000000000000000, -1.000000000000000000 ) ) ;
#1434=EDGE_CURVE ( 'NONE', #4396, #13798, #4339, .T. ) ;
#1435=EDGE_CURVE ( 'NONE', #2940, #9073, #12819, .T. ) ;
#1439=ORIENTED_EDGE ( 'NONE', *, *, #9429, .F. ) ;
#1440=FACE_OUTER_BOUND ( 'NONE', #2596, .T. ) ;
#1441=VERTEX_POINT ( 'NONE', #9258 ) ;
#1444=CARTESIAN_POINT ( 'NONE',  ( 45.89934640057532533, -26.49999999999987566, 8.000000000000000000 ) ) ;
#1449=CARTESIAN_POINT ( 'NONE',  ( 0.000000000000000000, 0.000000000000000000, -8.000000000000000000 ) ) ;
#1450=DIRECTION ( 'NONE',  ( -0.000000000000000000, -0.000000000000000000, -1.000000000000000000 ) ) ;
#1452=DIRECTION ( 'NONE',  ( 1.000000000000000000, 0.000000000000000000, -0.000000000000000000 ) ) ;
#1454=CIRCLE ( 'NONE', #11398, 44.89637028918152595 ) ;
#1455=FACE_OUTER_BOUND ( 'NONE', #10690, .T. ) ;
#1456=ORIENTED_EDGE ( 'NONE', *, *, #1154, .T. ) ;
#1457=ADVANCED_FACE ( 'NONE', ( #14972 ), #9334, .F. ) ;
#1458=DIRECTION ( 'NONE',  ( 1.000000000000000000, -2.664535259100375697E-15, 0.000000000000000000 ) ) ;
#1459=DIRECTION ( 'NONE',  ( -0.000000000000000000, -0.000000000000000000, -1.000000000000000000 ) ) ;
#1460=EDGE_CURVE ( 'NONE', #9900, #5810, #11616, .T. ) ;
#1461=FACE_OUTER_BOUND ( 'NONE', #12852, .T. ) ;
#1462=CIRCLE ( 'NONE', #11912, 0.5000000000000004441 ) ;
#1464=ORIENTED_EDGE ( 'NONE', *, *, #14610, .F. ) ;
#1465=AXIS2_PLACEMENT_3D ( 'NONE', #1014, #5557, #7829 ) ;
#1467=VECTOR ( 'NONE', #1991, 1000.000000000000000 ) ;
#1468=VERTEX_POINT ( 'NONE', #13909 ) ;
#1469=DIRECTION ( 'NONE',  ( 0.000000000000000000, 0.000000000000000000, 1.000000000000000000 ) ) ;
#1470=DIRECTION ( 'NONE',  ( 0.000000000000000000, 0.000000000000000000, 1.000000000000000000 ) ) ;
#1471=CARTESIAN_POINT ( 'NONE',  ( -90.10640870805754332, -37.02125851216322872, -10.50000000000000000 ) ) ;
#1472=DIRECTION ( 'NONE',  ( 0.000000000000000000, 0.000000000000000000, 1.000000000000000000 ) ) ;
#1475=AXIS2_PLACEMENT_3D ( 'NONE', #6663, #2120, #11319 ) ;
#1477=EDGE_CURVE ( 'NONE', #6265, #967, #4566, .T. ) ;
#1478=CARTESIAN_POINT ( 'NONE',  ( 30.80502811811196295, 49.00442420936003174, -13.00000000000000178 ) ) ;
#1479=AXIS2_PLACEMENT_3D ( 'NONE', #3814, #10710, #7130 ) ;
#1480=DIRECTION ( 'NONE',  ( 0.000000000000000000, 0.000000000000000000, 1.000000000000000000 ) ) ;
#1481=VECTOR ( 'NONE', #1957, 1000.000000000000000 ) ;
#1483=VERTEX_POINT ( 'NONE', #10476 ) ;
#1484=ADVANCED_FACE ( 'NONE', ( #4641 ), #3503, .F. ) ;
#1485=VERTEX_POINT ( 'NONE', #3175 ) ;
#1486=CIRCLE ( 'NONE', #10218, 0.5000000000000004441 ) ;
#1487=LINE ( 'NONE', #13257, #2797 ) ;
#1488=FACE_OUTER_BOUND ( 'NONE', #7782, .T. ) ;
#1489=AXIS2_PLACEMENT_3D ( 'NONE', #14541, #5279, #3999 ) ;
#1490=CARTESIAN_POINT ( 'NONE',  ( 0.000000000000000000, 0.000000000000000000, 8.000000000000000000 ) ) ;
#1492=CARTESIAN_POINT ( 'NONE',  ( 89.33979373934423052, -36.70371619500547666, -13.00000000000000178 ) ) ;
#1494=CYLINDRICAL_SURFACE ( 'NONE', #13473, 3.000000000000002665 ) ;
#1496=ORIENTED_EDGE ( 'NONE', *, *, #13694, .T. ) ;
#1497=EDGE_CURVE ( 'NONE', #7269, #5893, #5542, .T. ) ;
#1498=EDGE_LOOP ( 'NONE', ( #1221, #1723 ) ) ;
#1499=CARTESIAN_POINT ( 'NONE',  ( 9.706953719245472456, 57.06275842387054098, -8.000000000000000000 ) ) ;
#1500=DIRECTION ( 'NONE',  ( -1.000000000000000000, 0.000000000000000000, 0.000000000000000000 ) ) ;
#1501=AXIS2_PLACEMENT_3D ( 'NONE', #4653, #2297, #5929 ) ;
#1502=CARTESIAN_POINT ( 'NONE',  ( -9.714003807513881483, -53.63365512954690217, -8.000000000000000000 ) ) ;
#1504=AXIS2_PLACEMENT_3D ( 'NONE', #9059, #13707, #3083 ) ;
#1505=ORIENTED_EDGE ( 'NONE', *, *, #3299, .T. ) ;
#1507=ORIENTED_EDGE ( 'NONE', *, *, #302, .T. ) ;
#1509=AXIS2_PLACEMENT_3D ( 'NONE', #4880, #14137, #11641 ) ;
#1514=AXIS2_PLACEMENT_3D ( 'NONE', #12940, #2532, #13860 ) ;
#1515=EDGE_LOOP ( 'NONE', ( #3520, #12611, #7633, #1038, #14892, #4994, #4703, #9659, #13442, #13541, #14353, #12220 ) ) ;
#1516=DIRECTION ( 'NONE',  ( 0.000000000000000000, 0.000000000000000000, 1.000000000000000000 ) ) ;
#1517=VERTEX_POINT ( 'NONE', #7714 ) ;
#1519=AXIS2_PLACEMENT_3D ( 'NONE', #1871, #14937, #9370 ) ;
#1520=ORIENTED_EDGE ( 'NONE', *, *, #9716, .T. ) ;
#1521=DIRECTION ( 'NONE',  ( -0.000000000000000000, -0.000000000000000000, 1.000000000000000000 ) ) ;
#1522=EDGE_CURVE ( 'NONE', #14486, #4561, #13019, .T. ) ;
#1524=CIRCLE ( 'NONE', #13901, 3.000000000000002665 ) ;
#1526=CARTESIAN_POINT ( 'NONE',  ( -68.68541276968778675, 69.08004447556137961, -10.50000000000000000 ) ) ;
#1528=DIRECTION ( 'NONE',  ( 1.000000000000000000, 0.000000000000000000, 0.000000000000000000 ) ) ;
#1529=EDGE_CURVE ( 'NONE', #5666, #3662, #7649, .T. ) ;
#1530=DIRECTION ( 'NONE',  ( 0.000000000000000000, 0.000000000000000000, -1.000000000000000000 ) ) ;
#1532=ORIENTED_EDGE ( 'NONE', *, *, #3615, .F. ) ;
#1534=ORIENTED_EDGE ( 'NONE', *, *, #8925, .T. ) ;
#1536=CARTESIAN_POINT ( 'NONE',  ( 37.12029293941315444, -89.61631465359504034, -13.00000000000000178 ) ) ;
#1538=AXIS2_PLACEMENT_3D ( 'NONE', #9156, #8237, #5669 ) ;
#1539=CARTESIAN_POINT ( 'NONE',  ( 0.000000000000000000, 0.000000000000000000, -10.50000000000000000 ) ) ;
#1540=ADVANCED_FACE ( 'NONE', ( #826 ), #3326, .T. ) ;
#1545=CARTESIAN_POINT ( 'NONE',  ( 0.000000000000000000, 0.000000000000000000, -13.00000000000000178 ) ) ;
#1547=CYLINDRICAL_SURFACE ( 'NONE', #8965, 2.649999999999993694 ) ;
#1548=DIRECTION ( 'NONE',  ( 1.000000000000000000, 0.000000000000000000, 0.000000000000000000 ) ) ;
#1549=CIRCLE ( 'NONE', #13424, 60.50000000000000711 ) ;
#1550=LINE ( 'NONE', #6166, #246 ) ;
#1552=ORIENTED_EDGE ( 'NONE', *, *, #10567, .T. ) ;
#1554=LINE ( 'NONE', #8675, #13700 ) ;
#1556=AXIS2_PLACEMENT_3D ( 'NONE', #14823, #2357, #3 ) ;
#1558=AXIS2_PLACEMENT_3D ( 'NONE', #709, #5266, #8897 ) ;
#1559=ORIENTED_EDGE ( 'NONE', *, *, #6887, .T. ) ;
#1561=ADVANCED_FACE ( 'NONE', ( #10226 ), #909, .F. ) ;
#1562=ORIENTED_EDGE ( 'NONE', *, *, #10190, .F. ) ;
#1565=EDGE_CURVE ( 'NONE', #14343, #2406, #654, .T. ) ;
#1566=DIRECTION ( 'NONE',  ( -1.000000000000000000, 0.000000000000000000, 0.000000000000000000 ) ) ;
#1567=CARTESIAN_POINT ( 'NONE',  ( -51.45950017607691507, 4.121772567811807342, -13.00000000000000178 ) ) ;
#1568=CARTESIAN_POINT ( 'NONE',  ( -89.89283556784485540, 37.53686968382331202, -13.00000000000000178 ) ) ;
#1569=AXIS2_PLACEMENT_3D ( 'NONE', #284, #2561, #9748 ) ;
#1570=ORIENTED_EDGE ( 'NONE', *, *, #5786, .T. ) ;
#1571=EDGE_LOOP ( 'NONE', ( #6998, #4769 ) ) ;
#1572=EDGE_CURVE ( 'NONE', #4906, #10153, #14568, .T. ) ;
#1573=DIRECTION ( 'NONE',  ( 0.000000000000000000, 0.000000000000000000, -1.000000000000000000 ) ) ;
#1574=DIRECTION ( 'NONE',  ( 0.000000000000000000, 0.000000000000000000, 1.000000000000000000 ) ) ;
#1575=DIRECTION ( 'NONE',  ( -1.000000000000000000, 0.000000000000000000, 0.000000000000000000 ) ) ;
#1577=ORIENTED_EDGE ( 'NONE', *, *, #7452, .T. ) ;
#1578=CIRCLE ( 'NONE', #364, 56.99999999999999289 ) ;
#1579=ORIENTED_EDGE ( 'NONE', *, *, #3944, .F. ) ;
#1580=DIRECTION ( 'NONE',  ( -1.000000000000000000, 0.000000000000000000, 0.000000000000000000 ) ) ;
#1581=CIRCLE ( 'NONE', #1102, 0.5000000000000004441 ) ;
#1582=CIRCLE ( 'NONE', #10062, 50.00000000000000000 ) ;
#1583=AXIS2_PLACEMENT_3D ( 'NONE', #12548, #7747, #1990 ) ;
#1584=ORIENTED_EDGE ( 'NONE', *, *, #1752, .T. ) ;
#1585=EDGE_CURVE ( 'NONE', #490, #5159, #11376, .T. ) ;
#1589=VERTEX_POINT ( 'NONE', #9918 ) ;
#1590=CIRCLE ( 'NONE', #7878, 59.50000000000000000 ) ;
#1591=CARTESIAN_POINT ( 'NONE',  ( 89.12622059913255157, 37.21932736666302333, -10.50000000000000000 ) ) ;
#1592=CARTESIAN_POINT ( 'NONE',  ( -68.58935777509570642, -68.58935777509452691, -10.50000000000000000 ) ) ;
#1596=ORIENTED_EDGE ( 'NONE', *, *, #11827, .T. ) ;
#1598=DIRECTION ( 'NONE',  ( 1.000000000000000000, 0.000000000000000000, 0.000000000000000000 ) ) ;
#1599=AXIS2_PLACEMENT_3D ( 'NONE', #11133, #7551, #3090 ) ;
#1600=ORIENTED_EDGE ( 'NONE', *, *, #3757, .F. ) ;
#1603=CARTESIAN_POINT ( 'NONE',  ( -89.61631465359441506, 37.12029293941468211, 8.000000000000000000 ) ) ;
#1604=CARTESIAN_POINT ( 'NONE',  ( 38.79014761921569487, 11.74264578624841171, -28.00000000000000000 ) ) ;
#1605=DIRECTION ( 'NONE',  ( -1.000000000000000000, 0.000000000000000000, 0.000000000000000000 ) ) ;
#1607=VERTEX_POINT ( 'NONE', #1879 ) ;
#1609=AXIS2_PLACEMENT_3D ( 'NONE', #6465, #13312, #874 ) ;
#1613=VERTEX_POINT ( 'NONE', #13498 ) ;
#1614=DIRECTION ( 'NONE',  ( 0.000000000000000000, 0.000000000000000000, 1.000000000000000000 ) ) ;
#1615=FACE_OUTER_BOUND ( 'NONE', #13971, .T. ) ;
#1619=DIRECTION ( 'NONE',  ( 1.000000000000000000, 1.749300984178293162E-15, 0.000000000000000000 ) ) ;
#1620=VERTEX_POINT ( 'NONE', #12356 ) ;
#1623=EDGE_LOOP ( 'NONE', ( #8736, #90 ) ) ;
#1624=DIRECTION ( 'NONE',  ( -0.000000000000000000, -0.000000000000000000, 1.000000000000000000 ) ) ;
#1626=CARTESIAN_POINT ( 'NONE',  ( -23.50071946824040836, -45.96504489226015977, -13.00000000000000178 ) ) ;
#1627=LINE ( 'NONE', #3761, #8085 ) ;
#1629=EDGE_CURVE ( 'NONE', #4561, #5144, #12198, .T. ) ;
#1630=CARTESIAN_POINT ( 'NONE',  ( 0.000000000000000000, 0.000000000000000000, 13.00000000000000178 ) ) ;
#1631=VERTEX_POINT ( 'NONE', #7092 ) ;
#1632=ORIENTED_EDGE ( 'NONE', *, *, #13447, .F. ) ;
#1633=FACE_OUTER_BOUND ( 'NONE', #5273, .T. ) ;
#1634=DIRECTION ( 'NONE',  ( 0.000000000000000000, 0.000000000000000000, 1.000000000000000000 ) ) ;
#1639=VERTEX_POINT ( 'NONE', #4688 ) ;
#1640=DIRECTION ( 'NONE',  ( 0.000000000000000000, 0.000000000000000000, 1.000000000000000000 ) ) ;
#1641=CARTESIAN_POINT ( 'NONE',  ( -26.00011991137315803, -45.91029614918952007, 10.49999999999999822 ) ) ;
#1646=DIRECTION ( 'NONE',  ( 0.000000000000000000, 0.000000000000000000, -1.000000000000000000 ) ) ;
#1648=ADVANCED_FACE ( 'NONE', ( #4544 ), #15015, .F. ) ;
#1652=EDGE_CURVE ( 'NONE', #8710, #7182, #6934, .T. ) ;
#1653=ORIENTED_EDGE ( 'NONE', *, *, #12481, .F. ) ;
#1655=ORIENTED_EDGE ( 'NONE', *, *, #12259, .F. ) ;
#1657=EDGE_CURVE ( 'NONE', #13337, #11105, #10585, .T. ) ;
#1660=CARTESIAN_POINT ( 'NONE',  ( -45.39934640057513349, 26.50000000000019540, -13.00000000000000178 ) ) ;
#1661=CARTESIAN_POINT ( 'NONE',  ( 32.46576781417953583, -41.59008834022656487, -13.00000000000000178 ) ) ;
#1663=DIRECTION ( 'NONE',  ( 0.000000000000000000, 0.000000000000000000, -1.000000000000000000 ) ) ;
#1664=EDGE_CURVE ( 'NONE', #5275, #11092, #6347, .T. ) ;
#1665=EDGE_CURVE ( 'NONE', #13864, #5235, #13973, .T. ) ;
#1666=ORIENTED_EDGE ( 'NONE', *, *, #6511, .F. ) ;
#1667=AXIS2_PLACEMENT_3D ( 'NONE', #2350, #7897, #6970 ) ;
#1668=ORIENTED_EDGE ( 'NONE', *, *, #4410, .T. ) ;
#1669=LINE ( 'NONE', #14582, #12271 ) ;
#1672=DIRECTION ( 'NONE',  ( 0.000000000000000000, 0.000000000000000000, 1.000000000000000000 ) ) ;
#1673=DIRECTION ( 'NONE',  ( -1.000000000000000000, 0.000000000000000000, 0.000000000000000000 ) ) ;
#1674=CYLINDRICAL_SURFACE ( 'NONE', #8245, 0.5000000000000004441 ) ;
#1677=VERTEX_POINT ( 'NONE', #14096 ) ;
#1685=DIRECTION ( 'NONE',  ( -1.000000000000000000, 0.000000000000000000, 0.000000000000000000 ) ) ;
#1686=ORIENTED_EDGE ( 'NONE', *, *, #7580, .F. ) ;
#1687=CARTESIAN_POINT ( 'NONE',  ( -6.451868917687557214, -52.36539807335606156, -10.50000000000000000 ) ) ;
#1688=ORIENTED_EDGE ( 'NONE', *, *, #8973, .F. ) ;
#1694=DIRECTION ( 'NONE',  ( -1.000000000000000000, 0.000000000000000000, 0.000000000000000000 ) ) ;
#1695=CYLINDRICAL_SURFACE ( 'NONE', #7301, 20.00000000000000000 ) ;
#1696=VERTEX_POINT ( 'NONE', #1349 ) ;
#1697=CARTESIAN_POINT ( 'NONE',  ( 0.000000000000000000, 0.000000000000000000, 8.000000000000000000 ) ) ;
#1698=CARTESIAN_POINT ( 'NONE',  ( 50.71110588017602794, 13.58799986788256398, -10.50000000000000000 ) ) ;
#1703=AXIS2_PLACEMENT_3D ( 'NONE', #407, #5185, #14370 ) ;
#1705=AXIS2_PLACEMENT_3D ( 'NONE', #8280, #11857, #12015 ) ;
#1706=ORIENTED_EDGE ( 'NONE', *, *, #800, .T. ) ;
#1707=EDGE_CURVE ( 'NONE', #1207, #7016, #3786, .T. ) ;
#1708=ADVANCED_FACE ( 'NONE', ( #3553 ), #12741, .F. ) ;
#1713=AXIS2_PLACEMENT_3D ( 'NONE', #10559, #12773, #7126 ) ;
#1714=CARTESIAN_POINT ( 'NONE',  ( 0.000000000000000000, 0.000000000000000000, 10.50000000000000000 ) ) ;
#1715=CARTESIAN_POINT ( 'NONE',  ( 51.19406879332056093, 13.71740939043382745, 8.000000000000000000 ) ) ;
#1718=ORIENTED_EDGE ( 'NONE', *, *, #9762, .T. ) ;
#1721=PLANE ( 'NONE',  #12487 ) ;
#1723=ORIENTED_EDGE ( 'NONE', *, *, #7724, .F. ) ;
#1724=AXIS2_PLACEMENT_3D ( 'NONE', #6819, #5763, #3576 ) ;
#1725=AXIS2_PLACEMENT_3D ( 'NONE', #8111, #145, #4486 ) ;
#1727=DIRECTION ( 'NONE',  ( 1.000000000000000000, 0.000000000000000000, -0.000000000000000000 ) ) ;
#1728=EDGE_CURVE ( 'NONE', #2976, #12855, #11753, .T. ) ;
#1729=VECTOR ( 'NONE', #4913, 1000.000000000000000 ) ;
#1731=AXIS2_PLACEMENT_3D ( 'NONE', #520, #10691, #2646 ) ;
#1736=CARTESIAN_POINT ( 'NONE',  ( -49.00442420935969778, 30.80502811811250297, 8.000000000000000000 ) ) ;
#1737=AXIS2_PLACEMENT_3D ( 'NONE', #9236, #9009, #12663 ) ;
#1738=CARTESIAN_POINT ( 'NONE',  ( 6.117650515114745779, 53.20607447915232058, -10.50000000000000000 ) ) ;
#1739=ORIENTED_EDGE ( 'NONE', *, *, #14201, .F. ) ;
#1741=CIRCLE ( 'NONE', #5614, 60.50000000000000000 ) ;
#1742=ORIENTED_EDGE ( 'NONE', *, *, #8597, .T. ) ;
#1743=VERTEX_POINT ( 'NONE', #1134 ) ;
#1744=DIRECTION ( 'NONE',  ( 0.000000000000000000, 0.000000000000000000, 1.000000000000000000 ) ) ;
#1745=CARTESIAN_POINT ( 'NONE',  ( -52.05085522212502980, 6.852625091552908110, -10.50000000000000000 ) ) ;
#1746=EDGE_CURVE ( 'NONE', #9110, #3826, #4272, .T. ) ;
#1747=EDGE_CURVE ( 'NONE', #10698, #10670, #8240, .T. ) ;
#1748=CARTESIAN_POINT ( 'NONE',  ( -86.67575032682103142, -37.71449950291016506, -8.000000000000000000 ) ) ;
#1749=DIRECTION ( 'NONE',  ( 1.000000000000000000, 0.000000000000000000, 0.000000000000000000 ) ) ;
#1750=CYLINDRICAL_SURFACE ( 'NONE', #6767, 3.000000000000002665 ) ;
#1751=DIRECTION ( 'NONE',  ( 0.000000000000000000, 0.000000000000000000, -1.000000000000000000 ) ) ;
#1752=EDGE_CURVE ( 'NONE', #2510, #11469, #9346, .T. ) ;
#1755=DIRECTION ( 'NONE',  ( -1.000000000000000000, -2.775557561562867370E-14, 0.000000000000000000 ) ) ;
#1756=AXIS2_PLACEMENT_3D ( 'NONE', #13488, #3238, #5445 ) ;
#1757=EDGE_CURVE ( 'NONE', #8196, #13119, #2471, .T. ) ;
#1758=CARTESIAN_POINT ( 'NONE',  ( 89.61631465359491244, 37.12029293941346708, 10.49999999999999822 ) ) ;
#1759=CARTESIAN_POINT ( 'NONE',  ( 0.000000000000000000, 0.000000000000000000, 8.000000000000000000 ) ) ;
#1761=ORIENTED_EDGE ( 'NONE', *, *, #1113, .F. ) ;
#1766=ORIENTED_EDGE ( 'NONE', *, *, #8510, .F. ) ;
#1767=VECTOR ( 'NONE', #8926, 1000.000000000000000 ) ;
#1768=AXIS2_PLACEMENT_3D ( 'NONE', #2913, #7693, #8977 ) ;
#1769=ADVANCED_FACE ( 'NONE', ( #9449 ), #9235, .T. ) ;
#1770=DIRECTION ( 'NONE',  ( 0.000000000000000000, 0.000000000000000000, 1.000000000000000000 ) ) ;
#1771=DIRECTION ( 'NONE',  ( 1.000000000000000000, 0.000000000000000000, -0.000000000000000000 ) ) ;
#1772=FACE_OUTER_BOUND ( 'NONE', #3421, .T. ) ;
#1773=VECTOR ( 'NONE', #4961, 1000.000000000000000 ) ;
#1774=DIRECTION ( 'NONE',  ( 1.000000000000000000, 0.000000000000000000, 0.000000000000000000 ) ) ;
#1775=CARTESIAN_POINT ( 'NONE',  ( -26.49999999999971578, -45.89934640057541060, -13.00000000000000178 ) ) ;
#1778=CIRCLE ( 'NONE', #12446, 3.000000000000002665 ) ;
#1781=DIRECTION ( 'NONE',  ( 1.000000000000000000, 0.000000000000000000, 0.000000000000000000 ) ) ;
#1785=DIRECTION ( 'NONE',  ( 1.000000000000000000, -5.329070518200751394E-15, 0.000000000000000000 ) ) ;
#1786=AXIS2_PLACEMENT_3D ( 'NONE', #14852, #2242, #4751 ) ;
#1787=VERTEX_POINT ( 'NONE', #9600 ) ;
#1788=DIRECTION ( 'NONE',  ( -1.000000000000000000, 0.000000000000000000, 0.000000000000000000 ) ) ;
#1790=EDGE_LOOP ( 'NONE', ( #682, #13336, #5718, #4831, #12440, #14577, #6256, #12647, #7287 ) ) ;
#1796=ORIENTED_EDGE ( 'NONE', *, *, #11313, .T. ) ;
#1801=VECTOR ( 'NONE', #11111, 1000.000000000000000 ) ;
#1802=CARTESIAN_POINT ( 'NONE',  ( 42.04772703543530099, 32.26435573746242369, -10.50000000000000000 ) ) ;
#1805=ORIENTED_EDGE ( 'NONE', *, *, #14792, .F. ) ;
#1807=VECTOR ( 'NONE', #5376, 1000.000000000000000 ) ;
#1810=DIRECTION ( 'NONE',  ( 1.000000000000000000, 0.000000000000000000, 0.000000000000000000 ) ) ;
#1813=EDGE_CURVE ( 'NONE', #964, #3662, #8620, .T. ) ;
#1815=AXIS2_PLACEMENT_3D ( 'NONE', #14920, #3300, #2232 ) ;
#1816=CIRCLE ( 'NONE', #11044, 0.5000000000000022204 ) ;
#1817=ORIENTED_EDGE ( 'NONE', *, *, #11647, .F. ) ;
#1819=ORIENTED_EDGE ( 'NONE', *, *, #10834, .T. ) ;
#1821=CARTESIAN_POINT ( 'NONE',  ( 47.21331623427115431, 33.48561063518610581, -8.000000000000000000 ) ) ;
#1822=VECTOR ( 'NONE', #7967, 1000.000000000000000 ) ;
#1823=DIRECTION ( 'NONE',  ( 1.000000000000000000, 0.000000000000000000, 0.000000000000000000 ) ) ;
#1828=DIRECTION ( 'NONE',  ( 0.000000000000000000, 0.000000000000000000, 1.000000000000000000 ) ) ;
#1829=AXIS2_PLACEMENT_3D ( 'NONE', #6635, #6482, #8996 ) ;
#1830=DIRECTION ( 'NONE',  ( 1.000000000000000000, 0.000000000000000000, 0.000000000000000000 ) ) ;
#1834=EDGE_CURVE ( 'NONE', #1124, #8412, #10667, .T. ) ;
#1835=ORIENTED_EDGE ( 'NONE', *, *, #4139, .F. ) ;
#1836=SURFACE_SIDE_STYLE ('',( #12242 ) ) ;
#1837=ORIENTED_EDGE ( 'NONE', *, *, #1497, .F. ) ;
#1838=CARTESIAN_POINT ( 'NONE',  ( 90.10640870805727332, 37.02125851216391794, -10.50000000000000000 ) ) ;
#1839=VERTEX_POINT ( 'NONE', #14395 ) ;
#1840=DIRECTION ( 'NONE',  ( -1.000000000000000000, 0.000000000000000000, 0.000000000000000000 ) ) ;
#1842=CARTESIAN_POINT ( 'NONE',  ( 0.000000000000000000, 0.000000000000000000, 10.50000000000000000 ) ) ;
#1844=DIRECTION ( 'NONE',  ( 1.000000000000000000, 0.000000000000000000, 0.000000000000000000 ) ) ;
#1845=AXIS2_PLACEMENT_3D ( 'NONE', #2246, #480, #1407 ) ;
#1847=DIRECTION ( 'NONE',  ( -1.000000000000000000, 0.000000000000000000, 0.000000000000000000 ) ) ;
#1848=DIRECTION ( 'NONE',  ( 1.000000000000000000, 0.000000000000000000, -0.000000000000000000 ) ) ;
#1851=CARTESIAN_POINT ( 'NONE',  ( 0.000000000000000000, 0.000000000000000000, -28.00000000000000000 ) ) ;
#1853=ADVANCED_FACE ( 'NONE', ( #1418 ), #279, .F. ) ;
#1855=LINE ( 'NONE', #5497, #10009 ) ;
#1861=AXIS2_PLACEMENT_3D ( 'NONE', #6721, #12584, #7870 ) ;
#1862=CYLINDRICAL_SURFACE ( 'NONE', #4505, 60.49999999999999289 ) ;
#1865=CARTESIAN_POINT ( 'NONE',  ( 33.48561063518626923, -47.21331623427104063, 8.000000000000000000 ) ) ;
#1867=CIRCLE ( 'NONE', #10351, 50.00000000000000000 ) ;
#1869=DIRECTION ( 'NONE',  ( 1.000000000000000000, 0.000000000000000000, 0.000000000000000000 ) ) ;
#1871=CARTESIAN_POINT ( 'NONE',  ( 13.71740939043365337, -51.19406879332061067, -10.50000000000000000 ) ) ;
#1872=ORIENTED_EDGE ( 'NONE', *, *, #12364, .T. ) ;
#1873=ORIENTED_EDGE ( 'NONE', *, *, #10811, .T. ) ;
#1874=ORIENTED_EDGE ( 'NONE', *, *, #8851, .F. ) ;
#1875=EDGE_CURVE ( 'NONE', #914, #5501, #12055, .T. ) ;
#1878=( NAMED_UNIT ( * ) PLANE_ANGLE_UNIT ( ) SI_UNIT ( $, .RADIAN. ) );
#1879=CARTESIAN_POINT ( 'NONE',  ( -2.649999999999987921, 38.00000000000000000, -28.00000000000000000 ) ) ;
#1882=DIRECTION ( 'NONE',  ( 0.000000000000000000, 0.000000000000000000, 1.000000000000000000 ) ) ;
#1886=VERTEX_POINT ( 'NONE', #5055 ) ;
#1887=VERTEX_POINT ( 'NONE', #9664 ) ;
#1888=DIRECTION ( 'NONE',  ( 1.000000000000000000, 0.000000000000000000, 0.000000000000000000 ) ) ;
#1889=ADVANCED_FACE ( 'NONE', ( #3927 ), #1494, .T. ) ;
#1890=EDGE_CURVE ( 'NONE', #14215, #2940, #7895, .T. ) ;
#1891=EDGE_CURVE ( 'NONE', #14224, #2518, #9101, .T. ) ;
#1892=CARTESIAN_POINT ( 'NONE',  ( 50.13108361037843252, 56.43380494353993271, -8.000000000000000000 ) ) ;
#1894=FACE_BOUND ( 'NONE', #1623, .T. ) ;
#1895=DIRECTION ( 'NONE',  ( 1.000000000000000000, 0.000000000000000000, 0.000000000000000000 ) ) ;
#1898=CARTESIAN_POINT ( 'NONE',  ( 0.2790467552932217044, -96.58511096861892042, -10.50000000000000000 ) ) ;
#1900=CYLINDRICAL_SURFACE ( 'NONE', #4877, 0.5000000000000004441 ) ;
#1902=( NAMED_UNIT ( * ) PLANE_ANGLE_UNIT ( ) SI_UNIT ( $, .RADIAN. ) );
#1903=CARTESIAN_POINT ( 'NONE',  ( 48.29629131445336299, 12.94095225512624303, 8.000000000000000000 ) ) ;
#1904=ORIENTED_EDGE ( 'NONE', *, *, #7578, .F. ) ;
#1906=VERTEX_POINT ( 'NONE', #8917 ) ;
#1907=EDGE_LOOP ( 'NONE', ( #14747, #12378, #1018, #1761 ) ) ;
#1908=DIRECTION ( 'NONE',  ( -0.000000000000000000, -0.000000000000000000, -1.000000000000000000 ) ) ;
#1910=CARTESIAN_POINT ( 'NONE',  ( 51.79945067148123883, 13.60620885621592002, -10.50000000000000000 ) ) ;
#1911=FACE_OUTER_BOUND ( 'NONE', #12810, .T. ) ;
#1912=EDGE_CURVE ( 'NONE', #6451, #11873, #1123, .T. ) ;
#1913=LINE ( 'NONE', #5419, #1312 ) ;
#1914=VECTOR ( 'NONE', #14060, 1000.000000000000000 ) ;
#1917=FACE_OUTER_BOUND ( 'NONE', #5552, .T. ) ;
#1918=DIRECTION ( 'NONE',  ( -1.000000000000000000, 0.000000000000000000, 0.000000000000000000 ) ) ;
#1919=CARTESIAN_POINT ( 'NONE',  ( 90.11631465359491244, 37.12029293941346708, 10.49999999999999822 ) ) ;
#1921=ORIENTED_EDGE ( 'NONE', *, *, #458, .F. ) ;
#1922=CARTESIAN_POINT ( 'NONE',  ( -47.21331623427138879, -33.48561063518577896, 10.49999999999999822 ) ) ;
#1924=VERTEX_POINT ( 'NONE', #14634 ) ;
#1926=DIRECTION ( 'NONE',  ( 0.000000000000000000, 0.000000000000000000, 1.000000000000000000 ) ) ;
#1927=ORIENTED_EDGE ( 'NONE', *, *, #6462, .F. ) ;
#1930=EDGE_CURVE ( 'NONE', #4116, #8471, #9582, .T. ) ;
#1932=ORIENTED_EDGE ( 'NONE', *, *, #3289, .T. ) ;
#1935=VERTEX_POINT ( 'NONE', #2932 ) ;
#1936=ORIENTED_EDGE ( 'NONE', *, *, #7601, .T. ) ;
#1939=AXIS2_PLACEMENT_3D ( 'NONE', #5787, #1108, #5723 ) ;
#1940=CARTESIAN_POINT ( 'NONE',  ( -26.99988008862626643, -45.88839665196127271, -13.00000000000000178 ) ) ;
#1942=DIRECTION ( 'NONE',  ( 0.000000000000000000, 0.000000000000000000, 1.000000000000000000 ) ) ;
#1943=ORIENTED_EDGE ( 'NONE', *, *, #9597, .F. ) ;
#1944=EDGE_CURVE ( 'NONE', #11994, #12800, #14205, .T. ) ;
#1947=ORIENTED_EDGE ( 'NONE', *, *, #2820, .T. ) ;
#1948=CIRCLE ( 'NONE', #10432, 60.50000000000000000 ) ;
#1949=CARTESIAN_POINT ( 'NONE',  ( 38.79014761921568777, 11.74264578624841171, -28.00000000000000000 ) ) ;
#1951=EDGE_CURVE ( 'NONE', #1381, #2743, #6422, .T. ) ;
#1952=AXIS2_PLACEMENT_3D ( 'NONE', #10612, #211, #11772 ) ;
#1953=FACE_OUTER_BOUND ( 'NONE', #6368, .T. ) ;
#1956=EDGE_LOOP ( 'NONE', ( #7658, #2818, #11568, #9147, #13939, #884 ) ) ;
#1957=DIRECTION ( 'NONE',  ( -0.000000000000000000, -0.000000000000000000, 1.000000000000000000 ) ) ;
#1959=ORIENTED_EDGE ( 'NONE', *, *, #1746, .T. ) ;
#1960=CIRCLE ( 'NONE', #9699, 59.50000000000000000 ) ;
#1961=CARTESIAN_POINT ( 'NONE',  ( 97.50000000000000000, -3.384287605079545030E-13, -10.50000000000000000 ) ) ;
#1962=EDGE_LOOP ( 'NONE', ( #4881, #11336, #10308, #6264, #3877, #3089 ) ) ;
#1963=CIRCLE ( 'NONE', #12393, 60.50000000000000000 ) ;
#1964=AXIS2_PLACEMENT_3D ( 'NONE', #10770, #4019, #9764 ) ;
#1966=CYLINDRICAL_SURFACE ( 'NONE', #11306, 3.000000000000002665 ) ;
#1967=PLANE ( 'NONE',  #8496 ) ;
#1969=FACE_OUTER_BOUND ( 'NONE', #837, .T. ) ;
#1971=CARTESIAN_POINT ( 'NONE',  ( -14.07862063237857342, 50.84834283437004387, 10.49999999999999822 ) ) ;
#1972=CIRCLE ( 'NONE', #5846, 60.50000000000000000 ) ;
#1973=ORIENTED_EDGE ( 'NONE', *, *, #14260, .T. ) ;
#1977=DIRECTION ( 'NONE',  ( -1.000000000000000000, 0.000000000000000000, 0.000000000000000000 ) ) ;
#1978=CARTESIAN_POINT ( 'NONE',  ( 13.71740939043365337, -51.19406879332061067, -13.00000000000000178 ) ) ;
#1979=EDGE_CURVE ( 'NONE', #6594, #3549, #6409, .T. ) ;
#1980=AXIS2_PLACEMENT_3D ( 'NONE', #11041, #3623, #8747 ) ;
#1983=ORIENTED_EDGE ( 'NONE', *, *, #2278, .T. ) ;
#1984=DIRECTION ( 'NONE',  ( 0.000000000000000000, 0.000000000000000000, 1.000000000000000000 ) ) ;
#1985=AXIS2_PLACEMENT_3D ( 'NONE', #8037, #13580, #11320 ) ;
#1987=CARTESIAN_POINT ( 'NONE',  ( 0.000000000000000000, 0.000000000000000000, -10.50000000000000000 ) ) ;
#1990=DIRECTION ( 'NONE',  ( -1.000000000000000000, 0.000000000000000000, 0.000000000000000000 ) ) ;
#1991=DIRECTION ( 'NONE',  ( 0.000000000000000000, 0.000000000000000000, 1.000000000000000000 ) ) ;
#1992=DIRECTION ( 'NONE',  ( 1.000000000000000000, 0.000000000000000000, 0.000000000000000000 ) ) ;
#1993=DIRECTION ( 'NONE',  ( 1.000000000000000000, 0.000000000000000000, 0.000000000000000000 ) ) ;
#1994=CYLINDRICAL_SURFACE ( 'NONE', #13203, 0.5000000000000038858 ) ;
#1997=CIRCLE ( 'NONE', #1046, 3.000000000000002665 ) ;
#1998=ADVANCED_FACE ( 'NONE', ( #7635 ), #12201, .T. ) ;
#1999=DIRECTION ( 'NONE',  ( 0.000000000000000000, 0.000000000000000000, 1.000000000000000000 ) ) ;
#2001=DIRECTION ( 'NONE',  ( 1.000000000000000000, 0.000000000000000000, 0.000000000000000000 ) ) ;
#2004=ORIENTED_EDGE ( 'NONE', *, *, #1008, .T. ) ;
#2005=CARTESIAN_POINT ( 'NONE',  ( 68.68541276968825571, -69.08004447556089644, -13.00000000000000178 ) ) ;
#2006=EDGE_LOOP ( 'NONE', ( #5820, #12503, #5156, #9195 ) ) ;
#2008=LINE ( 'NONE', #14702, #12657 ) ;
#2009=AXIS2_PLACEMENT_3D ( 'NONE', #10521, #4611, #3471 ) ;
#2010=CARTESIAN_POINT ( 'NONE',  ( -68.08935777509570642, -68.58935777509452691, -13.00000000000000178 ) ) ;
#2011=CARTESIAN_POINT ( 'NONE',  ( 97.00000000000000000, -3.384287605079545030E-13, -10.50000000000000000 ) ) ;
#2013=ORIENTED_EDGE ( 'NONE', *, *, #7396, .T. ) ;
#2014=VERTEX_POINT ( 'NONE', #7784 ) ;
#2020=ORIENTED_EDGE ( 'NONE', *, *, #3944, .T. ) ;
#2021=EDGE_CURVE ( 'NONE', #2752, #9052, #3302, .T. ) ;
#2022=CIRCLE ( 'NONE', #11732, 59.50000000000000000 ) ;
#2023=EDGE_CURVE ( 'NONE', #1639, #1264, #7705, .T. ) ;
#2024=EDGE_LOOP ( 'NONE', ( #3147, #13532, #9238, #14993, #2848, #8079, #6197, #9100, #13934, #3016, #4925, #7406 ) ) ;
#2029=CARTESIAN_POINT ( 'NONE',  ( -68.58935777509570642, -68.58935777509452691, 10.49999999999999822 ) ) ;
#2033=AXIS2_PLACEMENT_3D ( 'NONE', #8078, #6932, #32 ) ;
#2034=ORIENTED_EDGE ( 'NONE', *, *, #8597, .F. ) ;
#2035=LINE ( 'NONE', #753, #1481 ) ;
#2037=ORIENTED_EDGE ( 'NONE', *, *, #4269, .F. ) ;
#2038=DIRECTION ( 'NONE',  ( -0.000000000000000000, -0.000000000000000000, 1.000000000000000000 ) ) ;
#2040=EDGE_CURVE ( 'NONE', #11760, #11078, #3545, .T. ) ;
#2041=ORIENTED_EDGE ( 'NONE', *, *, #8973, .T. ) ;
#2043=CIRCLE ( 'NONE', #5440, 63.00000000000000000 ) ;
#2044=CIRCLE ( 'NONE', #8575, 63.00000000000000000 ) ;
#2045=AXIS2_PLACEMENT_3D ( 'NONE', #13018, #2534, #11879 ) ;
#2046=LINE ( 'NONE', #8939, #5832 ) ;
#2048=DIRECTION ( 'NONE',  ( 1.000000000000000000, 0.000000000000000000, 0.000000000000000000 ) ) ;
#2049=DIRECTION ( 'NONE',  ( 0.000000000000000000, 0.000000000000000000, 1.000000000000000000 ) ) ;
#2050=CARTESIAN_POINT ( 'NONE',  ( 0.000000000000000000, 0.000000000000000000, -8.000000000000000000 ) ) ;
#2051=VERTEX_POINT ( 'NONE', #13947 ) ;
#2055=AXIS2_PLACEMENT_3D ( 'NONE', #9914, #7711, #13494 ) ;
#2057=DIRECTION ( 'NONE',  ( 0.000000000000000000, 0.000000000000000000, 1.000000000000000000 ) ) ;
#2059=ORIENTED_EDGE ( 'NONE', *, *, #451, .T. ) ;
#2060=FACE_OUTER_BOUND ( 'NONE', #12721, .T. ) ;
#2061=AXIS2_PLACEMENT_3D ( 'NONE', #6290, #9869, #13451 ) ;
#2066=DIRECTION ( 'NONE',  ( 0.000000000000000000, 0.000000000000000000, 1.000000000000000000 ) ) ;
#2067=CARTESIAN_POINT ( 'NONE',  ( -45.83364790889027773, 29.49928053175948506, -8.000000000000000000 ) ) ;
#2068=DIRECTION ( 'NONE',  ( 0.000000000000000000, 0.000000000000000000, 1.000000000000000000 ) ) ;
#2069=ADVANCED_FACE ( 'NONE', ( #10363 ), #4672, .T. ) ;
#2070=DIRECTION ( 'NONE',  ( 1.000000000000000000, 0.000000000000000000, 0.000000000000000000 ) ) ;
#2071=DIRECTION ( 'NONE',  ( -0.000000000000000000, -0.000000000000000000, -1.000000000000000000 ) ) ;
#2074=ORIENTED_EDGE ( 'NONE', *, *, #9353, .F. ) ;
#2075=DIRECTION ( 'NONE',  ( 1.000000000000000000, 0.000000000000000000, 0.000000000000000000 ) ) ;
#2080=DIRECTION ( 'NONE',  ( 1.000000000000000000, 0.000000000000000000, 0.000000000000000000 ) ) ;
#2082=VECTOR ( 'NONE', #11899, 1000.000000000000000 ) ;
#2084=CIRCLE ( 'NONE', #10569, 57.00000000000000000 ) ;
#2085=VERTEX_POINT ( 'NONE', #14935 ) ;
#2087=ADVANCED_FACE ( 'NONE', ( #12724 ), #10291, .F. ) ;
#2088=DIRECTION ( 'NONE',  ( -0.000000000000000000, -0.000000000000000000, 1.000000000000000000 ) ) ;
#2090=VERTEX_POINT ( 'NONE', #6937 ) ;
#2092=DIRECTION ( 'NONE',  ( -1.000000000000000000, 0.000000000000000000, 0.000000000000000000 ) ) ;
#2094=VERTEX_POINT ( 'NONE', #6777 ) ;
#2095=EDGE_CURVE ( 'NONE', #3662, #6497, #13746, .T. ) ;
#2099=CARTESIAN_POINT ( 'NONE',  ( -3.492805317593278058, 46.55633131742322917, -10.50000000000000000 ) ) ;
#2100=ORIENTED_EDGE ( 'NONE', *, *, #8157, .T. ) ;
#2101=ORIENTED_EDGE ( 'NONE', *, *, #11960, .F. ) ;
#2102=EDGE_LOOP ( 'NONE', ( #6144, #14266, #378, #1064 ) ) ;
#2103=CIRCLE ( 'NONE', #2833, 3.000000000000002665 ) ;
#2105=CARTESIAN_POINT ( 'NONE',  ( -13.71740939043329277, 51.19406879332069593, -10.50000000000000000 ) ) ;
#2107=DIRECTION ( 'NONE',  ( 0.000000000000000000, 0.000000000000000000, -1.000000000000000000 ) ) ;
#2109=FACE_BOUND ( 'NONE', #8563, .T. ) ;
#2110=DIRECTION ( 'NONE',  ( 1.000000000000000000, 0.000000000000000000, -0.000000000000000000 ) ) ;
#2111=EDGE_CURVE ( 'NONE', #13137, #13279, #6687, .T. ) ;
#2112=ORIENTED_EDGE ( 'NONE', *, *, #6887, .F. ) ;
#2116=ORIENTED_EDGE ( 'NONE', *, *, #12114, .F. ) ;
#2118=EDGE_CURVE ( 'NONE', #11737, #13523, #5959, .T. ) ;
#2119=VERTEX_POINT ( 'NONE', #11665 ) ;
#2120=DIRECTION ( 'NONE',  ( 0.000000000000000000, 0.000000000000000000, 1.000000000000000000 ) ) ;
#2122=DIRECTION ( 'NONE',  ( 0.000000000000000000, 0.000000000000000000, 1.000000000000000000 ) ) ;
#2126=EDGE_CURVE ( 'NONE', #12800, #12895, #4766, .T. ) ;
#2127=ORIENTED_EDGE ( 'NONE', *, *, #5878, .F. ) ;
#2131=ORIENTED_EDGE ( 'NONE', *, *, #9963, .F. ) ;
#2134=DIRECTION ( 'NONE',  ( 0.000000000000000000, 0.000000000000000000, 1.000000000000000000 ) ) ;
#2135=AXIS2_PLACEMENT_3D ( 'NONE', #8102, #2337, #12815 ) ;
#2136=CARTESIAN_POINT ( 'NONE',  ( 45.83364790889049090, -29.49928053175916887, -13.00000000000000178 ) ) ;
#2137=DIRECTION ( 'NONE',  ( -1.000000000000000000, 0.000000000000000000, 0.000000000000000000 ) ) ;
#2140=DIRECTION ( 'NONE',  ( -1.000000000000000000, 0.000000000000000000, 0.000000000000000000 ) ) ;
#2142=ORIENTED_EDGE ( 'NONE', *, *, #7165, .F. ) ;
#2143=CARTESIAN_POINT ( 'NONE',  ( 0.000000000000000000, 0.000000000000000000, 8.000000000000000000 ) ) ;
#2144=VERTEX_POINT ( 'NONE', #8161 ) ;
#2146=DIRECTION ( 'NONE',  ( 1.000000000000000000, 0.000000000000000000, 0.000000000000000000 ) ) ;
#2147=DIRECTION ( 'NONE',  ( 0.000000000000000000, 0.000000000000000000, -1.000000000000000000 ) ) ;
#2148=DIRECTION ( 'NONE',  ( 0.000000000000000000, 0.000000000000000000, 1.000000000000000000 ) ) ;
#2149=VERTEX_POINT ( 'NONE', #4458 ) ;
#2150=CARTESIAN_POINT ( 'NONE',  ( 39.30189486418243661, 33.47282819776626894, -8.000000000000000000 ) ) ;
#2152=CARTESIAN_POINT ( 'NONE',  ( 42.04772703543530099, 32.26435573746242369, 8.000000000000000000 ) ) ;
#2154=CARTESIAN_POINT ( 'NONE',  ( 39.61975340586557337, 91.27544013909754028, -8.000000000000000000 ) ) ;
#2155=DIRECTION ( 'NONE',  ( 0.000000000000000000, 0.000000000000000000, 1.000000000000000000 ) ) ;
#2157=ORIENTED_EDGE ( 'NONE', *, *, #4361, .F. ) ;
#2158=ORIENTED_EDGE ( 'NONE', *, *, #8886, .T. ) ;
#2159=EDGE_CURVE ( 'NONE', #8152, #4787, #8872, .T. ) ;
#2162=EDGE_CURVE ( 'NONE', #14615, #10761, #10089, .T. ) ;
#2163=FACE_OUTER_BOUND ( 'NONE', #14405, .T. ) ;
#2164=ADVANCED_FACE ( 'NONE', ( #11527 ), #3315, .F. ) ;
#2166=EDGE_LOOP ( 'NONE', ( #3676, #4232, #10209, #586 ) ) ;
#2167=AXIS2_PLACEMENT_3D ( 'NONE', #8647, #6281, #13288 ) ;
#2168=ORIENTED_EDGE ( 'NONE', *, *, #14901, .T. ) ;
#2171=VECTOR ( 'NONE', #12032, 1000.000000000000000 ) ;
#2174=CARTESIAN_POINT ( 'NONE',  ( 0.000000000000000000, 0.000000000000000000, -8.000000000000000000 ) ) ;
#2175=ORIENTED_EDGE ( 'NONE', *, *, #11477, .F. ) ;
#2176=CARTESIAN_POINT ( 'NONE',  ( -26.49999999999971578, -45.89934640057541060, 8.000000000000000000 ) ) ;
#2178=CIRCLE ( 'NONE', #5335, 3.000000000000002665 ) ;
#2179=EDGE_CURVE ( 'NONE', #2876, #12336, #12046, .T. ) ;
#2183=ORIENTED_EDGE ( 'NONE', *, *, #4231, .T. ) ;
#2185=VECTOR ( 'NONE', #703, 1000.000000000000000 ) ;
#2186=EDGE_LOOP ( 'NONE', ( #3065, #6709, #2536, #9817, #10492, #1577, #4627, #4554, #8167, #12707, #634 ) ) ;
#2187=DIRECTION ( 'NONE',  ( 1.000000000000000000, 0.000000000000000000, 0.000000000000000000 ) ) ;
#2188=AXIS2_PLACEMENT_3D ( 'NONE', #3211, #941, #14687 ) ;
#2189=AXIS2_PLACEMENT_3D ( 'NONE', #11339, #6458, #1771 ) ;
#2190=ORIENTED_EDGE ( 'NONE', *, *, #9392, .T. ) ;
#2194=DIRECTION ( 'NONE',  ( 0.000000000000000000, 0.000000000000000000, 1.000000000000000000 ) ) ;
#2195=DIRECTION ( 'NONE',  ( 1.000000000000000000, 0.000000000000000000, 0.000000000000000000 ) ) ;
#2199=ORIENTED_EDGE ( 'NONE', *, *, #6005, .T. ) ;
#2200=CIRCLE ( 'NONE', #3171, 59.49999999999999289 ) ;
#2201=DIRECTION ( 'NONE',  ( -0.000000000000000000, -0.000000000000000000, -1.000000000000000000 ) ) ;
#2202=CIRCLE ( 'NONE', #11426, 53.55662432702593634 ) ;
#2205=CARTESIAN_POINT ( 'NONE',  ( -13.71740939043329277, 51.19406879332069593, -8.000000000000000000 ) ) ;
#2206=ORIENTED_EDGE ( 'NONE', *, *, #8195, .T. ) ;
#2207=CYLINDRICAL_SURFACE ( 'NONE', #5469, 63.00000000000000000 ) ;
#2208=CIRCLE ( 'NONE', #14821, 2.649999999999992806 ) ;
#2211=AXIS2_PLACEMENT_3D ( 'NONE', #3555, #5596, #2334 ) ;
#2212=LINE ( 'NONE', #5550, #8334 ) ;
#2213=ADVANCED_FACE ( 'NONE', ( #6237 ), #260, .F. ) ;
#2215=DIRECTION ( 'NONE',  ( 1.000000000000000000, 0.000000000000000000, 0.000000000000000000 ) ) ;
#2217=EDGE_CURVE ( 'NONE', #3842, #3184, #11317, .T. ) ;
#2218=ADVANCED_FACE ( 'NONE', ( #5043 ), #7228, .T. ) ;
#2220=CYLINDRICAL_SURFACE ( 'NONE', #14187, 0.5000000000000073275 ) ;
#2221=CARTESIAN_POINT ( 'NONE',  ( 13.58799986788239345, -50.71110588017607768, -10.50000000000000000 ) ) ;
#2223=DIRECTION ( 'NONE',  ( 0.000000000000000000, 0.000000000000000000, -1.000000000000000000 ) ) ;
#2224=EDGE_CURVE ( 'NONE', #13003, #10670, #5007, .T. ) ;
#2225=CARTESIAN_POINT ( 'NONE',  ( 37.12029293941379393, 89.61631465359479876, -8.000000000000000000 ) ) ;
#2226=AXIS2_PLACEMENT_3D ( 'NONE', #11378, #50, #1136 ) ;
#2229=CARTESIAN_POINT ( 'NONE',  ( 37.12029293941315444, -89.61631465359504034, -10.50000000000000000 ) ) ;
#2230=CIRCLE ( 'NONE', #11206, 56.99999999999999289 ) ;
#2231=DIRECTION ( 'NONE',  ( 0.000000000000000000, 0.000000000000000000, 1.000000000000000000 ) ) ;
#2232=DIRECTION ( 'NONE',  ( 1.000000000000000000, 0.000000000000000000, 0.000000000000000000 ) ) ;
#2233=EDGE_CURVE ( 'NONE', #10670, #13141, #4288, .T. ) ;
#2234=ORIENTED_EDGE ( 'NONE', *, *, #12386, .T. ) ;
#2237=AXIS2_PLACEMENT_3D ( 'NONE', #10412, #12699, #10344 ) ;
#2238=PLANE ( 'NONE',  #10183 ) ;
#2239=PLANE ( 'NONE',  #4437 ) ;
#2242=DIRECTION ( 'NONE',  ( 0.000000000000000000, 0.000000000000000000, -1.000000000000000000 ) ) ;
#2246=CARTESIAN_POINT ( 'NONE',  ( -52.54657765281192638, 6.917888187662934563, -10.50000000000000000 ) ) ;
#2248=AXIS2_PLACEMENT_3D ( 'NONE', #2322, #13795, #7082 ) ;
#2251=EDGE_LOOP ( 'NONE', ( #8830, #6113, #2806, #12169, #4823 ) ) ;
#2252=EDGE_LOOP ( 'NONE', ( #8931, #3560, #14048, #14172, #2312 ) ) ;
#2253=LINE ( 'NONE', #5881, #12726 ) ;
#2254=AXIS2_PLACEMENT_3D ( 'NONE', #8603, #12949, #11816 ) ;
#2255=CARTESIAN_POINT ( 'NONE',  ( 47.63108361037843252, 56.43380494353993271, -13.00000000000000178 ) ) ;
#2256=CARTESIAN_POINT ( 'NONE',  ( -6.526309611002563571, -49.57224306869052555, 8.000000000000000000 ) ) ;
#2258=EDGE_CURVE ( 'NONE', #7227, #1401, #3554, .T. ) ;
#2260=EDGE_CURVE ( 'NONE', #5532, #9310, #3069, .T. ) ;
#2262=DIRECTION ( 'NONE',  ( -1.000000000000000000, 7.988474494414204077E-14, 0.000000000000000000 ) ) ;
#2263=AXIS2_PLACEMENT_3D ( 'NONE', #3445, #1237, #3522 ) ;
#2266=DIRECTION ( 'NONE',  ( 1.000000000000000000, 0.000000000000000000, 0.000000000000000000 ) ) ;
#2267=CIRCLE ( 'NONE', #10987, 60.50000000000000000 ) ;
#2268=ORIENTED_EDGE ( 'NONE', *, *, #8857, .T. ) ;
#2270=ORIENTED_EDGE ( 'NONE', *, *, #6263, .F. ) ;
#2271=CARTESIAN_POINT ( 'NONE',  ( -89.61631465359441506, 37.12029293941468211, -8.000000000000000000 ) ) ;
#2274=DIRECTION ( 'NONE',  ( 0.000000000000000000, 0.000000000000000000, 1.000000000000000000 ) ) ;
#2278=EDGE_CURVE ( 'NONE', #4906, #12796, #11062, .T. ) ;
#2280=ADVANCED_FACE ( 'NONE', ( #11883 ), #8384, .F. ) ;
#2283=CARTESIAN_POINT ( 'NONE',  ( -2.649999999999994138, 38.00000000000000000, -25.50000000000000355 ) ) ;
#2287=CYLINDRICAL_SURFACE ( 'NONE', #10312, 63.00000000000000000 ) ;
#2289=ORIENTED_EDGE ( 'NONE', *, *, #8692, .T. ) ;
#2290=FACE_OUTER_BOUND ( 'NONE', #14783, .T. ) ;
#2292=DIRECTION ( 'NONE',  ( -1.000000000000000000, 0.000000000000000000, 0.000000000000000000 ) ) ;
#2293=CARTESIAN_POINT ( 'NONE',  ( -53.63365512954686665, 9.714003807514082212, -8.000000000000000000 ) ) ;
#2294=VECTOR ( 'NONE', #2942, 1000.000000000000000 ) ;
#2296=EDGE_CURVE ( 'NONE', #218, #6283, #9841, .T. ) ;
#2297=DIRECTION ( 'NONE',  ( -0.000000000000000000, -0.000000000000000000, -1.000000000000000000 ) ) ;
#2298=ORIENTED_EDGE ( 'NONE', *, *, #2956, .T. ) ;
#2299=ADVANCED_FACE ( 'NONE', ( #8307 ), #184, .T. ) ;
#2300=CARTESIAN_POINT ( 'NONE',  ( -47.21331623427138879, -33.48561063518577896, -8.000000000000000000 ) ) ;
#2301=CARTESIAN_POINT ( 'NONE',  ( -2.449293598294700991E-16, 97.00000000000000000, -13.00000000000000178 ) ) ;
#2302=AXIS2_PLACEMENT_3D ( 'NONE', #12970, #4702, #14035 ) ;
#2303=EDGE_CURVE ( 'NONE', #1186, #12429, #6434, .T. ) ;
#2304=CARTESIAN_POINT ( 'NONE',  ( 0.000000000000000000, 0.000000000000000000, -10.50000000000000000 ) ) ;
#2306=CIRCLE ( 'NONE', #7386, 3.000000000000004441 ) ;
#2307=VECTOR ( 'NONE', #12695, 1000.000000000000000 ) ;
#2308=DIRECTION ( 'NONE',  ( -1.000000000000000000, -6.215849497113533642E-14, 0.000000000000000000 ) ) ;
#2309=ORIENTED_EDGE ( 'NONE', *, *, #6700, .T. ) ;
#2310=ADVANCED_FACE ( 'NONE', ( #1633 ), #11814, .T. ) ;
#2312=ORIENTED_EDGE ( 'NONE', *, *, #2949, .F. ) ;
#2313=CARTESIAN_POINT ( 'NONE',  ( -12.86891638962156215, 56.43380494353993271, -8.000000000000000000 ) ) ;
#2314=AXIS2_PLACEMENT_3D ( 'NONE', #10638, #10722, #13078 ) ;
#2315=DIRECTION ( 'NONE',  ( 0.000000000000000000, 0.000000000000000000, 1.000000000000000000 ) ) ;
#2316=CARTESIAN_POINT ( 'NONE',  ( 46.81487971942603110, -26.01305530232578533, -10.50000000000000000 ) ) ;
#2317=ADVANCED_FACE ( 'NONE', ( #4979, #9587 ), #3835, .T. ) ;
#2318=ORIENTED_EDGE ( 'NONE', *, *, #3202, .F. ) ;
#2319=EDGE_CURVE ( 'NONE', #8810, #8589, #5422, .T. ) ;
#2322=CARTESIAN_POINT ( 'NONE',  ( -30.80502811811232888, -49.00442420935981147, 10.49999999999999822 ) ) ;
#2324=VECTOR ( 'NONE', #7884, 1000.000000000000000 ) ;
#2328=CARTESIAN_POINT ( 'NONE',  ( -65.58935777509570642, -68.58935777509452691, 8.000000000000000000 ) ) ;
#2331=CARTESIAN_POINT ( 'NONE',  ( -47.21331623427138879, -33.48561063518577896, -10.50000000000000000 ) ) ;
#2332=AXIS2_PLACEMENT_3D ( 'NONE', #3686, #7078, #12043 ) ;
#2333=VERTEX_POINT ( 'NONE', #10962 ) ;
#2334=DIRECTION ( 'NONE',  ( -1.000000000000000000, 0.000000000000000000, 0.000000000000000000 ) ) ;
#2335=VERTEX_POINT ( 'NONE', #8674 ) ;
#2337=DIRECTION ( 'NONE',  ( -0.000000000000000000, -0.000000000000000000, -1.000000000000000000 ) ) ;
#2338=ORIENTED_EDGE ( 'NONE', *, *, #9963, .T. ) ;
#2339=ORIENTED_EDGE ( 'NONE', *, *, #9758, .F. ) ;
#2341=AXIS2_PLACEMENT_3D ( 'NONE', #12626, #3296, #12555 ) ;
#2342=ORIENTED_EDGE ( 'NONE', *, *, #9893, .T. ) ;
#2343=CARTESIAN_POINT ( 'NONE',  ( -56.43380494354004639, -12.86891638962099549, 8.000000000000000000 ) ) ;
#2347=ORIENTED_EDGE ( 'NONE', *, *, #10554, .F. ) ;
#2348=DIRECTION ( 'NONE',  ( 1.000000000000000000, 0.000000000000000000, 0.000000000000000000 ) ) ;
#2349=ORIENTED_EDGE ( 'NONE', *, *, #3311, .T. ) ;
#2350=CARTESIAN_POINT ( 'NONE',  ( 22.33583958711425055, -30.74264578624780597, -28.00000000000000000 ) ) ;
#2351=EDGE_CURVE ( 'NONE', #3975, #13877, #10329, .T. ) ;
#2352=ORIENTED_EDGE ( 'NONE', *, *, #665, .F. ) ;
#2353=CYLINDRICAL_SURFACE ( 'NONE', #5700, 3.000000000000002665 ) ;
#2354=EDGE_CURVE ( 'NONE', #13011, #7502, #12529, .T. ) ;
#2355=ADVANCED_FACE ( 'NONE', ( #1917 ), #3074, .T. ) ;
#2357=DIRECTION ( 'NONE',  ( 0.000000000000000000, 0.000000000000000000, -1.000000000000000000 ) ) ;
#2360=CARTESIAN_POINT ( 'NONE',  ( 50.13108361037843252, 56.43380494353993271, -13.00000000000000178 ) ) ;
#2361=CARTESIAN_POINT ( 'NONE',  ( -32.39328945491989487, 42.64958156413685941, -10.50000000000000000 ) ) ;
#2363=DIRECTION ( 'NONE',  ( -1.000000000000000000, 0.000000000000000000, 0.000000000000000000 ) ) ;
#2366=DIRECTION ( 'NONE',  ( 0.000000000000000000, 0.000000000000000000, -1.000000000000000000 ) ) ;
#2369=CARTESIAN_POINT ( 'NONE',  ( 97.41488903138106537, -0.2790467552935826934, -13.00000000000000178 ) ) ;
#2371=DIRECTION ( 'NONE',  ( -1.000000000000000000, 0.000000000000000000, 0.000000000000000000 ) ) ;
#2372=DIRECTION ( 'NONE',  ( 0.000000000000000000, 0.000000000000000000, 1.000000000000000000 ) ) ;
#2373=ORIENTED_EDGE ( 'NONE', *, *, #9362, .T. ) ;
#2376=EDGE_CURVE ( 'NONE', #12171, #13551, #14692, .T. ) ;
#2377=CARTESIAN_POINT ( 'NONE',  ( -3.492805317593278058, 46.55633131742322917, -10.50000000000000000 ) ) ;
#2379=CARTESIAN_POINT ( 'NONE',  ( -9.706953719245875689, -57.06275842387046993, -10.50000000000000000 ) ) ;
#2381=VERTEX_POINT ( 'NONE', #12264 ) ;
#2382=DIRECTION ( 'NONE',  ( 0.000000000000000000, 0.000000000000000000, 1.000000000000000000 ) ) ;
#2383=AXIS2_PLACEMENT_3D ( 'NONE', #3577, #3347, #4715 ) ;
#2384=CARTESIAN_POINT ( 'NONE',  ( -36.14014761921588104, 11.74264578624790190, -28.00000000000000000 ) ) ;
#2386=ORIENTED_EDGE ( 'NONE', *, *, #1068, .T. ) ;
#2388=ADVANCED_FACE ( 'NONE', ( #6305 ), #7689, .F. ) ;
#2389=ORIENTED_EDGE ( 'NONE', *, *, #927, .T. ) ;
#2391=CYLINDRICAL_SURFACE ( 'NONE', #356, 56.99999999999999289 ) ;
#2392=CARTESIAN_POINT ( 'NONE',  ( -33.47282819776587814, 39.30189486418276346, -8.000000000000000000 ) ) ;
#2396=EDGE_LOOP ( 'NONE', ( #670, #11136, #10551, #12131, #4584, #8503, #11152, #3952, #10673, #5544, #622, #10463 ) ) ;
#2397=ORIENTED_EDGE ( 'NONE', *, *, #2260, .F. ) ;
#2398=EDGE_CURVE ( 'NONE', #6631, #9297, #8879, .T. ) ;
#2399=LINE ( 'NONE', #10383, #849 ) ;
#2401=LINE ( 'NONE', #4836, #6001 ) ;
#2402=EDGE_LOOP ( 'NONE', ( #501, #12886, #10318, #9422, #14673, #9848 ) ) ;
#2403=ORIENTED_EDGE ( 'NONE', *, *, #7165, .T. ) ;
#2404=CARTESIAN_POINT ( 'NONE',  ( 0.000000000000000000, 0.000000000000000000, 8.000000000000000000 ) ) ;
#2406=VERTEX_POINT ( 'NONE', #4293 ) ;
#2407=EDGE_CURVE ( 'NONE', #6515, #3692, #13012, .T. ) ;
#2408=CARTESIAN_POINT ( 'NONE',  ( 6.917888187663118416, 52.54657765281190507, -10.50000000000000000 ) ) ;
#2409=AXIS2_PLACEMENT_3D ( 'NONE', #8803, #5540, #10162 ) ;
#2411=DIRECTION ( 'NONE',  ( 0.000000000000000000, 0.000000000000000000, 1.000000000000000000 ) ) ;
#2412=CARTESIAN_POINT ( 'NONE',  ( 0.000000000000000000, 0.000000000000000000, -10.50000000000000000 ) ) ;
#2413=ORIENTED_EDGE ( 'NONE', *, *, #9779, .T. ) ;
#2418=AXIS2_PLACEMENT_3D ( 'NONE', #10696, #13057, #7265 ) ;
#2419=EDGE_LOOP ( 'NONE', ( #12280, #10828, #7764, #1399, #5103, #7846 ) ) ;
#2420=CIRCLE ( 'NONE', #3394, 59.50000000000000000 ) ;
#2421=AXIS2_PLACEMENT_3D ( 'NONE', #4056, #2684, #3904 ) ;
#2423=ORIENTED_EDGE ( 'NONE', *, *, #11476, .T. ) ;
#2424=DIRECTION ( 'NONE',  ( 0.000000000000000000, 0.000000000000000000, 1.000000000000000000 ) ) ;
#2425=DIRECTION ( 'NONE',  ( -0.000000000000000000, -0.000000000000000000, -1.000000000000000000 ) ) ;
#2426=CARTESIAN_POINT ( 'NONE',  ( 43.30127018922200932, -24.99999999999987210, 8.000000000000000000 ) ) ;
#2427=CIRCLE ( 'NONE', #8487, 59.50000000000000000 ) ;
#2428=LINE ( 'NONE', #6912, #2307 ) ;
#2429=CARTESIAN_POINT ( 'NONE',  ( 89.61631465359468507, -37.12029293941410657, -8.000000000000000000 ) ) ;
#2430=CARTESIAN_POINT ( 'NONE',  ( 42.50536573064410106, 32.06294366074510549, -10.50000000000000000 ) ) ;
#2431=AXIS2_PLACEMENT_3D ( 'NONE', #5590, #7498, #969 ) ;
#2432=CARTESIAN_POINT ( 'NONE',  ( 9.706953719245472456, 57.06275842387054098, -13.00000000000000178 ) ) ;
#2433=CIRCLE ( 'NONE', #2383, 100.0000000000000000 ) ;
#2435=EDGE_CURVE ( 'NONE', #2645, #3692, #645, .T. ) ;
#2437=EDGE_CURVE ( 'NONE', #2144, #7876, #662, .T. ) ;
#2438=ORIENTED_EDGE ( 'NONE', *, *, #8804, .T. ) ;
#2439=AXIS2_PLACEMENT_3D ( 'NONE', #851, #13368, #9025 ) ;
#2441=DIRECTION ( 'NONE',  ( 1.000000000000000000, 0.000000000000000000, 0.000000000000000000 ) ) ;
#2442=CIRCLE ( 'NONE', #10928, 63.00000000000000000 ) ;
#2443=DIRECTION ( 'NONE',  ( -1.000000000000000000, 0.000000000000000000, 0.000000000000000000 ) ) ;
#2446=CIRCLE ( 'NONE', #9956, 3.000000000000002665 ) ;
#2448=FACE_OUTER_BOUND ( 'NONE', #10438, .T. ) ;
#2449=ORIENTED_EDGE ( 'NONE', *, *, #9032, .T. ) ;
#2454=CIRCLE ( 'NONE', #10942, 56.99999999999999289 ) ;
#2455=CARTESIAN_POINT ( 'NONE',  ( -37.12029293941441210, -89.61631465359452875, 10.49999999999999822 ) ) ;
#2456=CARTESIAN_POINT ( 'NONE',  ( 37.12029293941315444, -89.61631465359504034, -10.50000000000000000 ) ) ;
#2458=ORIENTED_EDGE ( 'NONE', *, *, #348, .T. ) ;
#2460=DIRECTION ( 'NONE',  ( 0.000000000000000000, 0.000000000000000000, 1.000000000000000000 ) ) ;
#2462=DIRECTION ( 'NONE',  ( 0.000000000000000000, 0.000000000000000000, -1.000000000000000000 ) ) ;
#2465=ORIENTED_EDGE ( 'NONE', *, *, #4969, .F. ) ;
#2466=ORIENTED_EDGE ( 'NONE', *, *, #7180, .T. ) ;
#2467=AXIS2_PLACEMENT_3D ( 'NONE', #12899, #5352, #12342 ) ;
#2470=DIRECTION ( 'NONE',  ( -0.000000000000000000, -0.000000000000000000, -1.000000000000000000 ) ) ;
#2471=LINE ( 'NONE', #195, #144 ) ;
#2472=EDGE_LOOP ( 'NONE', ( #3725, #1496, #13388, #10133, #12962, #13056 ) ) ;
#2475=CIRCLE ( 'NONE', #9735, 2.649999999999992806 ) ;
#2476=ORIENTED_EDGE ( 'NONE', *, *, #9352, .F. ) ;
#2477=ADVANCED_FACE ( 'NONE', ( #6842 ), #8066, .F. ) ;
#2478=DIRECTION ( 'NONE',  ( -0.000000000000000000, -0.000000000000000000, -1.000000000000000000 ) ) ;
#2479=CARTESIAN_POINT ( 'NONE',  ( 39.66766701456160860, 30.43807145043623308, 8.000000000000000000 ) ) ;
#2480=EDGE_CURVE ( 'NONE', #203, #964, #4296, .T. ) ;
#2482=CIRCLE ( 'NONE', #6103, 50.00000000000000000 ) ;
#2483=LINE ( 'NONE', #6591, #1063 ) ;
#2484=ORIENTED_EDGE ( 'NONE', *, *, #2501, .T. ) ;
#2485=ORIENTED_EDGE ( 'NONE', *, *, #9718, .F. ) ;
#2486=CARTESIAN_POINT ( 'NONE',  ( 33.48561063518626923, -47.21331623427104063, -10.50000000000000000 ) ) ;
#2487=ORIENTED_EDGE ( 'NONE', *, *, #2319, .F. ) ;
#2488=AXIS2_PLACEMENT_3D ( 'NONE', #14362, #13009, #8440 ) ;
#2489=DIRECTION ( 'NONE',  ( 1.000000000000000000, 0.000000000000000000, 0.000000000000000000 ) ) ;
#2495=AXIS2_PLACEMENT_3D ( 'NONE', #10665, #6110, #14629 ) ;
#2496=CARTESIAN_POINT ( 'NONE',  ( -13.35619814848797837, 51.53979475227131246, 10.49999999999999822 ) ) ;
#2499=CARTESIAN_POINT ( 'NONE',  ( 22.33583958711425055, -30.74264578624780597, -25.50000000000000355 ) ) ;
#2501=EDGE_CURVE ( 'NONE', #7516, #132, #13264, .T. ) ;
#2504=AXIS2_PLACEMENT_3D ( 'NONE', #8156, #1114, #13863 ) ;
#2505=CARTESIAN_POINT ( 'NONE',  ( -68.09867107463028901, -68.49330278050098286, -13.00000000000000178 ) ) ;
#2510=VERTEX_POINT ( 'NONE', #13849 ) ;
#2511=DIRECTION ( 'NONE',  ( -0.000000000000000000, -0.000000000000000000, 1.000000000000000000 ) ) ;
#2512=DIRECTION ( 'NONE',  ( 0.000000000000000000, 0.000000000000000000, -1.000000000000000000 ) ) ;
#2515=AXIS2_PLACEMENT_3D ( 'NONE', #4504, #13763, #6908 ) ;
#2516=CARTESIAN_POINT ( 'NONE',  ( -53.26842454702436669, -11.55014193876159645, 8.000000000000000000 ) ) ;
#2518=VERTEX_POINT ( 'NONE', #13695 ) ;
#2522=DIRECTION ( 'NONE',  ( -0.000000000000000000, -0.000000000000000000, 1.000000000000000000 ) ) ;
#2523=ORIENTED_EDGE ( 'NONE', *, *, #12524, .F. ) ;
#2525=ADVANCED_FACE ( 'NONE', ( #12702 ), #11344, .T. ) ;
#2526=AXIS2_PLACEMENT_3D ( 'NONE', #4425, #5843, #78 ) ;
#2527=CIRCLE ( 'NONE', #13444, 0.5000000000000004441 ) ;
#2529=CIRCLE ( 'NONE', #594, 46.33974596215558961 ) ;
#2531=CARTESIAN_POINT ( 'NONE',  ( 0.000000000000000000, 0.000000000000000000, -8.000000000000000000 ) ) ;
#2532=DIRECTION ( 'NONE',  ( 0.000000000000000000, 0.000000000000000000, 1.000000000000000000 ) ) ;
#2533=DIRECTION ( 'NONE',  ( 0.000000000000000000, 0.000000000000000000, 1.000000000000000000 ) ) ;
#2534=DIRECTION ( 'NONE',  ( 0.000000000000000000, 0.000000000000000000, 1.000000000000000000 ) ) ;
#2535=CIRCLE ( 'NONE', #5687, 3.000000000000002665 ) ;
#2536=ORIENTED_EDGE ( 'NONE', *, *, #9431, .T. ) ;
#2537=ORIENTED_EDGE ( 'NONE', *, *, #3799, .T. ) ;
#2538=AXIS2_PLACEMENT_3D ( 'NONE', #5505, #11432, #4302 ) ;
#2541=CARTESIAN_POINT ( 'NONE',  ( -89.33979373934396051, 36.70371619500605220, -13.00000000000000178 ) ) ;
#2542=CIRCLE ( 'NONE', #8844, 3.000000000000004441 ) ;
#2546=VERTEX_POINT ( 'NONE', #4579 ) ;
#2547=EDGE_CURVE ( 'NONE', #9310, #8180, #6208, .T. ) ;
#2548=EDGE_CURVE ( 'NONE', #13523, #6561, #6695, .T. ) ;
#2549=CIRCLE ( 'NONE', #12995, 52.50000000000000711 ) ;
#2550=ORIENTED_EDGE ( 'NONE', *, *, #1572, .F. ) ;
#2555=FACE_OUTER_BOUND ( 'NONE', #13595, .T. ) ;
#2557=DIRECTION ( 'NONE',  ( 1.000000000000000000, 0.000000000000000000, 0.000000000000000000 ) ) ;
#2558=EDGE_LOOP ( 'NONE', ( #13037, #3073, #1632, #13708 ) ) ;
#2559=EDGE_LOOP ( 'NONE', ( #11028, #2465, #5405, #2682, #6596 ) ) ;
#2560=AXIS2_PLACEMENT_3D ( 'NONE', #13328, #5513, #4380 ) ;
#2561=DIRECTION ( 'NONE',  ( 0.000000000000000000, 0.000000000000000000, -1.000000000000000000 ) ) ;
#2565=VERTEX_POINT ( 'NONE', #11503 ) ;
#2566=VERTEX_POINT ( 'NONE', #5495 ) ;
#2567=DIRECTION ( 'NONE',  ( 1.000000000000000000, 0.000000000000000000, 0.000000000000000000 ) ) ;
#2570=CARTESIAN_POINT ( 'NONE',  ( -12.86891638962156215, 56.43380494353993271, -13.00000000000000178 ) ) ;
#2575=DIRECTION ( 'NONE',  ( 0.000000000000000000, 0.000000000000000000, 1.000000000000000000 ) ) ;
#2576=EDGE_CURVE ( 'NONE', #4454, #1517, #13993, .T. ) ;
#2577=ORIENTED_EDGE ( 'NONE', *, *, #10702, .F. ) ;
#2578=DIRECTION ( 'NONE',  ( 0.000000000000000000, 0.000000000000000000, 1.000000000000000000 ) ) ;
#2579=AXIS2_PLACEMENT_3D ( 'NONE', #1536, #1236, #14219 ) ;
#2580=ORIENTED_EDGE ( 'NONE', *, *, #11505, .T. ) ;
#2581=EDGE_LOOP ( 'NONE', ( #13598, #11519, #2403, #12666 ) ) ;
#2582=CARTESIAN_POINT ( 'NONE',  ( 39.61975340586555916, 91.27544013909752607, 8.000000000000000000 ) ) ;
#2583=ORIENTED_EDGE ( 'NONE', *, *, #1875, .F. ) ;
#2586=EDGE_CURVE ( 'NONE', #1338, #9298, #8638, .T. ) ;
#2589=CYLINDRICAL_SURFACE ( 'NONE', #13842, 3.000000000000002665 ) ;
#2590=DIRECTION ( 'NONE',  ( -0.000000000000000000, -0.000000000000000000, -1.000000000000000000 ) ) ;
#2591=VECTOR ( 'NONE', #8974, 1000.000000000000000 ) ;
#2593=DIRECTION ( 'NONE',  ( 1.000000000000000000, 0.000000000000000000, 0.000000000000000000 ) ) ;
#2595=DIRECTION ( 'NONE',  ( 0.000000000000000000, 0.000000000000000000, -1.000000000000000000 ) ) ;
#2596=EDGE_LOOP ( 'NONE', ( #6203, #15002, #8892, #8727, #10518 ) ) ;
#2597=EDGE_CURVE ( 'NONE', #12895, #1468, #14761, .T. ) ;
#2598=CARTESIAN_POINT ( 'NONE',  ( -26.24999999999972289, -45.46633369868319363, -10.50000000000000000 ) ) ;
#2599=DIRECTION ( 'NONE',  ( 1.000000000000000000, 0.000000000000000000, 0.000000000000000000 ) ) ;
#2603=CARTESIAN_POINT ( 'NONE',  ( 30.80502811811196295, 49.00442420936003174, -8.000000000000000000 ) ) ;
#2604=EDGE_LOOP ( 'NONE', ( #13206, #10127, #419, #9359 ) ) ;
#2605=EDGE_CURVE ( 'NONE', #14446, #14518, #13610, .T. ) ;
#2606=EDGE_LOOP ( 'NONE', ( #6975, #3081, #3763, #4083, #1138 ) ) ;
#2608=DIRECTION ( 'NONE',  ( 0.000000000000000000, 0.000000000000000000, 1.000000000000000000 ) ) ;
#2610=CARTESIAN_POINT ( 'NONE',  ( 0.000000000000000000, 0.000000000000000000, 8.000000000000000000 ) ) ;
#2612=ORIENTED_EDGE ( 'NONE', *, *, #12954, .F. ) ;
#2613=DIRECTION ( 'NONE',  ( -0.000000000000000000, -0.000000000000000000, 1.000000000000000000 ) ) ;
#2614=FACE_OUTER_BOUND ( 'NONE', #10775, .T. ) ;
#2616=CARTESIAN_POINT ( 'NONE',  ( 52.36539807335608288, -6.451868917687384020, 10.49999999999999822 ) ) ;
#2620=DIRECTION ( 'NONE',  ( 0.000000000000000000, 0.000000000000000000, 1.000000000000000000 ) ) ;
#2622=CYLINDRICAL_SURFACE ( 'NONE', #3768, 100.0000000000000000 ) ;
#2625=DIRECTION ( 'NONE',  ( 1.000000000000000000, 0.000000000000000000, 0.000000000000000000 ) ) ;
#2626=EDGE_CURVE ( 'NONE', #13011, #5657, #13755, .T. ) ;
#2629=EDGE_CURVE ( 'NONE', #11371, #9152, #11813, .T. ) ;
#2630=ORIENTED_EDGE ( 'NONE', *, *, #7350, .F. ) ;
#2631=EDGE_CURVE ( 'NONE', #2565, #5824, #3563, .T. ) ;
#2632=CARTESIAN_POINT ( 'NONE',  ( 68.58935777509475429, -68.58935777509547904, 8.000000000000000000 ) ) ;
#2633=CARTESIAN_POINT ( 'NONE',  ( -32.26435573746199736, 42.04772703543562073, -10.50000000000000000 ) ) ;
#2634=DIRECTION ( 'NONE',  ( 1.000000000000000000, 0.000000000000000000, 0.000000000000000000 ) ) ;
#2636=EDGE_LOOP ( 'NONE', ( #5047, #14707, #8436, #12121 ) ) ;
#2638=ADVANCED_FACE ( 'NONE', ( #13075 ), #7366, .T. ) ;
#2639=ORIENTED_EDGE ( 'NONE', *, *, #4824, .T. ) ;
#2640=DIRECTION ( 'NONE',  ( -1.000000000000000000, 0.000000000000000000, 0.000000000000000000 ) ) ;
#2642=EDGE_CURVE ( 'NONE', #14343, #303, #14282, .T. ) ;
#2643=CARTESIAN_POINT ( 'NONE',  ( -0.2790467552932217599, 96.58511096861892042, 10.49999999999999822 ) ) ;
#2644=CIRCLE ( 'NONE', #11138, 100.0000000000000000 ) ;
#2645=VERTEX_POINT ( 'NONE', #7213 ) ;
#2646=DIRECTION ( 'NONE',  ( -1.000000000000000000, 0.000000000000000000, 0.000000000000000000 ) ) ;
#2649=EDGE_CURVE ( 'NONE', #12492, #2144, #4531, .T. ) ;
#2651=ORIENTED_EDGE ( 'NONE', *, *, #11048, .F. ) ;
#2653=ORIENTED_EDGE ( 'NONE', *, *, #8327, .T. ) ;
#2655=CIRCLE ( 'NONE', #5080, 63.00000000000000000 ) ;
#2656=CARTESIAN_POINT ( 'NONE',  ( 51.45950017607693638, -4.121772567811421872, -8.000000000000000000 ) ) ;
#2658=DIRECTION ( 'NONE',  ( -0.000000000000000000, -0.000000000000000000, 1.000000000000000000 ) ) ;
#2660=PLANE ( 'NONE',  #10425 ) ;
#2661=CIRCLE ( 'NONE', #10908, 53.55662432702593634 ) ;
#2662=CIRCLE ( 'NONE', #3404, 0.5000000000000004441 ) ;
#2663=CARTESIAN_POINT ( 'NONE',  ( 57.06275842387049835, -9.706953719245678514, -13.00000000000000178 ) ) ;
#2664=EDGE_LOOP ( 'NONE', ( #8695, #9215 ) ) ;
#2667=DIRECTION ( 'NONE',  ( 1.000000000000000000, 0.000000000000000000, 0.000000000000000000 ) ) ;
#2668=ORIENTED_EDGE ( 'NONE', *, *, #12523, .F. ) ;
#2669=AXIS2_PLACEMENT_3D ( 'NONE', #8499, #3815, #6216 ) ;
#2670=DIRECTION ( 'NONE',  ( 1.000000000000000000, 0.000000000000000000, 0.000000000000000000 ) ) ;
#2671=DIRECTION ( 'NONE',  ( 0.000000000000000000, 0.000000000000000000, 1.000000000000000000 ) ) ;
#2673=EDGE_CURVE ( 'NONE', #4759, #7919, #2103, .T. ) ;
#2676=CARTESIAN_POINT ( 'NONE',  ( -46.81487971942585347, 26.01305530232610863, -10.50000000000000000 ) ) ;
#2678=ORIENTED_EDGE ( 'NONE', *, *, #3984, .T. ) ;
#2679=CIRCLE ( 'NONE', #1465, 0.5000000000000004441 ) ;
#2682=ORIENTED_EDGE ( 'NONE', *, *, #8692, .F. ) ;
#2683=AXIS2_PLACEMENT_3D ( 'NONE', #2412, #10161, #14809 ) ;
#2684=DIRECTION ( 'NONE',  ( 0.000000000000000000, 0.000000000000000000, 1.000000000000000000 ) ) ;
#2685=DIRECTION ( 'NONE',  ( 1.000000000000000000, 0.000000000000000000, 0.000000000000000000 ) ) ;
#2686=EDGE_CURVE ( 'NONE', #9298, #4338, #10719, .T. ) ;
#2691=CARTESIAN_POINT ( 'NONE',  ( 9.706953719245472456, 57.06275842387054098, -10.50000000000000000 ) ) ;
#2692=CIRCLE ( 'NONE', #13364, 3.000000000000002665 ) ;
#2693=FACE_OUTER_BOUND ( 'NONE', #12286, .T. ) ;
#2695=CIRCLE ( 'NONE', #1731, 3.000000000000002665 ) ;
#2696=CARTESIAN_POINT ( 'NONE',  ( 65.64523757230274725, 68.01302780753375998, -13.00000000000000178 ) ) ;
#2699=ORIENTED_EDGE ( 'NONE', *, *, #2900, .T. ) ;
#2700=AXIS2_PLACEMENT_3D ( 'NONE', #5887, #15016, #14794 ) ;
#2701=CARTESIAN_POINT ( 'NONE',  ( 7.383907457638312799, 52.72775723226772726, -10.50000000000000000 ) ) ;
#2702=CIRCLE ( 'NONE', #11194, 60.50000000000000000 ) ;
#2703=DIRECTION ( 'NONE',  ( 1.000000000000000000, 1.003641614261141513E-13, 0.000000000000000000 ) ) ;
#2704=CIRCLE ( 'NONE', #14342, 60.50000000000000000 ) ;
#2705=DIRECTION ( 'NONE',  ( 0.000000000000000000, 0.000000000000000000, 1.000000000000000000 ) ) ;
#2709=ORIENTED_EDGE ( 'NONE', *, *, #10051, .F. ) ;
#2710=CARTESIAN_POINT ( 'NONE',  ( -24.98583958711379793, -30.74264578624812927, -25.50000000000000355 ) ) ;
#2711=DIRECTION ( 'NONE',  ( 0.000000000000000000, 0.000000000000000000, 1.000000000000000000 ) ) ;
#2712=AXIS2_PLACEMENT_3D ( 'NONE', #4211, #11418, #1016 ) ;
#2713=DIRECTION ( 'NONE',  ( 1.000000000000000000, 0.000000000000000000, 0.000000000000000000 ) ) ;
#2714=VERTEX_POINT ( 'NONE', #2598 ) ;
#2715=CIRCLE ( 'NONE', #13879, 63.00000000000000000 ) ;
#2716=ORIENTED_EDGE ( 'NONE', *, *, #12994, .F. ) ;
#2717=DIRECTION ( 'NONE',  ( -1.000000000000000000, 0.000000000000000000, 0.000000000000000000 ) ) ;
#2718=ORIENTED_EDGE ( 'NONE', *, *, #14425, .T. ) ;
#2719=ADVANCED_FACE ( 'NONE', ( #11798 ), #8289, .T. ) ;
#2721=EDGE_CURVE ( 'NONE', #10576, #14940, #14512, .T. ) ;
#2722=CIRCLE ( 'NONE', #14574, 3.000000000000002665 ) ;
#2723=CARTESIAN_POINT ( 'NONE',  ( 0.000000000000000000, 0.000000000000000000, -8.000000000000000000 ) ) ;
#2724=ORIENTED_EDGE ( 'NONE', *, *, #14365, .T. ) ;
#2725=DIRECTION ( 'NONE',  ( 0.000000000000000000, 0.000000000000000000, 1.000000000000000000 ) ) ;
#2726=DIRECTION ( 'NONE',  ( -1.000000000000000000, 0.000000000000000000, 0.000000000000000000 ) ) ;
#2729=CYLINDRICAL_SURFACE ( 'NONE', #11396, 0.5000000000000022204 ) ;
#2732=VERTEX_POINT ( 'NONE', #12089 ) ;
#2733=CARTESIAN_POINT ( 'NONE',  ( 0.000000000000000000, 0.000000000000000000, -10.50000000000000000 ) ) ;
#2734=AXIS2_PLACEMENT_3D ( 'NONE', #11108, #11495, #2363 ) ;
#2735=ADVANCED_FACE ( 'NONE', ( #7507 ), #8881, .T. ) ;
#2737=DIRECTION ( 'NONE',  ( 0.000000000000000000, 0.000000000000000000, 1.000000000000000000 ) ) ;
#2738=CARTESIAN_POINT ( 'NONE',  ( 36.52608637591580987, -92.55687898036917716, 8.000000000000000000 ) ) ;
#2739=CARTESIAN_POINT ( 'NONE',  ( -89.61631465359519666, -37.12029293941281338, -13.00000000000000178 ) ) ;
#2740=DIRECTION ( 'NONE',  ( 0.000000000000000000, 0.000000000000000000, 1.000000000000000000 ) ) ;
#2742=AXIS2_PLACEMENT_3D ( 'NONE', #7838, #11050, #5199 ) ;
#2743=VERTEX_POINT ( 'NONE', #12164 ) ;
#2744=CARTESIAN_POINT ( 'NONE',  ( 50.00000000000000000, -6.123233995736766085E-15, -13.00000000000000178 ) ) ;
#2745=ORIENTED_EDGE ( 'NONE', *, *, #12331, .F. ) ;
#2746=DIRECTION ( 'NONE',  ( -0.000000000000000000, -0.000000000000000000, 1.000000000000000000 ) ) ;
#2747=DIRECTION ( 'NONE',  ( 0.000000000000000000, 0.000000000000000000, 1.000000000000000000 ) ) ;
#2748=CIRCLE ( 'NONE', #10742, 0.5000000000000004441 ) ;
#2749=DIRECTION ( 'NONE',  ( -0.000000000000000000, -0.000000000000000000, -1.000000000000000000 ) ) ;
#2750=CARTESIAN_POINT ( 'NONE',  ( 97.00000000000000000, -3.384287605079545030E-13, -13.00000000000000178 ) ) ;
#2752=VERTEX_POINT ( 'NONE', #3966 ) ;
#2755=ORIENTED_EDGE ( 'NONE', *, *, #2303, .T. ) ;
#2758=AXIS2_PLACEMENT_3D ( 'NONE', #1865, #4149, #3156 ) ;
#2760=EDGE_CURVE ( 'NONE', #5754, #9386, #14476, .T. ) ;
#2761=DIRECTION ( 'NONE',  ( 1.000000000000000000, 0.000000000000000000, 0.000000000000000000 ) ) ;
#2762=DIRECTION ( 'NONE',  ( 0.000000000000000000, 0.000000000000000000, 1.000000000000000000 ) ) ;
#2765=CARTESIAN_POINT ( 'NONE',  ( -42.04772703543551415, -32.26435573746212526, 10.49999999999999822 ) ) ;
#2768=DIRECTION ( 'NONE',  ( 0.000000000000000000, 0.000000000000000000, 1.000000000000000000 ) ) ;
#2771=EDGE_CURVE ( 'NONE', #5876, #3028, #11579, .T. ) ;
#2773=DIRECTION ( 'NONE',  ( -1.000000000000000000, 0.000000000000000000, 0.000000000000000000 ) ) ;
#2774=ORIENTED_EDGE ( 'NONE', *, *, #1522, .T. ) ;
#2775=DIRECTION ( 'NONE',  ( 0.000000000000000000, 0.000000000000000000, 1.000000000000000000 ) ) ;
#2776=ORIENTED_EDGE ( 'NONE', *, *, #1912, .F. ) ;
#2778=AXIS2_PLACEMENT_3D ( 'NONE', #9675, #8979, #13540 ) ;
#2779=CARTESIAN_POINT ( 'NONE',  ( 30.80502811811196295, 49.00442420936003174, 10.49999999999999822 ) ) ;
#2780=EDGE_CURVE ( 'NONE', #13864, #14119, #6287, .T. ) ;
#2783=DIRECTION ( 'NONE',  ( 0.000000000000000000, 0.000000000000000000, 1.000000000000000000 ) ) ;
#2785=AXIS2_PLACEMENT_3D ( 'NONE', #1842, #1770, #6457 ) ;
#2787=ORIENTED_EDGE ( 'NONE', *, *, #3434, .T. ) ;
#2788=CARTESIAN_POINT ( 'NONE',  ( 2.649999999999993250, 38.00000000000000000, -25.50000000000000355 ) ) ;
#2789=FACE_OUTER_BOUND ( 'NONE', #2606, .T. ) ;
#2791=DIRECTION ( 'NONE',  ( 0.000000000000000000, 0.000000000000000000, -1.000000000000000000 ) ) ;
#2793=EDGE_CURVE ( 'NONE', #7980, #2928, #8411, .T. ) ;
#2794=CIRCLE ( 'NONE', #6895, 59.50000000000000000 ) ;
#2795=ORIENTED_EDGE ( 'NONE', *, *, #937, .F. ) ;
#2796=FACE_OUTER_BOUND ( 'NONE', #3840, .T. ) ;
#2797=VECTOR ( 'NONE', #1640, 1000.000000000000000 ) ;
#2798=AXIS2_PLACEMENT_3D ( 'NONE', #8975, #14838, #2146 ) ;
#2800=ORIENTED_EDGE ( 'NONE', *, *, #8886, .F. ) ;
#2801=DIRECTION ( 'NONE',  ( 0.000000000000000000, 0.000000000000000000, -1.000000000000000000 ) ) ;
#2805=DIRECTION ( 'NONE',  ( 1.000000000000000000, 0.000000000000000000, 0.000000000000000000 ) ) ;
#2806=ORIENTED_EDGE ( 'NONE', *, *, #11216, .T. ) ;
#2807=DIRECTION ( 'NONE',  ( 1.000000000000000000, 0.000000000000000000, -0.000000000000000000 ) ) ;
#2808=ORIENTED_EDGE ( 'NONE', *, *, #1188, .F. ) ;
#2809=EDGE_LOOP ( 'NONE', ( #10413, #11835, #10660, #13459 ) ) ;
#2811=VECTOR ( 'NONE', #1270, 1000.000000000000000 ) ;
#2812=CIRCLE ( 'NONE', #14699, 63.00000000000000000 ) ;
#2813=DIRECTION ( 'NONE',  ( 1.000000000000000000, 0.000000000000000000, 0.000000000000000000 ) ) ;
#2814=DIRECTION ( 'NONE',  ( 0.000000000000000000, 0.000000000000000000, -1.000000000000000000 ) ) ;
#2815=CARTESIAN_POINT ( 'NONE',  ( 89.61631465359468507, -37.12029293941410657, -8.000000000000000000 ) ) ;
#2816=DIRECTION ( 'NONE',  ( 1.000000000000000000, 0.000000000000000000, 0.000000000000000000 ) ) ;
#2818=ORIENTED_EDGE ( 'NONE', *, *, #13128, .T. ) ;
#2819=AXIS2_PLACEMENT_3D ( 'NONE', #11738, #4900, #10877 ) ;
#2820=EDGE_CURVE ( 'NONE', #5837, #8250, #8579, .T. ) ;
#2821=DIRECTION ( 'NONE',  ( 0.000000000000000000, 0.000000000000000000, 1.000000000000000000 ) ) ;
#2822=ORIENTED_EDGE ( 'NONE', *, *, #11520, .F. ) ;
#2823=EDGE_CURVE ( 'NONE', #12895, #14306, #5740, .T. ) ;
#2824=EDGE_CURVE ( 'NONE', #3692, #13772, #6454, .T. ) ;
#2825=EDGE_CURVE ( 'NONE', #5327, #198, #1867, .T. ) ;
#2826=DIRECTION ( 'NONE',  ( 1.000000000000000000, 0.000000000000000000, 0.000000000000000000 ) ) ;
#2827=DIRECTION ( 'NONE',  ( 0.000000000000000000, 0.000000000000000000, 1.000000000000000000 ) ) ;
#2828=EDGE_LOOP ( 'NONE', ( #12358, #11033, #10938, #1048 ) ) ;
#2830=EDGE_CURVE ( 'NONE', #303, #2935, #3816, .T. ) ;
#2832=ORIENTED_EDGE ( 'NONE', *, *, #4781, .T. ) ;
#2833=AXIS2_PLACEMENT_3D ( 'NONE', #8438, #11719, #1393 ) ;
#2834=DIRECTION ( 'NONE',  ( -1.000000000000000000, 0.000000000000000000, 0.000000000000000000 ) ) ;
#2836=CARTESIAN_POINT ( 'NONE',  ( 0.000000000000000000, 0.000000000000000000, 13.00000000000000178 ) ) ;
#2837=DIRECTION ( 'NONE',  ( -1.000000000000000000, 0.000000000000000000, 0.000000000000000000 ) ) ;
#2838=CARTESIAN_POINT ( 'NONE',  ( 36.14014761921570340, 11.74264578624841171, -25.50000000000000355 ) ) ;
#2840=DIRECTION ( 'NONE',  ( -0.000000000000000000, -0.000000000000000000, 1.000000000000000000 ) ) ;
#2841=ORIENTED_EDGE ( 'NONE', *, *, #13537, .F. ) ;
#2844=CARTESIAN_POINT ( 'NONE',  ( 32.26435573746228158, -42.04772703543541468, -8.000000000000000000 ) ) ;
#2845=EDGE_CURVE ( 'NONE', #11326, #2743, #13668, .T. ) ;
#2846=ORIENTED_EDGE ( 'NONE', *, *, #7882, .F. ) ;
#2848=ORIENTED_EDGE ( 'NONE', *, *, #12480, .F. ) ;
#2849=DIRECTION ( 'NONE',  ( 1.000000000000000000, 0.000000000000000000, 0.000000000000000000 ) ) ;
#2851=CARTESIAN_POINT ( 'NONE',  ( 51.53979475227119167, 13.35619814848851483, 10.49999999999999822 ) ) ;
#2857=CARTESIAN_POINT ( 'NONE',  ( -13.21740939043329099, 51.19406879332069593, -10.50000000000000000 ) ) ;
#2858=DIRECTION ( 'NONE',  ( 1.000000000000000000, 0.000000000000000000, -0.000000000000000000 ) ) ;
#2860=ORIENTED_EDGE ( 'NONE', *, *, #2824, .F. ) ;
#2863=ORIENTED_EDGE ( 'NONE', *, *, #8614, .F. ) ;
#2864=FACE_OUTER_BOUND ( 'NONE', #10048, .T. ) ;
#2865=ORIENTED_EDGE ( 'NONE', *, *, #8873, .T. ) ;
#2866=CARTESIAN_POINT ( 'NONE',  ( -48.19406879332065330, -13.71740939043347041, 8.000000000000000000 ) ) ;
#2870=CARTESIAN_POINT ( 'NONE',  ( -97.41488903138106537, 0.2790467552942557661, 10.49999999999999822 ) ) ;
#2872=EDGE_LOOP ( 'NONE', ( #10619, #5353, #8191, #11115, #887 ) ) ;
#2873=CYLINDRICAL_SURFACE ( 'NONE', #10654, 3.000000000000002665 ) ;
#2874=ORIENTED_EDGE ( 'NONE', *, *, #2780, .T. ) ;
#2876=VERTEX_POINT ( 'NONE', #11759 ) ;
#2877=DIRECTION ( 'NONE',  ( -1.000000000000000000, 0.000000000000000000, 0.000000000000000000 ) ) ;
#2878=VERTEX_POINT ( 'NONE', #7896 ) ;
#2880=CARTESIAN_POINT ( 'NONE',  ( -45.88839665196098849, 26.99988008862674960, 10.49999999999999822 ) ) ;
#2881=CARTESIAN_POINT ( 'NONE',  ( 100.0000000000000000, -3.675178358715236078E-13, -8.000000000000000000 ) ) ;
#2884=ORIENTED_EDGE ( 'NONE', *, *, #14608, .T. ) ;
#2885=DIRECTION ( 'NONE',  ( -1.000000000000000000, 0.000000000000000000, 0.000000000000000000 ) ) ;
#2886=CARTESIAN_POINT ( 'NONE',  ( 9.917888187663120192, 52.54657765281190507, -13.00000000000000178 ) ) ;
#2890=ORIENTED_EDGE ( 'NONE', *, *, #10068, .T. ) ;
#2892=DIRECTION ( 'NONE',  ( 0.000000000000000000, 0.000000000000000000, -1.000000000000000000 ) ) ;
#2893=ORIENTED_EDGE ( 'NONE', *, *, #7180, .F. ) ;
#2896=ORIENTED_EDGE ( 'NONE', *, *, #3604, .T. ) ;
#2897=AXIS2_PLACEMENT_3D ( 'NONE', #8890, #11104, #936 ) ;
#2899=CARTESIAN_POINT ( 'NONE',  ( 0.000000000000000000, 0.000000000000000000, -8.000000000000000000 ) ) ;
#2900=EDGE_CURVE ( 'NONE', #5135, #12050, #13419, .T. ) ;
#2901=DIRECTION ( 'NONE',  ( 0.000000000000000000, 0.000000000000000000, 1.000000000000000000 ) ) ;
#2902=CIRCLE ( 'NONE', #4367, 100.0000000000000000 ) ;
#2904=CARTESIAN_POINT ( 'NONE',  ( 37.12029293941315444, -89.61631465359504034, -8.000000000000000000 ) ) ;
#2905=CIRCLE ( 'NONE', #2669, 0.5000000000000073275 ) ;
#2906=CARTESIAN_POINT ( 'NONE',  ( 69.08004447556065486, 68.68541276968852571, -10.50000000000000000 ) ) ;
#2907=DIRECTION ( 'NONE',  ( -0.000000000000000000, -0.000000000000000000, -1.000000000000000000 ) ) ;
#2908=VERTEX_POINT ( 'NONE', #10253 ) ;
#2909=ORIENTED_EDGE ( 'NONE', *, *, #13742, .F. ) ;
#2910=CARTESIAN_POINT ( 'NONE',  ( 0.000000000000000000, 0.000000000000000000, 13.00000000000000178 ) ) ;
#2912=VECTOR ( 'NONE', #8588, 1000.000000000000000 ) ;
#2913=CARTESIAN_POINT ( 'NONE',  ( 56.43380494353997534, 12.86891638962136319, -13.00000000000000178 ) ) ;
#2914=CIRCLE ( 'NONE', #11410, 53.55662432702593634 ) ;
#2919=DIRECTION ( 'NONE',  ( -1.000000000000000000, 0.000000000000000000, 0.000000000000000000 ) ) ;
#2920=VERTEX_POINT ( 'NONE', #1080 ) ;
#2921=DIRECTION ( 'NONE',  ( 0.000000000000000000, 0.000000000000000000, -1.000000000000000000 ) ) ;
#2925=LINE ( 'NONE', #5130, #3433 ) ;
#2928=VERTEX_POINT ( 'NONE', #11329 ) ;
#2930=ORIENTED_EDGE ( 'NONE', *, *, #8566, .T. ) ;
#2931=AXIS2_PLACEMENT_3D ( 'NONE', #13516, #12383, #11249 ) ;
#2932=CARTESIAN_POINT ( 'NONE',  ( -20.00000000000000000, 0.000000000000000000, -25.50000000000000355 ) ) ;
#2933=CARTESIAN_POINT ( 'NONE',  ( 2.449293598294700991E-16, -97.00000000000000000, 8.000000000000000000 ) ) ;
#2935=VERTEX_POINT ( 'NONE', #9456 ) ;
#2936=VECTOR ( 'NONE', #11554, 1000.000000000000000 ) ;
#2937=VERTEX_POINT ( 'NONE', #4498 ) ;
#2940=VERTEX_POINT ( 'NONE', #999 ) ;
#2941=AXIS2_PLACEMENT_3D ( 'NONE', #11472, #1070, #3264 ) ;
#2942=DIRECTION ( 'NONE',  ( 0.000000000000000000, 0.000000000000000000, 1.000000000000000000 ) ) ;
#2943=PLANE ( 'NONE',  #9783 ) ;
#2944=ADVANCED_FACE ( 'NONE', ( #928 ), #8249, .T. ) ;
#2947=CIRCLE ( 'NONE', #7291, 63.00000000000000000 ) ;
#2949=EDGE_CURVE ( 'NONE', #9901, #8073, #2483, .T. ) ;
#2950=ORIENTED_EDGE ( 'NONE', *, *, #13235, .T. ) ;
#2951=DIRECTION ( 'NONE',  ( 0.000000000000000000, 0.000000000000000000, 1.000000000000000000 ) ) ;
#2952=AXIS2_PLACEMENT_3D ( 'NONE', #7806, #6732, #13749 ) ;
#2953=ORIENTED_EDGE ( 'NONE', *, *, #5003, .T. ) ;
#2955=CARTESIAN_POINT ( 'NONE',  ( 57.06275842387049835, -9.706953719245678514, -8.000000000000000000 ) ) ;
#2956=EDGE_CURVE ( 'NONE', #12263, #218, #13657, .T. ) ;
#2957=CIRCLE ( 'NONE', #7553, 2.649999999999992806 ) ;
#2959=CIRCLE ( 'NONE', #1504, 0.5000000000000022204 ) ;
#2960=CARTESIAN_POINT ( 'NONE',  ( 0.000000000000000000, 0.000000000000000000, -8.000000000000000000 ) ) ;
#2962=LINE ( 'NONE', #5471, #238 ) ;
#2963=EDGE_CURVE ( 'NONE', #4159, #14486, #8561, .T. ) ;
#2964=CARTESIAN_POINT ( 'NONE',  ( 49.11971303961677648, 15.88467684210564990, -13.00000000000000178 ) ) ;
#2965=EDGE_CURVE ( 'NONE', #5889, #13141, #5478, .T. ) ;
#2966=EDGE_LOOP ( 'NONE', ( #5799, #12449, #1206, #70, #13723, #11353, #13169, #12816, #12321 ) ) ;
#2967=PLANE ( 'NONE',  #13594 ) ;
#2968=CARTESIAN_POINT ( 'NONE',  ( 11.55014193876178652, -53.26842454702432406, -13.00000000000000178 ) ) ;
#2969=AXIS2_PLACEMENT_3D ( 'NONE', #11740, #15008, #3381 ) ;
#2972=EDGE_LOOP ( 'NONE', ( #3556, #13703, #4163, #793 ) ) ;
#2973=AXIS2_PLACEMENT_3D ( 'NONE', #10729, #4894, #7152 ) ;
#2974=ORIENTED_EDGE ( 'NONE', *, *, #5280, .F. ) ;
#2975=FILL_AREA_STYLE_COLOUR ( '', #12262 ) ;
#2976=VERTEX_POINT ( 'NONE', #12607 ) ;
#2979=CARTESIAN_POINT ( 'NONE',  ( -51.19406879332065330, -13.71740939043347041, -10.50000000000000000 ) ) ;
#2980=ORIENTED_EDGE ( 'NONE', *, *, #14625, .F. ) ;
#2982=FACE_OUTER_BOUND ( 'NONE', #6132, .T. ) ;
#2983=LINE ( 'NONE', #7684, #10246 ) ;
#2984=DIRECTION ( 'NONE',  ( 1.000000000000000000, 0.000000000000000000, 0.000000000000000000 ) ) ;
#2985=CARTESIAN_POINT ( 'NONE',  ( -65.64523757230321621, -68.01302780753330524, -8.000000000000000000 ) ) ;
#2988=VERTEX_POINT ( 'NONE', #14817 ) ;
#2989=DIRECTION ( 'NONE',  ( 0.000000000000000000, 0.000000000000000000, -1.000000000000000000 ) ) ;
#2990=DIRECTION ( 'NONE',  ( 0.000000000000000000, 0.000000000000000000, 1.000000000000000000 ) ) ;
#2998=DIRECTION ( 'NONE',  ( 0.000000000000000000, 0.000000000000000000, 1.000000000000000000 ) ) ;
#2999=DIRECTION ( 'NONE',  ( -1.000000000000000000, 0.000000000000000000, 0.000000000000000000 ) ) ;
#3000=ORIENTED_EDGE ( 'NONE', *, *, #6467, .F. ) ;
#3004=ORIENTED_EDGE ( 'NONE', *, *, #11647, .T. ) ;
#3007=CIRCLE ( 'NONE', #10524, 0.5000000000000038858 ) ;
#3008=CARTESIAN_POINT ( 'NONE',  ( -52.54657765281192638, 6.917888187662934563, 8.000000000000000000 ) ) ;
#3009=CARTESIAN_POINT ( 'NONE',  ( -49.00442420935969778, 30.80502811811250297, -10.50000000000000000 ) ) ;
#3010=CIRCLE ( 'NONE', #1558, 60.50000000000000711 ) ;
#3011=EDGE_CURVE ( 'NONE', #3028, #1282, #565, .T. ) ;
#3014=EDGE_CURVE ( 'NONE', #2149, #297, #432, .T. ) ;
#3016=ORIENTED_EDGE ( 'NONE', *, *, #12226, .F. ) ;
#3019=AXIS2_PLACEMENT_3D ( 'NONE', #12124, #431, #5286 ) ;
#3020=VECTOR ( 'NONE', #8405, 1000.000000000000000 ) ;
#3022=CARTESIAN_POINT ( 'NONE',  ( 7.417888187663120192, 52.54657765281190507, -10.50000000000000000 ) ) ;
#3024=AXIS2_PLACEMENT_3D ( 'NONE', #10373, #11675, #120 ) ;
#3025=CARTESIAN_POINT ( 'NONE',  ( 0.000000000000000000, 0.000000000000000000, -10.50000000000000000 ) ) ;
#3027=DIRECTION ( 'NONE',  ( 0.000000000000000000, 0.000000000000000000, 1.000000000000000000 ) ) ;
#3028=VERTEX_POINT ( 'NONE', #1502 ) ;
#3029=ORIENTED_EDGE ( 'NONE', *, *, #12983, .T. ) ;
#3030=LINE ( 'NONE', #4174, #7783 ) ;
#3034=AXIS2_PLACEMENT_3D ( 'NONE', #8253, #14185, #10462 ) ;
#3036=CIRCLE ( 'NONE', #11536, 20.00000000000000000 ) ;
#3037=ORIENTED_EDGE ( 'NONE', *, *, #1665, .F. ) ;
#3039=VERTEX_POINT ( 'NONE', #585 ) ;
#3041=EDGE_CURVE ( 'NONE', #8922, #915, #11492, .T. ) ;
#3042=FACE_OUTER_BOUND ( 'NONE', #3496, .T. ) ;
#3047=DIRECTION ( 'NONE',  ( 1.000000000000000000, 0.000000000000000000, 0.000000000000000000 ) ) ;
#3048=CIRCLE ( 'NONE', #2798, 3.000000000000002665 ) ;
#3049=CIRCLE ( 'NONE', #5223, 60.50000000000000000 ) ;
#3050=DIRECTION ( 'NONE',  ( 1.000000000000000000, 0.000000000000000000, 0.000000000000000000 ) ) ;
#3051=ORIENTED_EDGE ( 'NONE', *, *, #6748, .T. ) ;
#3052=DIRECTION ( 'NONE',  ( -1.000000000000000000, 0.000000000000000000, -0.000000000000000000 ) ) ;
#3053=AXIS2_PLACEMENT_3D ( 'NONE', #13485, #12283, #1869 ) ;
#3056=AXIS2_PLACEMENT_3D ( 'NONE', #3873, #11708, #8492 ) ;
#3058=( LENGTH_UNIT ( ) NAMED_UNIT ( * ) SI_UNIT ( .MILLI., .METRE. ) );
#3059=ADVANCED_FACE ( 'NONE', ( #5217 ), #7412, .T. ) ;
#3061=EDGE_CURVE ( 'NONE', #12145, #6775, #5658, .T. ) ;
#3062=VERTEX_POINT ( 'NONE', #14254 ) ;
#3063=DIRECTION ( 'NONE',  ( 0.000000000000000000, 0.000000000000000000, 1.000000000000000000 ) ) ;
#3064=ORIENTED_EDGE ( 'NONE', *, *, #8857, .F. ) ;
#3065=ORIENTED_EDGE ( 'NONE', *, *, #12364, .F. ) ;
#3067=DIRECTION ( 'NONE',  ( 0.000000000000000000, 0.000000000000000000, -1.000000000000000000 ) ) ;
#3069=CIRCLE ( 'NONE', #9111, 100.0000000000000000 ) ;
#3071=CYLINDRICAL_SURFACE ( 'NONE', #14400, 3.000000000000002665 ) ;
#3072=EDGE_CURVE ( 'NONE', #9656, #6859, #4940, .T. ) ;
#3073=ORIENTED_EDGE ( 'NONE', *, *, #3109, .T. ) ;
#3074=CYLINDRICAL_SURFACE ( 'NONE', #1609, 3.000000000000002665 ) ;
#3075=DIRECTION ( 'NONE',  ( 0.000000000000000000, 0.000000000000000000, -1.000000000000000000 ) ) ;
#3076=CARTESIAN_POINT ( 'NONE',  ( 0.000000000000000000, 0.000000000000000000, 8.000000000000000000 ) ) ;
#3079=ORIENTED_EDGE ( 'NONE', *, *, #6464, .T. ) ;
#3081=ORIENTED_EDGE ( 'NONE', *, *, #11550, .T. ) ;
#3082=FACE_OUTER_BOUND ( 'NONE', #11334, .T. ) ;
#3083=DIRECTION ( 'NONE',  ( 1.000000000000000000, 0.000000000000000000, 0.000000000000000000 ) ) ;
#3084=ORIENTED_EDGE ( 'NONE', *, *, #6039, .T. ) ;
#3085=CARTESIAN_POINT ( 'NONE',  ( 0.000000000000000000, 0.000000000000000000, 8.000000000000000000 ) ) ;
#3086=CARTESIAN_POINT ( 'NONE',  ( -100.0000000000000000, 0.000000000000000000, -13.00000000000000178 ) ) ;
#3088=ORIENTED_EDGE ( 'NONE', *, *, #7200, .T. ) ;
#3089=ORIENTED_EDGE ( 'NONE', *, *, #7585, .F. ) ;
#3090=DIRECTION ( 'NONE',  ( 1.000000000000000000, 0.000000000000000000, 0.000000000000000000 ) ) ;
#3092=LINE ( 'NONE', #9906, #9049 ) ;
#3094=EDGE_LOOP ( 'NONE', ( #14388, #3409, #5176, #2342, #13518 ) ) ;
#3098=EDGE_CURVE ( 'NONE', #4822, #13864, #14877, .T. ) ;
#3099=DIRECTION ( 'NONE',  ( 1.000000000000000000, 0.000000000000000000, -0.000000000000000000 ) ) ;
#3100=EDGE_CURVE ( 'NONE', #14147, #13178, #11832, .T. ) ;
#3103=CARTESIAN_POINT ( 'NONE',  ( 92.61631465359491244, 37.12029293941346708, 8.000000000000000000 ) ) ;
#3105=EDGE_LOOP ( 'NONE', ( #1584, #2884, #7100, #9089, #538, #15005, #13987 ) ) ;
#3106=CARTESIAN_POINT ( 'NONE',  ( 0.000000000000000000, 0.000000000000000000, -10.50000000000000000 ) ) ;
#3108=ORIENTED_EDGE ( 'NONE', *, *, #9123, .F. ) ;
#3109=EDGE_CURVE ( 'NONE', #6283, #8922, #4924, .T. ) ;
#3110=ORIENTED_EDGE ( 'NONE', *, *, #7123, .F. ) ;
#3112=EDGE_CURVE ( 'NONE', #2908, #12963, #13194, .T. ) ;
#3113=FACE_OUTER_BOUND ( 'NONE', #13889, .T. ) ;
#3114=DIRECTION ( 'NONE',  ( -0.000000000000000000, -0.000000000000000000, 1.000000000000000000 ) ) ;
#3115=DIRECTION ( 'NONE',  ( 0.000000000000000000, 0.000000000000000000, 1.000000000000000000 ) ) ;
#3116=ADVANCED_FACE ( 'NONE', ( #5141 ), #6329, .T. ) ;
#3117=EDGE_LOOP ( 'NONE', ( #2270, #1534, #3064, #9365 ) ) ;
#3120=VECTOR ( 'NONE', #9182, 1000.000000000000000 ) ;
#3121=DIRECTION ( 'NONE',  ( 0.000000000000000000, 0.000000000000000000, -1.000000000000000000 ) ) ;
#3123=DIRECTION ( 'NONE',  ( 0.000000000000000000, 0.000000000000000000, 1.000000000000000000 ) ) ;
#3124=ORIENTED_EDGE ( 'NONE', *, *, #6862, .F. ) ;
#3125=CARTESIAN_POINT ( 'NONE',  ( 55.00000000000000000, -6.735557395310442615E-15, -13.00000000000000178 ) ) ;
#3129=CARTESIAN_POINT ( 'NONE',  ( 46.63108361037843252, 56.43380494353993271, -10.50000000000000000 ) ) ;
#3130=DIRECTION ( 'NONE',  ( 1.000000000000000000, 0.000000000000000000, 0.000000000000000000 ) ) ;
#3132=CARTESIAN_POINT ( 'NONE',  ( 47.21331623427115431, 33.48561063518610581, 10.49999999999999822 ) ) ;
#3134=FACE_OUTER_BOUND ( 'NONE', #12510, .T. ) ;
#3135=DIRECTION ( 'NONE',  ( -0.000000000000000000, -0.000000000000000000, -1.000000000000000000 ) ) ;
#3138=CARTESIAN_POINT ( 'NONE',  ( 97.00000000000000000, -3.384287605079545030E-13, 8.000000000000000000 ) ) ;
#3141=ADVANCED_FACE ( 'NONE', ( #8849 ), #10019, .F. ) ;
#3142=DIRECTION ( 'NONE',  ( 0.000000000000000000, 0.000000000000000000, 1.000000000000000000 ) ) ;
#3144=ADVANCED_FACE ( 'NONE', ( #14554 ), #7555, .T. ) ;
#3146=FACE_OUTER_BOUND ( 'NONE', #4655, .T. ) ;
#3147=ORIENTED_EDGE ( 'NONE', *, *, #14087, .T. ) ;
#3148=ADVANCED_FACE ( 'NONE', ( #899 ), #14636, .F. ) ;
#3151=ORIENTED_EDGE ( 'NONE', *, *, #11980, .F. ) ;
#3153=DIRECTION ( 'NONE',  ( 1.000000000000000000, 0.000000000000000000, 0.000000000000000000 ) ) ;
#3154=ORIENTED_EDGE ( 'NONE', *, *, #1066, .F. ) ;
#3156=DIRECTION ( 'NONE',  ( 1.000000000000000000, 0.000000000000000000, 0.000000000000000000 ) ) ;
#3158=ORIENTED_EDGE ( 'NONE', *, *, #9090, .F. ) ;
#3159=CIRCLE ( 'NONE', #6761, 63.00000000000000000 ) ;
#3161=EDGE_CURVE ( 'NONE', #4530, #9110, #823, .T. ) ;
#3162=CIRCLE ( 'NONE', #5091, 59.49999999999999289 ) ;
#3166=DIRECTION ( 'NONE',  ( -1.000000000000000000, 0.000000000000000000, 0.000000000000000000 ) ) ;
#3169=ORIENTED_EDGE ( 'NONE', *, *, #5139, .F. ) ;
#3170=DIRECTION ( 'NONE',  ( 0.000000000000000000, 0.000000000000000000, -1.000000000000000000 ) ) ;
#3171=AXIS2_PLACEMENT_3D ( 'NONE', #1012, #4509, #2292 ) ;
#3172=AXIS2_PLACEMENT_3D ( 'NONE', #10688, #3720, #8340 ) ;
#3175=CARTESIAN_POINT ( 'NONE',  ( -0.2790467552932217599, 96.58511096861892042, -10.50000000000000000 ) ) ;
#3176=ORIENTED_EDGE ( 'NONE', *, *, #3014, .T. ) ;
#3177=DIRECTION ( 'NONE',  ( 1.000000000000000000, 0.000000000000000000, 0.000000000000000000 ) ) ;
#3178=DIRECTION ( 'NONE',  ( -1.000000000000000000, 0.000000000000000000, 0.000000000000000000 ) ) ;
#3180=AXIS2_PLACEMENT_3D ( 'NONE', #6148, #5250, #2667 ) ;
#3181=ORIENTED_EDGE ( 'NONE', *, *, #14610, .T. ) ;
#3183=AXIS2_PLACEMENT_3D ( 'NONE', #7484, #2725, #7342 ) ;
#3184=VERTEX_POINT ( 'NONE', #5365 ) ;
#3185=FACE_OUTER_BOUND ( 'NONE', #6867, .T. ) ;
#3186=EDGE_CURVE ( 'NONE', #14403, #9441, #7101, .T. ) ;
#3187=DIRECTION ( 'NONE',  ( 0.000000000000000000, 0.000000000000000000, 1.000000000000000000 ) ) ;
#3188=CARTESIAN_POINT ( 'NONE',  ( -90.10640870805754332, -37.02125851216322872, 10.49999999999999822 ) ) ;
#3189=CIRCLE ( 'NONE', #1737, 60.50000000000000000 ) ;
#3190=DIRECTION ( 'NONE',  ( 0.000000000000000000, 0.000000000000000000, 1.000000000000000000 ) ) ;
#3191=CARTESIAN_POINT ( 'NONE',  ( -24.98583958711379083, -30.74264578624812927, -28.00000000000000000 ) ) ;
#3192=LINE ( 'NONE', #9861, #11146 ) ;
#3194=ORIENTED_EDGE ( 'NONE', *, *, #4743, .F. ) ;
#3198=CIRCLE ( 'NONE', #3932, 3.000000000000002665 ) ;
#3199=VERTEX_POINT ( 'NONE', #6639 ) ;
#3201=EDGE_CURVE ( 'NONE', #13408, #2119, #12945, .T. ) ;
#3202=EDGE_CURVE ( 'NONE', #13490, #4514, #3092, .T. ) ;
#3203=EDGE_LOOP ( 'NONE', ( #6037, #1959, #11785, #2373, #6650, #6904, #11054, #14458, #6640 ) ) ;
#3205=AXIS2_PLACEMENT_3D ( 'NONE', #2570, #14112, #3636 ) ;
#3206=ORIENTED_EDGE ( 'NONE', *, *, #2258, .F. ) ;
#3207=DIRECTION ( 'NONE',  ( 0.000000000000000000, 0.000000000000000000, 1.000000000000000000 ) ) ;
#3208=DIRECTION ( 'NONE',  ( 0.000000000000000000, 0.000000000000000000, 1.000000000000000000 ) ) ;
#3209=CARTESIAN_POINT ( 'NONE',  ( 2.449293598294700991E-16, -97.00000000000000000, -8.000000000000000000 ) ) ;
#3210=DIRECTION ( 'NONE',  ( 1.000000000000000000, 0.000000000000000000, 0.000000000000000000 ) ) ;
#3211=CARTESIAN_POINT ( 'NONE',  ( -30.80502811811232888, -49.00442420935981147, 10.49999999999999822 ) ) ;
#3214=DIRECTION ( 'NONE',  ( 0.000000000000000000, 0.000000000000000000, 1.000000000000000000 ) ) ;
#3215=ORIENTED_EDGE ( 'NONE', *, *, #2407, .F. ) ;
#3216=CIRCLE ( 'NONE', #5637, 52.50000000000000711 ) ;
#3217=DIRECTION ( 'NONE',  ( 0.000000000000000000, 0.000000000000000000, 1.000000000000000000 ) ) ;
#3218=DIRECTION ( 'NONE',  ( -1.000000000000000000, 0.000000000000000000, 0.000000000000000000 ) ) ;
#3220=CARTESIAN_POINT ( 'NONE',  ( -3.492805317593278058, 46.55633131742322917, -10.50000000000000000 ) ) ;
#3222=ORIENTED_EDGE ( 'NONE', *, *, #10093, .F. ) ;
#3223=CARTESIAN_POINT ( 'NONE',  ( -56.43380494354004639, -12.86891638962099549, -10.50000000000000000 ) ) ;
#3227=DIRECTION ( 'NONE',  ( 0.000000000000000000, 0.000000000000000000, -1.000000000000000000 ) ) ;
#3228=ORIENTED_EDGE ( 'NONE', *, *, #8429, .T. ) ;
#3229=AXIS2_PLACEMENT_3D ( 'NONE', #7795, #14567, #13421 ) ;
#3231=CARTESIAN_POINT ( 'NONE',  ( 52.50000000000000711, -6.429395695523604744E-15, -13.00000000000000178 ) ) ;
#3232=DIRECTION ( 'NONE',  ( 1.000000000000000000, 0.000000000000000000, 0.000000000000000000 ) ) ;
#3233=ORIENTED_EDGE ( 'NONE', *, *, #11476, .F. ) ;
#3236=DIRECTION ( 'NONE',  ( 1.000000000000000000, 0.000000000000000000, 0.000000000000000000 ) ) ;
#3237=CARTESIAN_POINT ( 'NONE',  ( -37.12029293941250074, 89.61631465359532456, -13.00000000000000178 ) ) ;
#3238=DIRECTION ( 'NONE',  ( -0.000000000000000000, -0.000000000000000000, -1.000000000000000000 ) ) ;
#3239=ORIENTED_EDGE ( 'NONE', *, *, #3299, .F. ) ;
#3240=CIRCLE ( 'NONE', #6365, 63.00000000000000000 ) ;
#3241=ORIENTED_EDGE ( 'NONE', *, *, #7025, .F. ) ;
#3243=ORIENTED_EDGE ( 'NONE', *, *, #7112, .F. ) ;
#3244=AXIS2_PLACEMENT_3D ( 'NONE', #1424, #6033, #2634 ) ;
#3246=CARTESIAN_POINT ( 'NONE',  ( 9.706953719245472456, 57.06275842387054098, -13.00000000000000178 ) ) ;
#3247=CARTESIAN_POINT ( 'NONE',  ( 9.706953719245472456, 57.06275842387054098, 8.000000000000000000 ) ) ;
#3248=CARTESIAN_POINT ( 'NONE',  ( 37.12029293941315444, -89.61631465359504034, -13.00000000000000178 ) ) ;
#3249=CARTESIAN_POINT ( 'NONE',  ( -50.69406879332065330, -13.71740939043347041, -13.00000000000000178 ) ) ;
#3250=CIRCLE ( 'NONE', #4713, 0.5000000000000004441 ) ;
#3251=AXIS2_PLACEMENT_3D ( 'NONE', #11189, #5336, #790 ) ;
#3252=CYLINDRICAL_SURFACE ( 'NONE', #3673, 3.000000000000002665 ) ;
#3254=ORIENTED_EDGE ( 'NONE', *, *, #13997, .F. ) ;
#3255=EDGE_CURVE ( 'NONE', #4753, #1381, #12910, .T. ) ;
#3256=CARTESIAN_POINT ( 'NONE',  ( -56.43380494354004639, -12.86891638962099549, -13.00000000000000178 ) ) ;
#3261=AXIS2_PLACEMENT_3D ( 'NONE', #11841, #9683, #9612 ) ;
#3262=AXIS2_PLACEMENT_3D ( 'NONE', #13302, #271, #14449 ) ;
#3263=EDGE_LOOP ( 'NONE', ( #4692, #7429, #3241, #13964, #12511, #9372 ) ) ;
#3264=DIRECTION ( 'NONE',  ( 1.000000000000000000, 0.000000000000000000, 0.000000000000000000 ) ) ;
#3267=AXIS2_PLACEMENT_3D ( 'NONE', #5221, #8904, #1580 ) ;
#3268=DIRECTION ( 'NONE',  ( 1.000000000000000000, 0.000000000000000000, 0.000000000000000000 ) ) ;
#3269=ORIENTED_EDGE ( 'NONE', *, *, #12432, .T. ) ;
#3272=DIRECTION ( 'NONE',  ( 1.000000000000000000, 0.000000000000000000, 0.000000000000000000 ) ) ;
#3273=CIRCLE ( 'NONE', #12252, 53.55662432702593634 ) ;
#3274=ORIENTED_EDGE ( 'NONE', *, *, #5017, .F. ) ;
#3278=DIRECTION ( 'NONE',  ( 1.000000000000000000, 0.000000000000000000, 0.000000000000000000 ) ) ;
#3279=CIRCLE ( 'NONE', #10071, 3.000000000000002665 ) ;
#3282=DIRECTION ( 'NONE',  ( 1.000000000000000000, 0.000000000000000000, 0.000000000000000000 ) ) ;
#3283=AXIS2_PLACEMENT_3D ( 'NONE', #2960, #9105, #8942 ) ;
#3284=CYLINDRICAL_SURFACE ( 'NONE', #11291, 2.649999999999992806 ) ;
#3288=LINE ( 'NONE', #7909, #3626 ) ;
#3289=EDGE_CURVE ( 'NONE', #4561, #3819, #14859, .T. ) ;
#3291=EDGE_CURVE ( 'NONE', #11078, #8255, #13161, .T. ) ;
#3292=EDGE_CURVE ( 'NONE', #6509, #203, #10238, .T. ) ;
#3293=CARTESIAN_POINT ( 'NONE',  ( 26.01438936481372721, 47.21331623427104063, -10.50000000000000000 ) ) ;
#3294=CIRCLE ( 'NONE', #5712, 59.50000000000000000 ) ;
#3296=DIRECTION ( 'NONE',  ( 0.000000000000000000, 0.000000000000000000, 1.000000000000000000 ) ) ;
#3297=DIRECTION ( 'NONE',  ( 0.000000000000000000, 0.000000000000000000, 1.000000000000000000 ) ) ;
#3298=FACE_OUTER_BOUND ( 'NONE', #9987, .T. ) ;
#3299=EDGE_CURVE ( 'NONE', #12763, #6631, #9273, .T. ) ;
#3300=DIRECTION ( 'NONE',  ( 0.000000000000000000, 0.000000000000000000, 1.000000000000000000 ) ) ;
#3301=VERTEX_POINT ( 'NONE', #10437 ) ;
#3302=CIRCLE ( 'NONE', #1599, 3.000000000000002665 ) ;
#3305=ORIENTED_EDGE ( 'NONE', *, *, #11458, .T. ) ;
#3306=DIRECTION ( 'NONE',  ( 0.000000000000000000, 0.000000000000000000, -1.000000000000000000 ) ) ;
#3307=CARTESIAN_POINT ( 'NONE',  ( 37.12029293941315444, -89.61631465359504034, -8.000000000000000000 ) ) ;
#3308=CARTESIAN_POINT ( 'NONE',  ( 9.706953719245472456, 57.06275842387054098, -8.000000000000000000 ) ) ;
#3310=ORIENTED_EDGE ( 'NONE', *, *, #5017, .T. ) ;
#3311=EDGE_CURVE ( 'NONE', #8664, #14518, #14369, .T. ) ;
#3313=ORIENTED_EDGE ( 'NONE', *, *, #13919, .T. ) ;
#3314=AXIS2_PLACEMENT_3D ( 'NONE', #1697, #5195, #9885 ) ;
#3315=CYLINDRICAL_SURFACE ( 'NONE', #5719, 0.5000000000000022204 ) ;
#3317=CARTESIAN_POINT ( 'NONE',  ( 2.449293598294700991E-16, -97.00000000000000000, -8.000000000000000000 ) ) ;
#3321=EDGE_LOOP ( 'NONE', ( #10041, #10010, #996, #6082 ) ) ;
#3322=AXIS2_PLACEMENT_3D ( 'NONE', #10118, #9277, #13929 ) ;
#3324=CARTESIAN_POINT ( 'NONE',  ( 47.21331623427115431, 33.48561063518610581, 10.49999999999999822 ) ) ;
#3326=CYLINDRICAL_SURFACE ( 'NONE', #1861, 59.50000000000000000 ) ;
#3328=ORIENTED_EDGE ( 'NONE', *, *, #4719, .F. ) ;
#3329=DIRECTION ( 'NONE',  ( 1.000000000000000000, 0.000000000000000000, 0.000000000000000000 ) ) ;
#3330=DIRECTION ( 'NONE',  ( 0.000000000000000000, 0.000000000000000000, 1.000000000000000000 ) ) ;
#3332=EDGE_CURVE ( 'NONE', #12052, #6195, #9150, .T. ) ;
#3333=ORIENTED_EDGE ( 'NONE', *, *, #12594, .T. ) ;
#3337=ADVANCED_FACE ( 'NONE', ( #1183 ), #6939, .F. ) ;
#3340=DIRECTION ( 'NONE',  ( -1.000000000000000000, 9.175396897728567444E-16, 0.000000000000000000 ) ) ;
#3344=ORIENTED_EDGE ( 'NONE', *, *, #9352, .T. ) ;
#3345=EDGE_CURVE ( 'NONE', #3039, #11882, #7813, .T. ) ;
#3346=CARTESIAN_POINT ( 'NONE',  ( -42.04772703543551415, -32.26435573746212526, -8.000000000000000000 ) ) ;
#3347=DIRECTION ( 'NONE',  ( 0.000000000000000000, 0.000000000000000000, 1.000000000000000000 ) ) ;
#3348=ORIENTED_EDGE ( 'NONE', *, *, #2296, .T. ) ;
#3349=CARTESIAN_POINT ( 'NONE',  ( 89.89283556784508278, -37.53686968382275779, -13.00000000000000178 ) ) ;
#3350=ORIENTED_EDGE ( 'NONE', *, *, #4500, .F. ) ;
#3353=DIRECTION ( 'NONE',  ( 0.000000000000000000, 0.000000000000000000, -1.000000000000000000 ) ) ;
#3354=FACE_OUTER_BOUND ( 'NONE', #5895, .T. ) ;
#3359=ORIENTED_EDGE ( 'NONE', *, *, #6971, .F. ) ;
#3360=DIRECTION ( 'NONE',  ( -1.000000000000000000, 0.000000000000000000, 0.000000000000000000 ) ) ;
#3361=CARTESIAN_POINT ( 'NONE',  ( 33.48561063518626923, -47.21331623427104063, 10.49999999999999822 ) ) ;
#3362=DIRECTION ( 'NONE',  ( 0.000000000000000000, 0.000000000000000000, 1.000000000000000000 ) ) ;
#3363=CARTESIAN_POINT ( 'NONE',  ( -42.04772703543551415, -32.26435573746212526, -10.50000000000000000 ) ) ;
#3365=EDGE_CURVE ( 'NONE', #2335, #13021, #13394, .T. ) ;
#3367=EDGE_CURVE ( 'NONE', #967, #3376, #13898, .T. ) ;
#3369=FACE_OUTER_BOUND ( 'NONE', #4376, .T. ) ;
#3370=FACE_OUTER_BOUND ( 'NONE', #11300, .T. ) ;
#3372=DIRECTION ( 'NONE',  ( 1.000000000000000000, 0.000000000000000000, 0.000000000000000000 ) ) ;
#3373=DIRECTION ( 'NONE',  ( -0.000000000000000000, -0.000000000000000000, 1.000000000000000000 ) ) ;
#3376=VERTEX_POINT ( 'NONE', #6781 ) ;
#3377=ORIENTED_EDGE ( 'NONE', *, *, #12523, .T. ) ;
#3380=DIRECTION ( 'NONE',  ( -1.000000000000000000, 0.000000000000000000, 0.000000000000000000 ) ) ;
#3381=DIRECTION ( 'NONE',  ( 1.000000000000000000, 0.000000000000000000, 0.000000000000000000 ) ) ;
#3384=ORIENTED_EDGE ( 'NONE', *, *, #8246, .T. ) ;
#3387=ORIENTED_EDGE ( 'NONE', *, *, #7926, .F. ) ;
#3391=DIRECTION ( 'NONE',  ( -0.000000000000000000, -0.000000000000000000, 1.000000000000000000 ) ) ;
#3394=AXIS2_PLACEMENT_3D ( 'NONE', #11038, #5190, #13017 ) ;
#3397=ORIENTED_EDGE ( 'NONE', *, *, #2435, .T. ) ;
#3398=CARTESIAN_POINT ( 'NONE',  ( 0.000000000000000000, 0.000000000000000000, 10.50000000000000000 ) ) ;
#3399=ORIENTED_EDGE ( 'NONE', *, *, #2956, .F. ) ;
#3400=CIRCLE ( 'NONE', #3891, 60.50000000000000000 ) ;
#3403=ORIENTED_EDGE ( 'NONE', *, *, #6611, .F. ) ;
#3404=AXIS2_PLACEMENT_3D ( 'NONE', #2979, #9037, #5553 ) ;
#3405=EDGE_LOOP ( 'NONE', ( #10883, #13151, #4480, #3749, #11608, #2485, #11173, #1742, #540, #8841 ) ) ;
#3406=DIRECTION ( 'NONE',  ( 1.000000000000000000, 0.000000000000000000, -0.000000000000000000 ) ) ;
#3407=AXIS2_PLACEMENT_3D ( 'NONE', #5629, #6530, #11188 ) ;
#3408=ORIENTED_EDGE ( 'NONE', *, *, #2376, .F. ) ;
#3409=ORIENTED_EDGE ( 'NONE', *, *, #7532, .T. ) ;
#3410=DIRECTION ( 'NONE',  ( -0.000000000000000000, -0.000000000000000000, -1.000000000000000000 ) ) ;
#3411=EDGE_CURVE ( 'NONE', #10761, #4919, #7563, .T. ) ;
#3412=CARTESIAN_POINT ( 'NONE',  ( 45.91029614918936375, -26.00011991137331790, 10.49999999999999822 ) ) ;
#3414=EDGE_CURVE ( 'NONE', #5837, #5604, #6590, .T. ) ;
#3417=AXIS2_PLACEMENT_3D ( 'NONE', #6443, #7735, #11328 ) ;
#3418=ORIENTED_EDGE ( 'NONE', *, *, #14716, .F. ) ;
#3419=CIRCLE ( 'NONE', #6546, 3.000000000000002665 ) ;
#3421=EDGE_LOOP ( 'NONE', ( #1119, #1872, #10794, #12340, #4213, #3702, #7733, #6997, #10903, #14424, #7046 ) ) ;
#3422=AXIS2_PLACEMENT_3D ( 'NONE', #9189, #11411, #5848 ) ;
#3424=ADVANCED_FACE ( 'NONE', ( #13872 ), #7934, .T. ) ;
#3425=CARTESIAN_POINT ( 'NONE',  ( 0.000000000000000000, 0.000000000000000000, -8.000000000000000000 ) ) ;
#3428=ORIENTED_EDGE ( 'NONE', *, *, #12098, .T. ) ;
#3430=DIRECTION ( 'NONE',  ( -0.000000000000000000, -0.000000000000000000, 1.000000000000000000 ) ) ;
#3431=EDGE_LOOP ( 'NONE', ( #14921, #4444, #7666, #7971 ) ) ;
#3433=VECTOR ( 'NONE', #8460, 1000.000000000000000 ) ;
#3434=EDGE_CURVE ( 'NONE', #3819, #7980, #3463, .T. ) ;
#3435=ADVANCED_FACE ( 'NONE', ( #2163 ), #11445, .F. ) ;
#3437=DIRECTION ( 'NONE',  ( 1.000000000000000000, 0.000000000000000000, 0.000000000000000000 ) ) ;
#3438=CARTESIAN_POINT ( 'NONE',  ( 52.36539807335608288, -6.451868917687384020, -10.50000000000000000 ) ) ;
#3439=DIRECTION ( 'NONE',  ( 0.000000000000000000, 0.000000000000000000, 1.000000000000000000 ) ) ;
#3441=CARTESIAN_POINT ( 'NONE',  ( -26.49999999999971578, -45.89934640057541060, -10.50000000000000000 ) ) ;
#3442=CIRCLE ( 'NONE', #8287, 50.00000000000000000 ) ;
#3443=ORIENTED_EDGE ( 'NONE', *, *, #13676, .T. ) ;
#3445=CARTESIAN_POINT ( 'NONE',  ( 0.000000000000000000, 0.000000000000000000, -10.50000000000000000 ) ) ;
#3446=CIRCLE ( 'NONE', #13910, 3.000000000000002665 ) ;
#3447=AXIS2_PLACEMENT_3D ( 'NONE', #12453, #9249, #10393 ) ;
#3448=CARTESIAN_POINT ( 'NONE',  ( 50.84834283436990177, 14.07862063237912054, -10.50000000000000000 ) ) ;
#3449=DIRECTION ( 'NONE',  ( 1.000000000000000000, 0.000000000000000000, 0.000000000000000000 ) ) ;
#3450=VERTEX_POINT ( 'NONE', #5662 ) ;
#3451=DIRECTION ( 'NONE',  ( 0.000000000000000000, 0.000000000000000000, 1.000000000000000000 ) ) ;
#3452=ORIENTED_EDGE ( 'NONE', *, *, #4242, .T. ) ;
#3456=LINE ( 'NONE', #12792, #1255 ) ;
#3457=CIRCLE ( 'NONE', #7317, 60.50000000000000711 ) ;
#3458=CARTESIAN_POINT ( 'NONE',  ( -56.43380494354004639, -12.86891638962099549, 10.49999999999999822 ) ) ;
#3460=CARTESIAN_POINT ( 'NONE',  ( 97.00000000000000000, -3.384287605079545030E-13, -13.00000000000000178 ) ) ;
#3462=CIRCLE ( 'NONE', #11956, 0.5000000000000022204 ) ;
#3463=LINE ( 'NONE', #13950, #5873 ) ;
#3464=VERTEX_POINT ( 'NONE', #1260 ) ;
#3465=AXIS2_PLACEMENT_3D ( 'NONE', #12621, #3439, #10486 ) ;
#3466=ORIENTED_EDGE ( 'NONE', *, *, #4698, .F. ) ;
#3467=EDGE_LOOP ( 'NONE', ( #653, #3348, #4904, #12007, #3792, #9478, #8141, #14632, #7264, #6424 ) ) ;
#3470=DIRECTION ( 'NONE',  ( 0.000000000000000000, 0.000000000000000000, 1.000000000000000000 ) ) ;
#3471=DIRECTION ( 'NONE',  ( -1.000000000000000000, 0.000000000000000000, 0.000000000000000000 ) ) ;
#3473=DIRECTION ( 'NONE',  ( 1.000000000000000000, 0.000000000000000000, 0.000000000000000000 ) ) ;
#3474=ORIENTED_EDGE ( 'NONE', *, *, #3414, .T. ) ;
#3476=ORIENTED_EDGE ( 'NONE', *, *, #14087, .F. ) ;
#3480=EDGE_CURVE ( 'NONE', #877, #7720, #3837, .T. ) ;
#3481=CYLINDRICAL_SURFACE ( 'NONE', #7863, 3.000000000000004441 ) ;
#3482=DIRECTION ( 'NONE',  ( 0.000000000000000000, 0.000000000000000000, 1.000000000000000000 ) ) ;
#3486=ORIENTED_EDGE ( 'NONE', *, *, #7477, .T. ) ;
#3488=VERTEX_POINT ( 'NONE', #6098 ) ;
#3489=ORIENTED_EDGE ( 'NONE', *, *, #744, .T. ) ;
#3490=CIRCLE ( 'NONE', #7106, 56.99999999999998579 ) ;
#3494=DIRECTION ( 'NONE',  ( 0.000000000000000000, 0.000000000000000000, 1.000000000000000000 ) ) ;
#3495=DIRECTION ( 'NONE',  ( 1.000000000000000000, 0.000000000000000000, 0.000000000000000000 ) ) ;
#3496=EDGE_LOOP ( 'NONE', ( #9002, #4538, #3928, #5576, #3004, #1098, #4357, #305, #4849 ) ) ;
#3497=CARTESIAN_POINT ( 'NONE',  ( -89.61631465359519666, -37.12029293941281338, -8.000000000000000000 ) ) ;
#3498=ORIENTED_EDGE ( 'NONE', *, *, #13128, .F. ) ;
#3499=FACE_OUTER_BOUND ( 'NONE', #7883, .T. ) ;
#3500=AXIS2_PLACEMENT_3D ( 'NONE', #5033, #244, #9640 ) ;
#3501=CIRCLE ( 'NONE', #14170, 52.50000000000000711 ) ;
#3502=AXIS2_PLACEMENT_3D ( 'NONE', #14114, #295, #8554 ) ;
#3503=CYLINDRICAL_SURFACE ( 'NONE', #948, 60.50000000000000000 ) ;
#3504=AXIS2_PLACEMENT_3D ( 'NONE', #8822, #3135, #6610 ) ;
#3505=EDGE_CURVE ( 'NONE', #4977, #10396, #2475, .T. ) ;
#3506=EDGE_LOOP ( 'NONE', ( #8916, #4758, #949, #1686 ) ) ;
#3507=DIRECTION ( 'NONE',  ( 0.000000000000000000, 0.000000000000000000, 1.000000000000000000 ) ) ;
#3510=CARTESIAN_POINT ( 'NONE',  ( 89.61631465359491244, 37.12029293941346708, -8.000000000000000000 ) ) ;
#3512=DIRECTION ( 'NONE',  ( 0.000000000000000000, 0.000000000000000000, 1.000000000000000000 ) ) ;
#3513=CARTESIAN_POINT ( 'NONE',  ( -55.00000000000000000, 0.000000000000000000, -13.00000000000000178 ) ) ;
#3514=AXIS2_PLACEMENT_3D ( 'NONE', #5749, #9162, #11463 ) ;
#3515=AXIS2_PLACEMENT_3D ( 'NONE', #2384, #7001, #4602 ) ;
#3520=ORIENTED_EDGE ( 'NONE', *, *, #3332, .F. ) ;
#3521=DIRECTION ( 'NONE',  ( -0.000000000000000000, -0.000000000000000000, 1.000000000000000000 ) ) ;
#3522=DIRECTION ( 'NONE',  ( 1.000000000000000000, 1.243449787580175325E-13, 0.000000000000000000 ) ) ;
#3523=EDGE_CURVE ( 'NONE', #8423, #511, #13635, .T. ) ;
#3524=AXIS2_PLACEMENT_3D ( 'NONE', #7765, #14326, #2080 ) ;
#3526=LINE ( 'NONE', #1238, #1051 ) ;
#3527=AXIS2_PLACEMENT_3D ( 'NONE', #13401, #11203, #12565 ) ;
#3528=CIRCLE ( 'NONE', #4981, 63.00000000000000000 ) ;
#3529=CARTESIAN_POINT ( 'NONE',  ( 37.21932736666271779, -89.12622059913267947, -13.00000000000000178 ) ) ;
#3530=ORIENTED_EDGE ( 'NONE', *, *, #9973, .F. ) ;
#3533=DIRECTION ( 'NONE',  ( 0.000000000000000000, 0.000000000000000000, 1.000000000000000000 ) ) ;
#3534=CARTESIAN_POINT ( 'NONE',  ( -25.99999999999971223, -45.89934640057541060, -13.00000000000000178 ) ) ;
#3538=DIRECTION ( 'NONE',  ( -0.000000000000000000, -0.000000000000000000, 1.000000000000000000 ) ) ;
#3541=DIRECTION ( 'NONE',  ( 0.000000000000000000, 0.000000000000000000, -1.000000000000000000 ) ) ;
#3542=CYLINDRICAL_SURFACE ( 'NONE', #3515, 2.649999999999992806 ) ;
#3544=CARTESIAN_POINT ( 'NONE',  ( 50.00000000000000000, 6.123233995736766085E-15, 13.00000000000000178 ) ) ;
#3545=CIRCLE ( 'NONE', #12037, 60.50000000000000000 ) ;
#3546=ORIENTED_EDGE ( 'NONE', *, *, #6983, .T. ) ;
#3548=ORIENTED_EDGE ( 'NONE', *, *, #12478, .T. ) ;
#3549=VERTEX_POINT ( 'NONE', #2616 ) ;
#3550=DIRECTION ( 'NONE',  ( 1.000000000000000000, 0.000000000000000000, 0.000000000000000000 ) ) ;
#3551=LINE ( 'NONE', #9523, #14825 ) ;
#3553=FACE_OUTER_BOUND ( 'NONE', #6311, .T. ) ;
#3554=CIRCLE ( 'NONE', #13484, 0.5000000000000038858 ) ;
#3555=CARTESIAN_POINT ( 'NONE',  ( 0.000000000000000000, 0.000000000000000000, -13.00000000000000178 ) ) ;
#3556=ORIENTED_EDGE ( 'NONE', *, *, #13066, .F. ) ;
#3557=ORIENTED_EDGE ( 'NONE', *, *, #11019, .T. ) ;
#3558=DIRECTION ( 'NONE',  ( 0.000000000000000000, 0.000000000000000000, 1.000000000000000000 ) ) ;
#3559=CARTESIAN_POINT ( 'NONE',  ( 69.08935777509475429, -68.58935777509547904, 10.49999999999999822 ) ) ;
#3560=ORIENTED_EDGE ( 'NONE', *, *, #3569, .T. ) ;
#3561=ORIENTED_EDGE ( 'NONE', *, *, #1434, .T. ) ;
#3562=PLANE ( 'NONE',  #13211 ) ;
#3563=CIRCLE ( 'NONE', #11080, 3.000000000000002665 ) ;
#3564=ORIENTED_EDGE ( 'NONE', *, *, #4887, .F. ) ;
#3565=ORIENTED_EDGE ( 'NONE', *, *, #9807, .T. ) ;
#3566=ADVANCED_FACE ( 'NONE', ( #483 ), #9514, .T. ) ;
#3567=DIRECTION ( 'NONE',  ( 0.000000000000000000, 0.000000000000000000, 1.000000000000000000 ) ) ;
#3568=CARTESIAN_POINT ( 'NONE',  ( -53.06332297728247482, 7.252293700257352427, -10.50000000000000000 ) ) ;
#3569=EDGE_CURVE ( 'NONE', #6334, #1115, #12676, .T. ) ;
#3570=CARTESIAN_POINT ( 'NONE',  ( -49.11971303961688307, -15.88467684210530528, -8.000000000000000000 ) ) ;
#3571=DIRECTION ( 'NONE',  ( 1.000000000000000000, 0.000000000000000000, 0.000000000000000000 ) ) ;
#3573=CARTESIAN_POINT ( 'NONE',  ( -26.99988008862626643, -45.88839665196127271, -10.50000000000000000 ) ) ;
#3574=ORIENTED_EDGE ( 'NONE', *, *, #12668, .T. ) ;
#3575=EDGE_CURVE ( 'NONE', #5656, #1886, #3703, .T. ) ;
#3576=DIRECTION ( 'NONE',  ( 1.000000000000000000, 0.000000000000000000, 0.000000000000000000 ) ) ;
#3577=CARTESIAN_POINT ( 'NONE',  ( 0.000000000000000000, 0.000000000000000000, 8.000000000000000000 ) ) ;
#3578=ORIENTED_EDGE ( 'NONE', *, *, #9207, .F. ) ;
#3581=ORIENTED_EDGE ( 'NONE', *, *, #5772, .F. ) ;
#3583=VERTEX_POINT ( 'NONE', #11887 ) ;
#3585=CARTESIAN_POINT ( 'NONE',  ( 40.12029293941316155, -89.61631465359504034, 8.000000000000000000 ) ) ;
#3586=CARTESIAN_POINT ( 'NONE',  ( 90.11631465359468507, -37.12029293941410657, -10.50000000000000000 ) ) ;
#3587=CARTESIAN_POINT ( 'NONE',  ( 51.19406879332056093, 13.71740939043382745, -10.50000000000000000 ) ) ;
#3588=PLANE ( 'NONE',  #11231 ) ;
#3594=AXIS2_PLACEMENT_3D ( 'NONE', #5170, #4478, #9092 ) ;
#3595=DIRECTION ( 'NONE',  ( 1.000000000000000000, 0.000000000000000000, 0.000000000000000000 ) ) ;
#3597=CYLINDRICAL_SURFACE ( 'NONE', #12486, 50.00000000000000000 ) ;
#3598=ORIENTED_EDGE ( 'NONE', *, *, #2673, .F. ) ;
#3600=CARTESIAN_POINT ( 'NONE',  ( -33.48561063518626923, 47.21331623427104063, 10.49999999999999822 ) ) ;
#3601=ORIENTED_EDGE ( 'NONE', *, *, #374, .F. ) ;
#3602=DIRECTION ( 'NONE',  ( -0.000000000000000000, -0.000000000000000000, 1.000000000000000000 ) ) ;
#3604=EDGE_CURVE ( 'NONE', #4704, #9453, #10817, .T. ) ;
#3606=CARTESIAN_POINT ( 'NONE',  ( 0.000000000000000000, 0.000000000000000000, -10.50000000000000000 ) ) ;
#3607=ADVANCED_FACE ( 'NONE', ( #14303 ), #3914, .F. ) ;
#3608=CARTESIAN_POINT ( 'NONE',  ( -26.00011991137315803, -45.91029614918952007, -10.50000000000000000 ) ) ;
#3610=DIRECTION ( 'NONE',  ( 0.000000000000000000, 0.000000000000000000, 1.000000000000000000 ) ) ;
#3611=VECTOR ( 'NONE', #15029, 1000.000000000000000 ) ;
#3614=ORIENTED_EDGE ( 'NONE', *, *, #880, .T. ) ;
#3615=EDGE_CURVE ( 'NONE', #5777, #14224, #3462, .T. ) ;
#3617=ORIENTED_EDGE ( 'NONE', *, *, #3202, .T. ) ;
#3619=DIRECTION ( 'NONE',  ( 0.000000000000000000, 0.000000000000000000, -1.000000000000000000 ) ) ;
#3621=CARTESIAN_POINT ( 'NONE',  ( -36.14014761921588104, 11.74264578624790190, -28.00000000000000000 ) ) ;
#3622=CARTESIAN_POINT ( 'NONE',  ( 0.000000000000000000, 0.000000000000000000, -10.50000000000000000 ) ) ;
#3623=DIRECTION ( 'NONE',  ( 0.000000000000000000, 0.000000000000000000, 1.000000000000000000 ) ) ;
#3625=DIRECTION ( 'NONE',  ( 1.000000000000000000, 0.000000000000000000, -0.000000000000000000 ) ) ;
#3626=VECTOR ( 'NONE', #6753, 1000.000000000000000 ) ;
#3627=DIRECTION ( 'NONE',  ( 1.000000000000000000, 0.000000000000000000, 0.000000000000000000 ) ) ;
#3629=ORIENTED_EDGE ( 'NONE', *, *, #5776, .F. ) ;
#3631=FACE_OUTER_BOUND ( 'NONE', #3203, .T. ) ;
#3633=VERTEX_POINT ( 'NONE', #14382 ) ;
#3634=CARTESIAN_POINT ( 'NONE',  ( 9.706953719245472456, 57.06275842387054098, -13.00000000000000178 ) ) ;
#3635=CIRCLE ( 'NONE', #10900, 0.5000000000000004441 ) ;
#3636=DIRECTION ( 'NONE',  ( 1.000000000000000000, 0.000000000000000000, 0.000000000000000000 ) ) ;
#3637=CARTESIAN_POINT ( 'NONE',  ( 99.48933418828643482, -1.674280531759671176, 8.000000000000000000 ) ) ;
#3640=DIRECTION ( 'NONE',  ( 0.000000000000000000, 0.000000000000000000, 1.000000000000000000 ) ) ;
#3642=ADVANCED_FACE ( 'NONE', ( #13051 ), #13205, .F. ) ;
#3644=CIRCLE ( 'NONE', #7500, 0.5000000000000043299 ) ;
#3646=EDGE_CURVE ( 'NONE', #3918, #14223, #553, .T. ) ;
#3648=CIRCLE ( 'NONE', #12136, 2.649999999999985700 ) ;
#3649=VERTEX_POINT ( 'NONE', #1409 ) ;
#3651=ORIENTED_EDGE ( 'NONE', *, *, #9405, .T. ) ;
#3653=LINE ( 'NONE', #2360, #5818 ) ;
#3654=CIRCLE ( 'NONE', #242, 59.50000000000000000 ) ;
#3655=FACE_OUTER_BOUND ( 'NONE', #11358, .T. ) ;
#3657=DIRECTION ( 'NONE',  ( -1.000000000000000000, 0.000000000000000000, 0.000000000000000000 ) ) ;
#3659=CIRCLE ( 'NONE', #12147, 53.55662432702593634 ) ;
#3660=ORIENTED_EDGE ( 'NONE', *, *, #7325, .F. ) ;
#3661=CARTESIAN_POINT ( 'NONE',  ( -51.19406879332065330, -13.71740939043347041, 8.000000000000000000 ) ) ;
#3662=VERTEX_POINT ( 'NONE', #648 ) ;
#3663=EDGE_CURVE ( 'NONE', #4909, #2144, #4684, .T. ) ;
#3664=ADVANCED_FACE ( 'NONE', ( #6619 ), #7762, .T. ) ;
#3665=EDGE_CURVE ( 'NONE', #10864, #10761, #4204, .T. ) ;
#3666=CIRCLE ( 'NONE', #268, 0.5000000000000004441 ) ;
#3669=CIRCLE ( 'NONE', #8014, 56.99999999999999289 ) ;
#3671=EDGE_CURVE ( 'NONE', #9386, #5754, #11725, .T. ) ;
#3672=LINE ( 'NONE', #11952, #14160 ) ;
#3673=AXIS2_PLACEMENT_3D ( 'NONE', #5382, #10147, #1810 ) ;
#3674=EDGE_LOOP ( 'NONE', ( #6882, #7316, #13379, #9845, #10345 ) ) ;
#3675=DIRECTION ( 'NONE',  ( 0.000000000000000000, 0.000000000000000000, 1.000000000000000000 ) ) ;
#3676=ORIENTED_EDGE ( 'NONE', *, *, #10787, .F. ) ;
#3679=CYLINDRICAL_SURFACE ( 'NONE', #4188, 3.000000000000002665 ) ;
#3681=FACE_OUTER_BOUND ( 'NONE', #4322, .T. ) ;
#3682=DIRECTION ( 'NONE',  ( -1.000000000000000000, 0.000000000000000000, 0.000000000000000000 ) ) ;
#3683=ORIENTED_EDGE ( 'NONE', *, *, #5722, .F. ) ;
#3684=AXIS2_PLACEMENT_3D ( 'NONE', #4366, #8982, #5503 ) ;
#3685=ORIENTED_EDGE ( 'NONE', *, *, #1113, .T. ) ;
#3686=CARTESIAN_POINT ( 'NONE',  ( 0.000000000000000000, 0.000000000000000000, -8.000000000000000000 ) ) ;
#3687=CARTESIAN_POINT ( 'NONE',  ( 45.89934640057532533, -26.49999999999987566, 10.49999999999999822 ) ) ;
#3689=ORIENTED_EDGE ( 'NONE', *, *, #7960, .T. ) ;
#3690=CIRCLE ( 'NONE', #12175, 3.000000000000002665 ) ;
#3692=VERTEX_POINT ( 'NONE', #1919 ) ;
#3702=ORIENTED_EDGE ( 'NONE', *, *, #81, .T. ) ;
#3703=CIRCLE ( 'NONE', #14619, 3.000000000000002665 ) ;
#3704=ORIENTED_EDGE ( 'NONE', *, *, #9865, .F. ) ;
#3705=ORIENTED_EDGE ( 'NONE', *, *, #1912, .T. ) ;
#3706=CARTESIAN_POINT ( 'NONE',  ( -26.00011991137315803, -45.91029614918952007, -13.00000000000000178 ) ) ;
#3707=CARTESIAN_POINT ( 'NONE',  ( 37.62029293941316155, -89.61631465359504034, -13.00000000000000178 ) ) ;
#3708=DIRECTION ( 'NONE',  ( 0.000000000000000000, 0.000000000000000000, -1.000000000000000000 ) ) ;
#3710=EDGE_CURVE ( 'NONE', #11690, #10452, #3715, .T. ) ;
#3711=EDGE_CURVE ( 'NONE', #1924, #12179, #12267, .T. ) ;
#3712=ORIENTED_EDGE ( 'NONE', *, *, #2547, .T. ) ;
#3713=DIRECTION ( 'NONE',  ( 1.000000000000000000, 0.000000000000000000, 0.000000000000000000 ) ) ;
#3715=CIRCLE ( 'NONE', #11716, 63.00000000000000000 ) ;
#3716=CARTESIAN_POINT ( 'NONE',  ( 56.43380494353997534, 12.86891638962136319, -13.00000000000000178 ) ) ;
#3717=DIRECTION ( 'NONE',  ( 0.000000000000000000, 0.000000000000000000, 1.000000000000000000 ) ) ;
#3718=AXIS2_PLACEMENT_3D ( 'NONE', #13294, #10941, #7290 ) ;
#3719=CARTESIAN_POINT ( 'NONE',  ( -68.01302780753309207, 65.64523757230344359, -8.000000000000000000 ) ) ;
#3720=DIRECTION ( 'NONE',  ( 0.000000000000000000, 0.000000000000000000, 1.000000000000000000 ) ) ;
#3721=EDGE_CURVE ( 'NONE', #5754, #900, #1855, .T. ) ;
#3724=CARTESIAN_POINT ( 'NONE',  ( 89.61631465359468507, -37.12029293941410657, -10.50000000000000000 ) ) ;
#3725=ORIENTED_EDGE ( 'NONE', *, *, #1890, .F. ) ;
#3729=ORIENTED_EDGE ( 'NONE', *, *, #8166, .F. ) ;
#3730=ORIENTED_EDGE ( 'NONE', *, *, #13168, .F. ) ;
#3732=AXIS2_PLACEMENT_3D ( 'NONE', #10431, #106, #13788 ) ;
#3735=LINE ( 'NONE', #388, #14811 ) ;
#3737=CARTESIAN_POINT ( 'NONE',  ( 57.06275842387049835, -9.706953719245678514, -13.00000000000000178 ) ) ;
#3738=LINE ( 'NONE', #8359, #7494 ) ;
#3740=ORIENTED_EDGE ( 'NONE', *, *, #408, .T. ) ;
#3741=AXIS2_PLACEMENT_3D ( 'NONE', #9280, #9051, #5860 ) ;
#3742=CARTESIAN_POINT ( 'NONE',  ( 92.61631465359468507, -37.12029293941410657, 8.000000000000000000 ) ) ;
#3743=VECTOR ( 'NONE', #1369, 1000.000000000000000 ) ;
#3744=ORIENTED_EDGE ( 'NONE', *, *, #10613, .F. ) ;
#3745=DIRECTION ( 'NONE',  ( -0.000000000000000000, -0.000000000000000000, -1.000000000000000000 ) ) ;
#3749=ORIENTED_EDGE ( 'NONE', *, *, #12954, .T. ) ;
#3750=ORIENTED_EDGE ( 'NONE', *, *, #13962, .F. ) ;
#3751=CIRCLE ( 'NONE', #7373, 56.99999999999999289 ) ;
#3753=CARTESIAN_POINT ( 'NONE',  ( 6.917888187663118416, 52.54657765281190507, -13.00000000000000178 ) ) ;
#3755=ORIENTED_EDGE ( 'NONE', *, *, #7926, .T. ) ;
#3757=EDGE_CURVE ( 'NONE', #9770, #8423, #7573, .T. ) ;
#3758=CARTESIAN_POINT ( 'NONE',  ( -99.48933418828642061, 1.674280531760366397, -8.000000000000000000 ) ) ;
#3761=CARTESIAN_POINT ( 'NONE',  ( -42.89934640057513349, 26.50000000000019540, -13.00000000000000178 ) ) ;
#3762=AXIS2_PLACEMENT_3D ( 'NONE', #512, #588, #10989 ) ;
#3763=ORIENTED_EDGE ( 'NONE', *, *, #4719, .T. ) ;
#3764=CIRCLE ( 'NONE', #12006, 3.000000000000002665 ) ;
#3765=ORIENTED_EDGE ( 'NONE', *, *, #665, .T. ) ;
#3766=DIRECTION ( 'NONE',  ( -1.000000000000000000, 0.000000000000000000, 0.000000000000000000 ) ) ;
#3767=FACE_OUTER_BOUND ( 'NONE', #5152, .T. ) ;
#3768=AXIS2_PLACEMENT_3D ( 'NONE', #6376, #191, #4121 ) ;
#3769=DIRECTION ( 'NONE',  ( -0.000000000000000000, -0.000000000000000000, 1.000000000000000000 ) ) ;
#3770=VERTEX_POINT ( 'NONE', #5272 ) ;
#3773=ORIENTED_EDGE ( 'NONE', *, *, #853, .T. ) ;
#3774=CARTESIAN_POINT ( 'NONE',  ( 0.000000000000000000, 0.000000000000000000, 13.00000000000000178 ) ) ;
#3775=ADVANCED_FACE ( 'NONE', ( #12184 ), #9887, .F. ) ;
#3778=CARTESIAN_POINT ( 'NONE',  ( -47.21331623427138879, -33.48561063518577896, -13.00000000000000178 ) ) ;
#3782=ORIENTED_EDGE ( 'NONE', *, *, #13127, .F. ) ;
#3786=CIRCLE ( 'NONE', #12516, 100.0000000000000000 ) ;
#3788=DIRECTION ( 'NONE',  ( 0.000000000000000000, 0.000000000000000000, 1.000000000000000000 ) ) ;
#3789=AXIS2_PLACEMENT_3D ( 'NONE', #13358, #13217, #6500 ) ;
#3790=CARTESIAN_POINT ( 'NONE',  ( -97.41488903138106537, 0.2790467552942557661, -13.00000000000000178 ) ) ;
#3791=EDGE_LOOP ( 'NONE', ( #11149, #5966, #14013, #14976 ) ) ;
#3792=ORIENTED_EDGE ( 'NONE', *, *, #12667, .T. ) ;
#3793=CARTESIAN_POINT ( 'NONE',  ( 12.86891638962116247, -56.43380494354001087, 8.000000000000000000 ) ) ;
#3795=AXIS2_PLACEMENT_3D ( 'NONE', #1478, #6016, #6096 ) ;
#3798=DIRECTION ( 'NONE',  ( -0.000000000000000000, -0.000000000000000000, 1.000000000000000000 ) ) ;
#3799=EDGE_CURVE ( 'NONE', #2645, #5275, #12448, .T. ) ;
#3800=CYLINDRICAL_SURFACE ( 'NONE', #14826, 56.99999999999999289 ) ;
#3801=DIRECTION ( 'NONE',  ( 0.000000000000000000, 0.000000000000000000, -1.000000000000000000 ) ) ;
#3802=ADVANCED_FACE ( 'NONE', ( #12488 ), #1171, .T. ) ;
#3803=VERTEX_POINT ( 'NONE', #6922 ) ;
#3804=DIRECTION ( 'NONE',  ( -1.000000000000000000, -1.065814103640150279E-14, 0.000000000000000000 ) ) ;
#3806=EDGE_LOOP ( 'NONE', ( #9086, #7248 ) ) ;
#3809=ADVANCED_FACE ( 'NONE', ( #6846 ), #6987, .T. ) ;
#3810=DIRECTION ( 'NONE',  ( 1.000000000000000000, 0.000000000000000000, 0.000000000000000000 ) ) ;
#3811=AXIS2_PLACEMENT_3D ( 'NONE', #14726, #2107, #13649 ) ;
#3812=CARTESIAN_POINT ( 'NONE',  ( -3.492805317593278058, 46.55633131742322917, -10.50000000000000000 ) ) ;
#3814=CARTESIAN_POINT ( 'NONE',  ( -42.04772703543551415, -32.26435573746212526, -13.00000000000000178 ) ) ;
#3815=DIRECTION ( 'NONE',  ( 0.000000000000000000, 0.000000000000000000, 1.000000000000000000 ) ) ;
#3816=CIRCLE ( 'NONE', #12299, 0.5000000000000073275 ) ;
#3818=EDGE_CURVE ( 'NONE', #5159, #13568, #12686, .T. ) ;
#3819=VERTEX_POINT ( 'NONE', #10193 ) ;
#3820=DIRECTION ( 'NONE',  ( 0.000000000000000000, 0.000000000000000000, 1.000000000000000000 ) ) ;
#3821=ORIENTED_EDGE ( 'NONE', *, *, #8150, .F. ) ;
#3822=DIRECTION ( 'NONE',  ( 0.000000000000000000, 0.000000000000000000, -1.000000000000000000 ) ) ;
#3823=CARTESIAN_POINT ( 'NONE',  ( 72.70695371924547601, 57.06275842387054098, -13.00000000000000178 ) ) ;
#3824=CARTESIAN_POINT ( 'NONE',  ( 89.61631465359468507, -37.12029293941410657, 10.49999999999999822 ) ) ;
#3825=CARTESIAN_POINT ( 'NONE',  ( -30.80502811811232888, -49.00442420935981147, -10.50000000000000000 ) ) ;
#3826=VERTEX_POINT ( 'NONE', #11506 ) ;
#3827=DIRECTION ( 'NONE',  ( 0.000000000000000000, 0.000000000000000000, -1.000000000000000000 ) ) ;
#3828=ORIENTED_EDGE ( 'NONE', *, *, #4231, .F. ) ;
#3830=CARTESIAN_POINT ( 'NONE',  ( -45.91029614918924295, 26.00011991137363765, 10.49999999999999822 ) ) ;
#3831=DIRECTION ( 'NONE',  ( -0.000000000000000000, -0.000000000000000000, -1.000000000000000000 ) ) ;
#3832=DIRECTION ( 'NONE',  ( 1.000000000000000000, 0.000000000000000000, 0.000000000000000000 ) ) ;
#3833=AXIS2_PLACEMENT_3D ( 'NONE', #6803, #7947, #4108 ) ;
#3835=PLANE ( 'NONE',  #10577 ) ;
#3836=DIRECTION ( 'NONE',  ( 0.000000000000000000, 0.000000000000000000, 1.000000000000000000 ) ) ;
#3837=LINE ( 'NONE', #2696, #10966 ) ;
#3838=EDGE_CURVE ( 'NONE', #6551, #9479, #5643, .T. ) ;
#3840=EDGE_LOOP ( 'NONE', ( #7818, #5429, #4501, #10790 ) ) ;
#3841=CYLINDRICAL_SURFACE ( 'NONE', #7284, 63.00000000000000000 ) ;
#3842=VERTEX_POINT ( 'NONE', #3448 ) ;
#3843=DIRECTION ( 'NONE',  ( 0.000000000000000000, 0.000000000000000000, -1.000000000000000000 ) ) ;
#3844=ORIENTED_EDGE ( 'NONE', *, *, #275, .T. ) ;
#3845=DIRECTION ( 'NONE',  ( 1.000000000000000000, 0.000000000000000000, 0.000000000000000000 ) ) ;
#3851=DIRECTION ( 'NONE',  ( 0.000000000000000000, 0.000000000000000000, 1.000000000000000000 ) ) ;
#3852=CARTESIAN_POINT ( 'NONE',  ( 56.43380494353997534, 12.86891638962136319, -10.50000000000000000 ) ) ;
#3855=ADVANCED_FACE ( 'NONE', ( #11346 ), #14990, .F. ) ;
#3856=EDGE_LOOP ( 'NONE', ( #6831, #9459, #13273, #1873, #12208, #4144, #13395 ) ) ;
#3857=ORIENTED_EDGE ( 'NONE', *, *, #2547, .F. ) ;
#3858=DIRECTION ( 'NONE',  ( 1.000000000000000000, 0.000000000000000000, -0.000000000000000000 ) ) ;
#3860=ADVANCED_FACE ( 'NONE', ( #13931 ), #4659, .T. ) ;
#3861=DIRECTION ( 'NONE',  ( 0.000000000000000000, 0.000000000000000000, 1.000000000000000000 ) ) ;
#3862=CARTESIAN_POINT ( 'NONE',  ( -0.2790467552932288098, -97.41488903138106537, -10.50000000000000000 ) ) ;
#3863=FACE_OUTER_BOUND ( 'NONE', #3094, .T. ) ;
#3864=AXIS2_PLACEMENT_3D ( 'NONE', #10114, #14756, #4354 ) ;
#3865=ORIENTED_EDGE ( 'NONE', *, *, #1431, .T. ) ;
#3866=DIRECTION ( 'NONE',  ( 1.000000000000000000, 0.000000000000000000, 0.000000000000000000 ) ) ;
#3867=FACE_OUTER_BOUND ( 'NONE', #14651, .T. ) ;
#3868=ORIENTED_EDGE ( 'NONE', *, *, #302, .F. ) ;
#3869=FACE_OUTER_BOUND ( 'NONE', #13705, .T. ) ;
#3872=ORIENTED_EDGE ( 'NONE', *, *, #3993, .F. ) ;
#3873=CARTESIAN_POINT ( 'NONE',  ( -33.48561063518626923, 47.21331623427104063, -13.00000000000000178 ) ) ;
#3874=AXIS2_PLACEMENT_3D ( 'NONE', #12070, #11924, #5155 ) ;
#3875=DIRECTION ( 'NONE',  ( -0.000000000000000000, -0.000000000000000000, -1.000000000000000000 ) ) ;
#3876=ADVANCED_FACE ( 'NONE', ( #12706 ), #12558, .T. ) ;
#3877=ORIENTED_EDGE ( 'NONE', *, *, #10834, .F. ) ;
#3879=EDGE_CURVE ( 'NONE', #7182, #1468, #8792, .T. ) ;
#3880=LINE ( 'NONE', #14275, #11766 ) ;
#3881=DIRECTION ( 'NONE',  ( 0.000000000000000000, 0.000000000000000000, 1.000000000000000000 ) ) ;
#3882=CARTESIAN_POINT ( 'NONE',  ( -45.89934640057513349, 26.50000000000019540, -13.00000000000000178 ) ) ;
#3884=CIRCLE ( 'NONE', #9678, 100.0000000000000000 ) ;
#3885=DIRECTION ( 'NONE',  ( 0.000000000000000000, 0.000000000000000000, -1.000000000000000000 ) ) ;
#3887=EDGE_CURVE ( 'NONE', #14486, #2928, #3526, .T. ) ;
#3888=AXIS2_PLACEMENT_3D ( 'NONE', #2899, #1624, #11807 ) ;
#3890=VERTEX_POINT ( 'NONE', #9354 ) ;
#3891=AXIS2_PLACEMENT_3D ( 'NONE', #5993, #536, #8432 ) ;
#3894=FACE_OUTER_BOUND ( 'NONE', #14344, .T. ) ;
#3896=AXIS2_PLACEMENT_3D ( 'NONE', #4947, #11938, #8494 ) ;
#3897=DIRECTION ( 'NONE',  ( -0.000000000000000000, -0.000000000000000000, -1.000000000000000000 ) ) ;
#3898=ADVANCED_FACE ( 'NONE', ( #3298 ), #6760, .T. ) ;
#3899=ORIENTED_EDGE ( 'NONE', *, *, #4764, .T. ) ;
#3900=DIRECTION ( 'NONE',  ( -1.000000000000000000, 0.000000000000000000, 0.000000000000000000 ) ) ;
#3902=ORIENTED_EDGE ( 'NONE', *, *, #131, .F. ) ;
#3903=AXIS2_PLACEMENT_3D ( 'NONE', #14115, #3798, #12902 ) ;
#3904=DIRECTION ( 'NONE',  ( 1.000000000000000000, 0.000000000000000000, 0.000000000000000000 ) ) ;
#3906=LINE ( 'NONE', #1626, #13572 ) ;
#3912=CIRCLE ( 'NONE', #1489, 0.5000000000000004441 ) ;
#3913=CYLINDRICAL_SURFACE ( 'NONE', #7642, 60.50000000000000000 ) ;
#3914=CYLINDRICAL_SURFACE ( 'NONE', #10489, 0.5000000000000022204 ) ;
#3916=ORIENTED_EDGE ( 'NONE', *, *, #6890, .T. ) ;
#3918=VERTEX_POINT ( 'NONE', #5640 ) ;
#3920=CARTESIAN_POINT ( 'NONE',  ( -34.12029293941441210, -89.61631465359452875, -8.000000000000000000 ) ) ;
#3922=AXIS2_PLACEMENT_3D ( 'NONE', #2838, #8524, #7450 ) ;
#3925=LINE ( 'NONE', #1567, #6597 ) ;
#3927=FACE_OUTER_BOUND ( 'NONE', #11718, .T. ) ;
#3928=ORIENTED_EDGE ( 'NONE', *, *, #2548, .T. ) ;
#3930=CYLINDRICAL_SURFACE ( 'NONE', #12734, 3.000000000000002665 ) ;
#3931=DIRECTION ( 'NONE',  ( 1.000000000000000000, 0.000000000000000000, 0.000000000000000000 ) ) ;
#3932=AXIS2_PLACEMENT_3D ( 'NONE', #3138, #5420, #10269 ) ;
#3934=ORIENTED_EDGE ( 'NONE', *, *, #5280, .T. ) ;
#3935=ORIENTED_EDGE ( 'NONE', *, *, #14014, .T. ) ;
#3936=CYLINDRICAL_SURFACE ( 'NONE', #14676, 59.50000000000000000 ) ;
#3937=ORIENTED_EDGE ( 'NONE', *, *, #2437, .T. ) ;
#3938=CYLINDRICAL_SURFACE ( 'NONE', #7277, 60.50000000000000000 ) ;
#3940=ADVANCED_FACE ( 'NONE', ( #3894 ), #466, .F. ) ;
#3942=SURFACE_STYLE_USAGE ( .BOTH. , #14334 ) ;
#3943=EDGE_CURVE ( 'NONE', #3062, #1186, #11722, .T. ) ;
#3944=EDGE_CURVE ( 'NONE', #5657, #4604, #13409, .T. ) ;
#3945=DIRECTION ( 'NONE',  ( 0.000000000000000000, 0.000000000000000000, 1.000000000000000000 ) ) ;
#3946=CARTESIAN_POINT ( 'NONE',  ( -52.54657765281192638, 6.917888187662934563, -8.000000000000000000 ) ) ;
#3947=CIRCLE ( 'NONE', #12671, 100.0000000000000000 ) ;
#3949=DIRECTION ( 'NONE',  ( 0.000000000000000000, 0.000000000000000000, 1.000000000000000000 ) ) ;
#3950=ORIENTED_EDGE ( 'NONE', *, *, #13497, .T. ) ;
#3952=ORIENTED_EDGE ( 'NONE', *, *, #14952, .F. ) ;
#3953=CARTESIAN_POINT ( 'NONE',  ( -34.62083247296263266, -87.95718916809180143, 8.000000000000000000 ) ) ;
#3955=CIRCLE ( 'NONE', #5879, 2.649999999999985700 ) ;
#3957=DIRECTION ( 'NONE',  ( 1.000000000000000000, 0.000000000000000000, 0.000000000000000000 ) ) ;
#3958=DIRECTION ( 'NONE',  ( -0.5000000000000009992, 0.000000000000000000, 0.8660254037844380415 ) ) ;
#3959=DIRECTION ( 'NONE',  ( -1.000000000000000000, 0.000000000000000000, 0.000000000000000000 ) ) ;
#3961=ORIENTED_EDGE ( 'NONE', *, *, #593, .T. ) ;
#3962=DIRECTION ( 'NONE',  ( 1.000000000000000000, 0.000000000000000000, 0.000000000000000000 ) ) ;
#3963=VECTOR ( 'NONE', #9131, 1000.000000000000000 ) ;
#3965=EDGE_CURVE ( 'NONE', #1743, #2090, #7825, .T. ) ;
#3966=CARTESIAN_POINT ( 'NONE',  ( -48.29629131445344115, -12.94095225512594816, 8.000000000000000000 ) ) ;
#3967=FACE_OUTER_BOUND ( 'NONE', #5721, .T. ) ;
#3968=AXIS2_PLACEMENT_3D ( 'NONE', #6996, #3373, #10359 ) ;
#3972=AXIS2_PLACEMENT_3D ( 'NONE', #5545, #6742, #4341 ) ;
#3974=CARTESIAN_POINT ( 'NONE',  ( 34.62083247296202160, 87.95718916809205723, -13.00000000000000178 ) ) ;
#3975=VERTEX_POINT ( 'NONE', #14144 ) ;
#3976=CARTESIAN_POINT ( 'NONE',  ( -42.64958156413675994, -32.39328945492002276, -10.50000000000000000 ) ) ;
#3979=CARTESIAN_POINT ( 'NONE',  ( 0.000000000000000000, 0.000000000000000000, -10.50000000000000000 ) ) ;
#3981=DIRECTION ( 'NONE',  ( -1.000000000000000000, 2.682261509073381941E-15, 0.000000000000000000 ) ) ;
#3983=ORIENTED_EDGE ( 'NONE', *, *, #1243, .T. ) ;
#3984=EDGE_CURVE ( 'NONE', #1696, #12197, #6848, .T. ) ;
#3985=DIRECTION ( 'NONE',  ( 0.000000000000000000, 0.000000000000000000, 1.000000000000000000 ) ) ;
#3988=AXIS2_PLACEMENT_3D ( 'NONE', #12783, #4580, #7141 ) ;
#3990=AXIS2_PLACEMENT_3D ( 'NONE', #5179, #2892, #11253 ) ;
#3991=AXIS2_PLACEMENT_3D ( 'NONE', #11073, #7712, #11303 ) ;
#3993=EDGE_CURVE ( 'NONE', #215, #6594, #6348, .T. ) ;
#3995=ORIENTED_EDGE ( 'NONE', *, *, #12207, .F. ) ;
#3998=CIRCLE ( 'NONE', #2778, 60.50000000000000000 ) ;
#3999=DIRECTION ( 'NONE',  ( 1.000000000000000000, 0.000000000000000000, 0.000000000000000000 ) ) ;
#4002=CARTESIAN_POINT ( 'NONE',  ( -51.19406879332065330, -13.71740939043347041, 10.49999999999999822 ) ) ;
#4007=DIRECTION ( 'NONE',  ( -1.000000000000000000, 0.000000000000000000, 0.000000000000000000 ) ) ;
#4008=CARTESIAN_POINT ( 'NONE',  ( -45.88839665196098849, 26.99988008862674960, -10.50000000000000000 ) ) ;
#4013=CIRCLE ( 'NONE', #7879, 50.00000000000000000 ) ;
#4015=DIRECTION ( 'NONE',  ( 1.000000000000000000, 0.000000000000000000, 0.000000000000000000 ) ) ;
#4018=AXIS2_PLACEMENT_3D ( 'NONE', #4099, #6212, #12149 ) ;
#4019=DIRECTION ( 'NONE',  ( -0.000000000000000000, -0.000000000000000000, -1.000000000000000000 ) ) ;
#4020=LINE ( 'NONE', #13278, #10457 ) ;
#4021=ORIENTED_EDGE ( 'NONE', *, *, #4242, .F. ) ;
#4022=DIRECTION ( 'NONE',  ( 1.000000000000000000, 0.000000000000000000, 0.000000000000000000 ) ) ;
#4023=AXIS2_PLACEMENT_3D ( 'NONE', #10094, #7889, #12229 ) ;
#4024=ORIENTED_EDGE ( 'NONE', *, *, #6547, .F. ) ;
#4026=ORIENTED_EDGE ( 'NONE', *, *, #6810, .F. ) ;
#4028=EDGE_CURVE ( 'NONE', #5501, #7998, #13908, .T. ) ;
#4029=AXIS2_PLACEMENT_3D ( 'NONE', #6873, #10377, #6111 ) ;
#4033=DIRECTION ( 'NONE',  ( 1.000000000000000000, 0.000000000000000000, 0.000000000000000000 ) ) ;
#4034=DIRECTION ( 'NONE',  ( -1.000000000000000000, 0.000000000000000000, 0.000000000000000000 ) ) ;
#4038=AXIS2_PLACEMENT_3D ( 'NONE', #10815, #415, #10735 ) ;
#4043=CARTESIAN_POINT ( 'NONE',  ( 0.000000000000000000, 0.000000000000000000, 8.000000000000000000 ) ) ;
#4045=EDGE_LOOP ( 'NONE', ( #12281, #7377, #11151, #9153, #6403 ) ) ;
#4046=LINE ( 'NONE', #11402, #4985 ) ;
#4049=DIRECTION ( 'NONE',  ( -1.000000000000000000, 0.000000000000000000, -0.000000000000000000 ) ) ;
#4053=VERTEX_POINT ( 'NONE', #9639 ) ;
#4054=ORIENTED_EDGE ( 'NONE', *, *, #10702, .T. ) ;
#4056=CARTESIAN_POINT ( 'NONE',  ( -51.19406879332065330, -13.71740939043347041, -13.00000000000000178 ) ) ;
#4057=DIRECTION ( 'NONE',  ( 0.000000000000000000, 0.000000000000000000, 1.000000000000000000 ) ) ;
#4058=DIRECTION ( 'NONE',  ( 1.000000000000000000, 0.000000000000000000, 0.000000000000000000 ) ) ;
#4060=CARTESIAN_POINT ( 'NONE',  ( 50.84834283436990177, 14.07862063237912054, 10.49999999999999822 ) ) ;
#4063=CARTESIAN_POINT ( 'NONE',  ( 0.000000000000000000, 0.000000000000000000, -8.000000000000000000 ) ) ;
#4067=CARTESIAN_POINT ( 'NONE',  ( -42.04772703543551415, -32.26435573746212526, -10.50000000000000000 ) ) ;
#4068=EDGE_CURVE ( 'NONE', #4159, #3184, #4749, .T. ) ;
#4069=EDGE_CURVE ( 'NONE', #5810, #10576, #8128, .T. ) ;
#4070=VERTEX_POINT ( 'NONE', #11868 ) ;
#4071=ADVANCED_FACE ( 'NONE', ( #1461 ), #325, .F. ) ;
#4073=DIRECTION ( 'NONE',  ( 0.000000000000000000, 0.000000000000000000, 1.000000000000000000 ) ) ;
#4075=CARTESIAN_POINT ( 'NONE',  ( 52.72775723226780542, -7.383907457637739036, 10.49999999999999822 ) ) ;
#4076=FACE_OUTER_BOUND ( 'NONE', #4280, .T. ) ;
#4079=EDGE_CURVE ( 'NONE', #3301, #8551, #14927, .T. ) ;
#4081=DIRECTION ( 'NONE',  ( -1.000000000000000000, 1.765157221169382931E-15, 0.000000000000000000 ) ) ;
#4082=CARTESIAN_POINT ( 'NONE',  ( -68.58935777509570642, -68.58935777509452691, 10.49999999999999822 ) ) ;
#4083=ORIENTED_EDGE ( 'NONE', *, *, #892, .T. ) ;
#4086=ORIENTED_EDGE ( 'NONE', *, *, #2224, .T. ) ;
#4087=EDGE_CURVE ( 'NONE', #6876, #836, #12747, .T. ) ;
#4088=ORIENTED_EDGE ( 'NONE', *, *, #6673, .F. ) ;
#4089=EDGE_CURVE ( 'NONE', #12422, #6857, #10026, .T. ) ;
#4091=DIRECTION ( 'NONE',  ( -1.000000000000000000, 0.000000000000000000, 0.000000000000000000 ) ) ;
#4093=LINE ( 'NONE', #13346, #7530 ) ;
#4094=CARTESIAN_POINT ( 'NONE',  ( 51.19406879332056093, 13.71740939043382745, -8.000000000000000000 ) ) ;
#4095=ORIENTED_EDGE ( 'NONE', *, *, #3710, .F. ) ;
#4097=ORIENTED_EDGE ( 'NONE', *, *, #4865, .F. ) ;
#4098=ORIENTED_EDGE ( 'NONE', *, *, #3365, .T. ) ;
#4099=CARTESIAN_POINT ( 'NONE',  ( -33.48561063518626923, 47.21331623427104063, 10.49999999999999822 ) ) ;
#4101=DIRECTION ( 'NONE',  ( 0.000000000000000000, 0.000000000000000000, 1.000000000000000000 ) ) ;
#4103=DIRECTION ( 'NONE',  ( 1.000000000000000000, 0.000000000000000000, 0.000000000000000000 ) ) ;
#4108=DIRECTION ( 'NONE',  ( 1.000000000000000000, 0.000000000000000000, 0.000000000000000000 ) ) ;
#4114=EDGE_LOOP ( 'NONE', ( #7332, #4858, #3950, #4964 ) ) ;
#4116=VERTEX_POINT ( 'NONE', #3125 ) ;
#4117=CARTESIAN_POINT ( 'NONE',  ( -2.449293598294700991E-16, 97.00000000000000000, 8.000000000000000000 ) ) ;
#4119=ORIENTED_EDGE ( 'NONE', *, *, #8284, .F. ) ;
#4120=CIRCLE ( 'NONE', #4609, 3.000000000000002665 ) ;
#4121=DIRECTION ( 'NONE',  ( -1.000000000000000000, 0.000000000000000000, 0.000000000000000000 ) ) ;
#4122=CARTESIAN_POINT ( 'NONE',  ( 33.48561063518626923, -47.21331623427104063, -8.000000000000000000 ) ) ;
#4125=FACE_OUTER_BOUND ( 'NONE', #7137, .T. ) ;
#4127=CIRCLE ( 'NONE', #6044, 53.55662432702593634 ) ;
#4128=FACE_OUTER_BOUND ( 'NONE', #13282, .T. ) ;
#4130=EDGE_CURVE ( 'NONE', #14448, #10153, #4263, .T. ) ;
#4132=ORIENTED_EDGE ( 'NONE', *, *, #10811, .F. ) ;
#4134=ORIENTED_EDGE ( 'NONE', *, *, #883, .F. ) ;
#4135=CARTESIAN_POINT ( 'NONE',  ( 57.06275842387049835, -9.706953719245678514, 10.49999999999999822 ) ) ;
#4136=CIRCLE ( 'NONE', #14561, 50.00000000000000000 ) ;
#4138=AXIS2_PLACEMENT_3D ( 'NONE', #11109, #5418, #2984 ) ;
#4139=EDGE_CURVE ( 'NONE', #7269, #6876, #7443, .T. ) ;
#4140=AXIS2_PLACEMENT_3D ( 'NONE', #4812, #3602, #9423 ) ;
#4144=ORIENTED_EDGE ( 'NONE', *, *, #8764, .F. ) ;
#4145=CARTESIAN_POINT ( 'NONE',  ( 68.58935777509475429, -68.58935777509547904, -8.000000000000000000 ) ) ;
#4149=DIRECTION ( 'NONE',  ( -0.000000000000000000, -0.000000000000000000, -1.000000000000000000 ) ) ;
#4152=CIRCLE ( 'NONE', #4874, 3.000000000000002665 ) ;
#4154=CIRCLE ( 'NONE', #12632, 100.0000000000000000 ) ;
#4155=DIRECTION ( 'NONE',  ( -1.000000000000000000, 0.000000000000000000, 0.000000000000000000 ) ) ;
#4156=CYLINDRICAL_SURFACE ( 'NONE', #14999, 60.50000000000000000 ) ;
#4159=VERTEX_POINT ( 'NONE', #14599 ) ;
#4160=VECTOR ( 'NONE', #13756, 1000.000000000000000 ) ;
#4161=CIRCLE ( 'NONE', #8748, 3.000000000000004441 ) ;
#4163=ORIENTED_EDGE ( 'NONE', *, *, #9533, .F. ) ;
#4164=ORIENTED_EDGE ( 'NONE', *, *, #8305, .T. ) ;
#4167=CIRCLE ( 'NONE', #8753, 3.000000000000002665 ) ;
#4169=MANIFOLD_SOLID_BREP ( 'Cut-Extrude1', #8911 ) ;
#4174=CARTESIAN_POINT ( 'NONE',  ( -9.714003807513870825, -53.63365512954690217, -13.00000000000000178 ) ) ;
#4175=CIRCLE ( 'NONE', #14847, 3.000000000000002665 ) ;
#4176=CARTESIAN_POINT ( 'NONE',  ( -31.76435573746199381, 42.04772703543562073, -10.50000000000000000 ) ) ;
#4177=ORIENTED_EDGE ( 'NONE', *, *, #7858, .F. ) ;
#4179=EDGE_CURVE ( 'NONE', #12800, #8993, #4046, .T. ) ;
#4181=CIRCLE ( 'NONE', #5387, 3.000000000000002665 ) ;
#4182=ORIENTED_EDGE ( 'NONE', *, *, #6193, .T. ) ;
#4183=VERTEX_POINT ( 'NONE', #13761 ) ;
#4188=AXIS2_PLACEMENT_3D ( 'NONE', #8301, #8154, #9361 ) ;
#4190=DIRECTION ( 'NONE',  ( 0.000000000000000000, 0.000000000000000000, -1.000000000000000000 ) ) ;
#4191=DIRECTION ( 'NONE',  ( -0.000000000000000000, -0.000000000000000000, -1.000000000000000000 ) ) ;
#4192=ORIENTED_EDGE ( 'NONE', *, *, #11689, .F. ) ;
#4195=ADVANCED_FACE ( 'NONE', ( #1003 ), #931, .F. ) ;
#4199=ORIENTED_EDGE ( 'NONE', *, *, #4449, .F. ) ;
#4200=FACE_BOUND ( 'NONE', #461, .T. ) ;
#4202=DIRECTION ( 'NONE',  ( 1.000000000000000000, 0.000000000000000000, 0.000000000000000000 ) ) ;
#4204=CIRCLE ( 'NONE', #14633, 100.0000000000000000 ) ;
#4206=DIRECTION ( 'NONE',  ( 1.000000000000000000, 0.000000000000000000, 0.000000000000000000 ) ) ;
#4207=FACE_OUTER_BOUND ( 'NONE', #3405, .T. ) ;
#4209=DIRECTION ( 'NONE',  ( -0.000000000000000000, -0.000000000000000000, 1.000000000000000000 ) ) ;
#4210=FACE_OUTER_BOUND ( 'NONE', #11307, .T. ) ;
#4211=CARTESIAN_POINT ( 'NONE',  ( 0.000000000000000000, 0.000000000000000000, 13.00000000000000178 ) ) ;
#4212=CIRCLE ( 'NONE', #8797, 50.00000000000000000 ) ;
#4213=ORIENTED_EDGE ( 'NONE', *, *, #13274, .T. ) ;
#4214=CARTESIAN_POINT ( 'NONE',  ( 0.000000000000000000, 0.000000000000000000, -10.50000000000000000 ) ) ;
#4215=DIRECTION ( 'NONE',  ( 1.000000000000000000, 0.000000000000000000, 0.000000000000000000 ) ) ;
#4219=ORIENTED_EDGE ( 'NONE', *, *, #10261, .T. ) ;
#4220=ADVANCED_FACE ( 'NONE', ( #9184 ), #13679, .T. ) ;
#4221=DIRECTION ( 'NONE',  ( -1.000000000000000000, 0.000000000000000000, 0.000000000000000000 ) ) ;
#4223=ORIENTED_EDGE ( 'NONE', *, *, #8070, .F. ) ;
#4224=CARTESIAN_POINT ( 'NONE',  ( 89.61631465359491244, 37.12029293941346708, 8.000000000000000000 ) ) ;
#4225=CARTESIAN_POINT ( 'NONE',  ( 100.0000000000000000, -3.384287605079545030E-13, -13.00000000000000178 ) ) ;
#4226=ORIENTED_EDGE ( 'NONE', *, *, #9758, .T. ) ;
#4227=FACE_OUTER_BOUND ( 'NONE', #14959, .T. ) ;
#4228=DIRECTION ( 'NONE',  ( -1.000000000000000000, 0.000000000000000000, 0.000000000000000000 ) ) ;
#4231=EDGE_CURVE ( 'NONE', #15024, #1076, #1590, .T. ) ;
#4232=ORIENTED_EDGE ( 'NONE', *, *, #12259, .T. ) ;
#4233=ORIENTED_EDGE ( 'NONE', *, *, #1565, .F. ) ;
#4234=AXIS2_PLACEMENT_3D ( 'NONE', #3363, #12631, #6847 ) ;
#4237=CIRCLE ( 'NONE', #5444, 0.5000000000000073275 ) ;
#4238=ADVANCED_FACE ( 'NONE', ( #2060 ), #11332, .T. ) ;
#4241=EDGE_LOOP ( 'NONE', ( #10390, #10211, #6704, #8900, #10020 ) ) ;
#4242=EDGE_CURVE ( 'NONE', #10287, #8196, #11297, .T. ) ;
#4243=ORIENTED_EDGE ( 'NONE', *, *, #4068, .T. ) ;
#4244=AXIS2_PLACEMENT_3D ( 'NONE', #6879, #8026, #1139 ) ;
#4246=CIRCLE ( 'NONE', #5927, 63.00000000000000000 ) ;
#4247=LINE ( 'NONE', #6418, #14638 ) ;
#4250=FACE_BOUND ( 'NONE', #1571, .T. ) ;
#4252=ORIENTED_EDGE ( 'NONE', *, *, #14625, .T. ) ;
#4254=CIRCLE ( 'NONE', #7624, 50.00000000000000000 ) ;
#4256=AXIS2_PLACEMENT_3D ( 'NONE', #6938, #8082, #185 ) ;
#4259=ORIENTED_EDGE ( 'NONE', *, *, #5315, .F. ) ;
#4261=DIRECTION ( 'NONE',  ( -1.000000000000000000, 0.000000000000000000, 0.000000000000000000 ) ) ;
#4262=EDGE_CURVE ( 'NONE', #12963, #1264, #14690, .T. ) ;
#4263=CIRCLE ( 'NONE', #2061, 3.000000000000002665 ) ;
#4266=FACE_OUTER_BOUND ( 'NONE', #8321, .T. ) ;
#4269=EDGE_CURVE ( 'NONE', #7351, #1743, #9115, .T. ) ;
#4271=DIRECTION ( 'NONE',  ( 0.000000000000000000, 0.000000000000000000, 1.000000000000000000 ) ) ;
#4272=CIRCLE ( 'NONE', #5710, 3.000000000000002665 ) ;
#4273=ADVANCED_FACE ( 'NONE', ( #12612 ), #2207, .T. ) ;
#4275=DIRECTION ( 'NONE',  ( 0.000000000000000000, 0.000000000000000000, -1.000000000000000000 ) ) ;
#4276=CIRCLE ( 'NONE', #1126, 59.50000000000000000 ) ;
#4277=EDGE_LOOP ( 'NONE', ( #2716, #1135 ) ) ;
#4278=ORIENTED_EDGE ( 'NONE', *, *, #6612, .F. ) ;
#4280=EDGE_LOOP ( 'NONE', ( #9167, #14516, #11601, #671 ) ) ;
#4281=DIRECTION ( 'NONE',  ( 1.000000000000000000, 0.000000000000000000, 0.000000000000000000 ) ) ;
#4282=ORIENTED_EDGE ( 'NONE', *, *, #7255, .T. ) ;
#4283=ADVANCED_FACE ( 'NONE', ( #12690 ), #5697, .F. ) ;
#4284=ORIENTED_EDGE ( 'NONE', *, *, #2023, .F. ) ;
#4286=DIRECTION ( 'NONE',  ( 0.000000000000000000, 0.000000000000000000, 1.000000000000000000 ) ) ;
#4288=CIRCLE ( 'NONE', #7661, 0.5000000000000022204 ) ;
#4289=CYLINDRICAL_SURFACE ( 'NONE', #8000, 3.000000000000002665 ) ;
#4290=DIRECTION ( 'NONE',  ( 0.000000000000000000, 0.000000000000000000, 1.000000000000000000 ) ) ;
#4291=CARTESIAN_POINT ( 'NONE',  ( 44.13108361037843252, 56.43380494353993271, -13.00000000000000178 ) ) ;
#4292=EDGE_LOOP ( 'NONE', ( #13559, #14263 ) ) ;
#4293=CARTESIAN_POINT ( 'NONE',  ( -7.252293700257136599, -53.06332297728250325, -10.50000000000000000 ) ) ;
#4295=CARTESIAN_POINT ( 'NONE',  ( 47.21331623427115431, 33.48561063518610581, -10.50000000000000000 ) ) ;
#4296=CIRCLE ( 'NONE', #403, 59.50000000000000000 ) ;
#4298=DIRECTION ( 'NONE',  ( 0.000000000000000000, 0.000000000000000000, -1.000000000000000000 ) ) ;
#4299=ORIENTED_EDGE ( 'NONE', *, *, #5268, .F. ) ;
#4301=ORIENTED_EDGE ( 'NONE', *, *, #13152, .F. ) ;
#4302=DIRECTION ( 'NONE',  ( 1.000000000000000000, 0.000000000000000000, 0.000000000000000000 ) ) ;
#4305=LINE ( 'NONE', #7467, #11241 ) ;
#4306=PRODUCT_CONTEXT ( 'NONE', #9976, 'mechanical' ) ;
#4308=ORIENTED_EDGE ( 'NONE', *, *, #1084, .T. ) ;
#4309=ORIENTED_EDGE ( 'NONE', *, *, #10723, .F. ) ;
#4310=ADVANCED_FACE ( 'NONE', ( #10402 ), #2287, .T. ) ;
#4311=DIRECTION ( 'NONE',  ( 0.000000000000000000, 0.000000000000000000, 1.000000000000000000 ) ) ;
#4312=LINE ( 'NONE', #1940, #6171 ) ;
#4313=ADVANCED_FACE ( 'NONE', ( #12769 ), #2353, .T. ) ;
#4314=DIRECTION ( 'NONE',  ( 1.000000000000000000, 0.000000000000000000, 0.000000000000000000 ) ) ;
#4316=ORIENTED_EDGE ( 'NONE', *, *, #5960, .F. ) ;
#4317=ORIENTED_EDGE ( 'NONE', *, *, #13624, .F. ) ;
#4318=CARTESIAN_POINT ( 'NONE',  ( 6.917888187663118416, 52.54657765281190507, 8.000000000000000000 ) ) ;
#4319=DIRECTION ( 'NONE',  ( 0.000000000000000000, 0.000000000000000000, 1.000000000000000000 ) ) ;
#4320=SHAPE_REPRESENTATION_RELATIONSHIP ( 'NONE' , 'NONE' ,  #8100, #7823 ) ;
#4321=DIRECTION ( 'NONE',  ( 0.000000000000000000, 0.000000000000000000, 1.000000000000000000 ) ) ;
#4322=EDGE_LOOP ( 'NONE', ( #7996, #14796, #7899, #6022 ) ) ;
#4323=DIRECTION ( 'NONE',  ( 0.000000000000000000, 0.000000000000000000, 1.000000000000000000 ) ) ;
#4324=CARTESIAN_POINT ( 'NONE',  ( -2.449293598294700991E-16, 97.00000000000000000, -8.000000000000000000 ) ) ;
#4326=EDGE_CURVE ( 'NONE', #8856, #10004, #3279, .T. ) ;
#4328=CARTESIAN_POINT ( 'NONE',  ( -49.00442420935969778, 30.80502811811250297, -10.50000000000000000 ) ) ;
#4330=ORIENTED_EDGE ( 'NONE', *, *, #4410, .F. ) ;
#4331=VERTEX_POINT ( 'NONE', #2582 ) ;
#4333=ORIENTED_EDGE ( 'NONE', *, *, #9911, .T. ) ;
#4335=PLANE ( 'NONE',  #11047 ) ;
#4336=CARTESIAN_POINT ( 'NONE',  ( -37.12029293941441210, -89.61631465359452875, 10.49999999999999822 ) ) ;
#4338=VERTEX_POINT ( 'NONE', #14270 ) ;
#4339=CIRCLE ( 'NONE', #5056, 53.55662432702593634 ) ;
#4340=FACE_OUTER_BOUND ( 'NONE', #4898, .T. ) ;
#4341=DIRECTION ( 'NONE',  ( 1.000000000000000000, 0.000000000000000000, 0.000000000000000000 ) ) ;
#4342=CARTESIAN_POINT ( 'NONE',  ( 0.000000000000000000, 0.000000000000000000, -10.50000000000000000 ) ) ;
#4343=EDGE_CURVE ( 'NONE', #10098, #7516, #2549, .T. ) ;
#4344=ORIENTED_EDGE ( 'NONE', *, *, #1434, .F. ) ;
#4345=CARTESIAN_POINT ( 'NONE',  ( -33.48561063518626923, 47.21331623427104063, 10.49999999999999822 ) ) ;
#4346=FACE_BOUND ( 'NONE', #108, .T. ) ;
#4347=EDGE_CURVE ( 'NONE', #3184, #11976, #4276, .T. ) ;
#4349=PLANE ( 'NONE',  #5101 ) ;
#4351=CARTESIAN_POINT ( 'NONE',  ( -0.2790467552932288098, -97.41488903138106537, 10.49999999999999822 ) ) ;
#4352=CARTESIAN_POINT ( 'NONE',  ( 89.33979373934423052, -36.70371619500547666, 10.49999999999999822 ) ) ;
#4353=EDGE_CURVE ( 'NONE', #2094, #11817, #5480, .T. ) ;
#4354=DIRECTION ( 'NONE',  ( 1.000000000000000000, 0.000000000000000000, 0.000000000000000000 ) ) ;
#4355=CARTESIAN_POINT ( 'NONE',  ( 90.11631465359468507, -37.12029293941410657, -13.00000000000000178 ) ) ;
#4356=DIRECTION ( 'NONE',  ( 1.000000000000000000, 0.000000000000000000, 0.000000000000000000 ) ) ;
#4357=ORIENTED_EDGE ( 'NONE', *, *, #4600, .T. ) ;
#4360=EDGE_CURVE ( 'NONE', #6631, #197, #8607, .T. ) ;
#4361=EDGE_CURVE ( 'NONE', #9608, #4909, #14441, .T. ) ;
#4364=DIRECTION ( 'NONE',  ( 1.000000000000000000, 0.000000000000000000, 0.000000000000000000 ) ) ;
#4366=CARTESIAN_POINT ( 'NONE',  ( -68.58935777509570642, -68.58935777509452691, -8.000000000000000000 ) ) ;
#4367=AXIS2_PLACEMENT_3D ( 'NONE', #13667, #8877, #3268 ) ;
#4368=ORIENTED_EDGE ( 'NONE', *, *, #10013, .T. ) ;
#4369=CARTESIAN_POINT ( 'NONE',  ( 6.917888187663118416, 52.54657765281190507, -10.50000000000000000 ) ) ;
#4371=ADVANCED_FACE ( 'NONE', ( #10478 ), #13986, .T. ) ;
#4374=CARTESIAN_POINT ( 'NONE',  ( -30.80502811811232888, -49.00442420935981147, -10.50000000000000000 ) ) ;
#4376=EDGE_LOOP ( 'NONE', ( #9697, #237, #1688, #12590 ) ) ;
#4378=ORIENTED_EDGE ( 'NONE', *, *, #14291, .T. ) ;
#4379=VECTOR ( 'NONE', #6548, 1000.000000000000000 ) ;
#4380=DIRECTION ( 'NONE',  ( 1.000000000000000000, 0.000000000000000000, 0.000000000000000000 ) ) ;
#4381=CIRCLE ( 'NONE', #3888, 50.00000000000000000 ) ;
#4384=CARTESIAN_POINT ( 'NONE',  ( 47.21331623427115431, 33.48561063518610581, -13.00000000000000178 ) ) ;
#4386=EDGE_LOOP ( 'NONE', ( #11067, #3176, #8706, #2487 ) ) ;
#4389=DIRECTION ( 'NONE',  ( 0.000000000000000000, 0.000000000000000000, 1.000000000000000000 ) ) ;
#4391=CIRCLE ( 'NONE', #12146, 3.000000000000002665 ) ;
#4392=DIRECTION ( 'NONE',  ( 1.000000000000000000, 0.000000000000000000, 0.000000000000000000 ) ) ;
#4393=AXIS2_PLACEMENT_3D ( 'NONE', #1759, #11171, #8882 ) ;
#4396=VERTEX_POINT ( 'NONE', #9401 ) ;
#4397=CYLINDRICAL_SURFACE ( 'NONE', #6556, 3.000000000000002665 ) ;
#4398=DIRECTION ( 'NONE',  ( 0.000000000000000000, 0.000000000000000000, 1.000000000000000000 ) ) ;
#4399=ORIENTED_EDGE ( 'NONE', *, *, #13626, .T. ) ;
#4402=ORIENTED_EDGE ( 'NONE', *, *, #14358, .T. ) ;
#4403=AXIS2_PLACEMENT_3D ( 'NONE', #10594, #192, #14093 ) ;
#4404=AXIS2_PLACEMENT_3D ( 'NONE', #5050, #14307, #9737 ) ;
#4406=FACE_OUTER_BOUND ( 'NONE', #1195, .T. ) ;
#4409=ADVANCED_FACE ( 'NONE', ( #6350 ), #10924, .T. ) ;
#4410=EDGE_CURVE ( 'NONE', #6432, #6463, #2812, .T. ) ;
#4411=LINE ( 'NONE', #614, #14089 ) ;
#4412=DIRECTION ( 'NONE',  ( 0.000000000000000000, 0.000000000000000000, 1.000000000000000000 ) ) ;
#4417=CARTESIAN_POINT ( 'NONE',  ( 89.61631465359468507, -37.12029293941410657, -10.50000000000000000 ) ) ;
#4418=AXIS2_PLACEMENT_3D ( 'NONE', #10123, #6541, #4221 ) ;
#4420=DIRECTION ( 'NONE',  ( -0.000000000000000000, -0.000000000000000000, -1.000000000000000000 ) ) ;
#4421=ORIENTED_EDGE ( 'NONE', *, *, #4449, .T. ) ;
#4425=CARTESIAN_POINT ( 'NONE',  ( 37.12029293941315444, -89.61631465359504034, -13.00000000000000178 ) ) ;
#4426=AXIS2_PLACEMENT_3D ( 'NONE', #807, #1926, #6545 ) ;
#4428=DIRECTION ( 'NONE',  ( -0.000000000000000000, -0.000000000000000000, 1.000000000000000000 ) ) ;
#4429=CARTESIAN_POINT ( 'NONE',  ( -23.50071946824040836, -45.96504489226015977, 8.000000000000000000 ) ) ;
#4430=CARTESIAN_POINT ( 'NONE',  ( -12.86891638962156215, 56.43380494353993271, -8.000000000000000000 ) ) ;
#4431=LINE ( 'NONE', #5332, #9276 ) ;
#4432=DIRECTION ( 'NONE',  ( -0.000000000000000000, -0.000000000000000000, -1.000000000000000000 ) ) ;
#4433=EDGE_CURVE ( 'NONE', #6138, #13092, #3294, .T. ) ;
#4436=ORIENTED_EDGE ( 'NONE', *, *, #8388, .F. ) ;
#4437=AXIS2_PLACEMENT_3D ( 'NONE', #11659, #5650, #4525 ) ;
#4438=DIRECTION ( 'NONE',  ( -0.000000000000000000, -0.000000000000000000, -1.000000000000000000 ) ) ;
#4439=DIRECTION ( 'NONE',  ( 0.000000000000000000, 0.000000000000000000, 1.000000000000000000 ) ) ;
#4441=VERTEX_POINT ( 'NONE', #13507 ) ;
#4442=DIRECTION ( 'NONE',  ( 0.000000000000000000, 0.000000000000000000, -1.000000000000000000 ) ) ;
#4444=ORIENTED_EDGE ( 'NONE', *, *, #13821, .F. ) ;
#4449=EDGE_CURVE ( 'NONE', #669, #10819, #9822, .T. ) ;
#4451=CARTESIAN_POINT ( 'NONE',  ( -49.00442420935969778, 30.80502811811250297, -13.00000000000000178 ) ) ;
#4452=EDGE_CURVE ( 'NONE', #13716, #6488, #8864, .T. ) ;
#4453=FACE_OUTER_BOUND ( 'NONE', #8678, .T. ) ;
#4454=VERTEX_POINT ( 'NONE', #10851 ) ;
#4455=EDGE_CURVE ( 'NONE', #4704, #8488, #147, .T. ) ;
#4456=ORIENTED_EDGE ( 'NONE', *, *, #133, .F. ) ;
#4457=AXIS2_PLACEMENT_3D ( 'NONE', #12126, #12966, #1575 ) ;
#4458=CARTESIAN_POINT ( 'NONE',  ( 69.08935777509475429, -68.58935777509547904, -10.50000000000000000 ) ) ;
#4459=CARTESIAN_POINT ( 'NONE',  ( -37.21932736666205699, 89.12622059913296368, -10.50000000000000000 ) ) ;
#4460=DIRECTION ( 'NONE',  ( -1.000000000000000000, 0.000000000000000000, 0.000000000000000000 ) ) ;
#4461=EDGE_LOOP ( 'NONE', ( #14666, #6054, #587, #8306 ) ) ;
#4462=EDGE_CURVE ( 'NONE', #11994, #3488, #1669, .T. ) ;
#4463=CIRCLE ( 'NONE', #2758, 56.99999999999998579 ) ;
#4467=CARTESIAN_POINT ( 'NONE',  ( 45.91029614918936375, -26.00011991137331790, -10.50000000000000000 ) ) ;
#4468=DIRECTION ( 'NONE',  ( 0.000000000000000000, 0.000000000000000000, 1.000000000000000000 ) ) ;
#4470=CARTESIAN_POINT ( 'NONE',  ( 0.000000000000000000, 0.000000000000000000, 13.00000000000000178 ) ) ;
#4471=CARTESIAN_POINT ( 'NONE',  ( 0.000000000000000000, 0.000000000000000000, -10.50000000000000000 ) ) ;
#4474=ORIENTED_EDGE ( 'NONE', *, *, #3014, .F. ) ;
#4475=DIRECTION ( 'NONE',  ( 1.000000000000000000, 0.000000000000000000, 0.000000000000000000 ) ) ;
#4476=ORIENTED_EDGE ( 'NONE', *, *, #13230, .F. ) ;
#4477=CARTESIAN_POINT ( 'NONE',  ( 2.449293598294700991E-16, -97.00000000000000000, -13.00000000000000178 ) ) ;
#4478=DIRECTION ( 'NONE',  ( 0.000000000000000000, 0.000000000000000000, 1.000000000000000000 ) ) ;
#4480=ORIENTED_EDGE ( 'NONE', *, *, #12768, .T. ) ;
#4481=DIRECTION ( 'NONE',  ( 0.000000000000000000, 0.000000000000000000, 1.000000000000000000 ) ) ;
#4482=CIRCLE ( 'NONE', #12235, 63.00000000000000000 ) ;
#4484=ORIENTED_EDGE ( 'NONE', *, *, #81, .F. ) ;
#4485=VERTEX_POINT ( 'NONE', #3953 ) ;
#4486=DIRECTION ( 'NONE',  ( -1.000000000000000000, -1.387778780781434947E-14, 0.000000000000000000 ) ) ;
#4487=CARTESIAN_POINT ( 'NONE',  ( 9.706953719245472456, 57.06275842387054098, 8.000000000000000000 ) ) ;
#4489=CARTESIAN_POINT ( 'NONE',  ( -33.48561063518626923, 47.21331623427104063, -10.50000000000000000 ) ) ;
#4490=AXIS2_PLACEMENT_3D ( 'NONE', #11425, #96, #4661 ) ;
#4491=CARTESIAN_POINT ( 'NONE',  ( -3.492805317593278058, 46.55633131742322917, -10.50000000000000000 ) ) ;
#4493=AXIS2_PLACEMENT_3D ( 'NONE', #6625, #14538, #14848 ) ;
#4494=AXIS2_PLACEMENT_3D ( 'NONE', #4063, #14158, #6239 ) ;
#4498=CARTESIAN_POINT ( 'NONE',  ( -4.121772567811602173, -51.45950017607692217, -8.000000000000000000 ) ) ;
#4499=CARTESIAN_POINT ( 'NONE',  ( -12.86891638962156215, 56.43380494353993271, -10.50000000000000000 ) ) ;
#4500=EDGE_CURVE ( 'NONE', #1589, #490, #136, .T. ) ;
#4501=ORIENTED_EDGE ( 'NONE', *, *, #8062, .T. ) ;
#4504=CARTESIAN_POINT ( 'NONE',  ( -51.19406879332065330, -13.71740939043347041, -8.000000000000000000 ) ) ;
#4505=AXIS2_PLACEMENT_3D ( 'NONE', #6474, #723, #14624 ) ;
#4507=AXIS2_PLACEMENT_3D ( 'NONE', #10016, #7808, #2048 ) ;
#4508=DIRECTION ( 'NONE',  ( 1.000000000000000000, 8.881784197001252323E-16, 0.000000000000000000 ) ) ;
#4509=DIRECTION ( 'NONE',  ( 0.000000000000000000, 0.000000000000000000, -1.000000000000000000 ) ) ;
#4513=AXIS2_PLACEMENT_3D ( 'NONE', #5534, #5753, #839 ) ;
#4514=VERTEX_POINT ( 'NONE', #7492 ) ;
#4516=DIRECTION ( 'NONE',  ( -1.000000000000000000, 0.000000000000000000, 0.000000000000000000 ) ) ;
#4517=CARTESIAN_POINT ( 'NONE',  ( 32.26435573746228158, -42.04772703543541468, 10.49999999999999822 ) ) ;
#4519=PLANE ( 'NONE',  #14418 ) ;
#4521=AXIS2_PLACEMENT_3D ( 'NONE', #1333, #6172, #5948 ) ;
#4523=VERTEX_POINT ( 'NONE', #14879 ) ;
#4525=DIRECTION ( 'NONE',  ( 1.000000000000000000, 0.000000000000000000, 0.000000000000000000 ) ) ;
#4526=CYLINDRICAL_SURFACE ( 'NONE', #7503, 0.5000000000000004441 ) ;
#4527=CARTESIAN_POINT ( 'NONE',  ( -49.00442420935969778, 30.80502811811250297, 8.000000000000000000 ) ) ;
#4529=ORIENTED_EDGE ( 'NONE', *, *, #14012, .F. ) ;
#4530=VERTEX_POINT ( 'NONE', #5680 ) ;
#4531=CIRCLE ( 'NONE', #11070, 53.55662432702593634 ) ;
#4532=CARTESIAN_POINT ( 'NONE',  ( -51.19406879332065330, -13.71740939043347041, 10.49999999999999822 ) ) ;
#4534=CARTESIAN_POINT ( 'NONE',  ( 6.917888187663118416, 52.54657765281190507, -8.000000000000000000 ) ) ;
#4535=ORIENTED_EDGE ( 'NONE', *, *, #9807, .F. ) ;
#4536=ADVANCED_FACE ( 'NONE', ( #3185 ), #12591, .F. ) ;
#4537=EDGE_CURVE ( 'NONE', #14514, #7460, #10555, .T. ) ;
#4538=ORIENTED_EDGE ( 'NONE', *, *, #2118, .T. ) ;
#4540=AXIS2_PLACEMENT_3D ( 'NONE', #9710, #9945, #13231 ) ;
#4541=CARTESIAN_POINT ( 'NONE',  ( 0.000000000000000000, 0.000000000000000000, -28.00000000000000000 ) ) ;
#4543=FACE_OUTER_BOUND ( 'NONE', #1515, .T. ) ;
#4544=FACE_OUTER_BOUND ( 'NONE', #9773, .T. ) ;
#4545=EDGE_CURVE ( 'NONE', #9298, #8164, #386, .T. ) ;
#4547=CARTESIAN_POINT ( 'NONE',  ( 37.12029293941315444, -89.61631465359504034, 10.49999999999999822 ) ) ;
#4548=ORIENTED_EDGE ( 'NONE', *, *, #539, .F. ) ;
#4549=CARTESIAN_POINT ( 'NONE',  ( 33.47282819776613394, -39.30189486418255740, -13.00000000000000178 ) ) ;
#4554=ORIENTED_EDGE ( 'NONE', *, *, #13792, .T. ) ;
#4555=PLANE ( 'NONE',  #12038 ) ;
#4556=EDGE_LOOP ( 'NONE', ( #11891, #3233, #2776, #9316, #1766, #3206 ) ) ;
#4557=DIRECTION ( 'NONE',  ( 0.000000000000000000, 0.000000000000000000, -1.000000000000000000 ) ) ;
#4558=DIRECTION ( 'NONE',  ( 1.000000000000000000, -1.172395514004165559E-13, 0.000000000000000000 ) ) ;
#4560=CARTESIAN_POINT ( 'NONE',  ( 0.000000000000000000, 0.000000000000000000, 8.000000000000000000 ) ) ;
#4561=VERTEX_POINT ( 'NONE', #5605 ) ;
#4562=VECTOR ( 'NONE', #981, 1000.000000000000000 ) ;
#4563=DIRECTION ( 'NONE',  ( 1.000000000000000000, 0.000000000000000000, 0.000000000000000000 ) ) ;
#4564=ORIENTED_EDGE ( 'NONE', *, *, #6462, .T. ) ;
#4566=LINE ( 'NONE', #10400, #3611 ) ;
#4567=ORIENTED_EDGE ( 'NONE', *, *, #14406, .T. ) ;
#4568=DIRECTION ( 'NONE',  ( 1.000000000000000000, 0.000000000000000000, 0.000000000000000000 ) ) ;
#4574=EDGE_CURVE ( 'NONE', #9479, #8402, #13725, .T. ) ;
#4579=CARTESIAN_POINT ( 'NONE',  ( 9.714003807514275834, 53.63365512954683112, -8.000000000000000000 ) ) ;
#4580=DIRECTION ( 'NONE',  ( -0.000000000000000000, -0.000000000000000000, 1.000000000000000000 ) ) ;
#4581=DIRECTION ( 'NONE',  ( 1.000000000000000000, 0.000000000000000000, -0.000000000000000000 ) ) ;
#4582=EDGE_LOOP ( 'NONE', ( #2651, #8633, #10326, #3578 ) ) ;
#4583=DIRECTION ( 'NONE',  ( 1.000000000000000000, 0.000000000000000000, -0.000000000000000000 ) ) ;
#4584=ORIENTED_EDGE ( 'NONE', *, *, #83, .F. ) ;
#4585=DIRECTION ( 'NONE',  ( 1.000000000000000000, 0.000000000000000000, 0.000000000000000000 ) ) ;
#4587=EDGE_CURVE ( 'NONE', #5511, #3376, #13896, .T. ) ;
#4590=CARTESIAN_POINT ( 'NONE',  ( -3.492805317593278058, 46.55633131742322917, -10.50000000000000000 ) ) ;
#4591=ADVANCED_FACE ( 'NONE', ( #10088 ), #6728, .T. ) ;
#4594=CARTESIAN_POINT ( 'NONE',  ( -47.21331623427138879, -33.48561063518577896, 8.000000000000000000 ) ) ;
#4596=ORIENTED_EDGE ( 'NONE', *, *, #5389, .F. ) ;
#4597=ORIENTED_EDGE ( 'NONE', *, *, #12291, .T. ) ;
#4598=ORIENTED_EDGE ( 'NONE', *, *, #7534, .F. ) ;
#4600=EDGE_CURVE ( 'NONE', #12645, #14446, #9583, .T. ) ;
#4602=DIRECTION ( 'NONE',  ( -1.000000000000000000, 0.000000000000000000, 0.000000000000000000 ) ) ;
#4604=VERTEX_POINT ( 'NONE', #11316 ) ;
#4605=AXIS2_PLACEMENT_3D ( 'NONE', #1592, #3801, #2726 ) ;
#4606=EDGE_LOOP ( 'NONE', ( #8119, #935, #437, #393 ) ) ;
#4607=ORIENTED_EDGE ( 'NONE', *, *, #12597, .T. ) ;
#4609=AXIS2_PLACEMENT_3D ( 'NONE', #13349, #8868, #12298 ) ;
#4611=DIRECTION ( 'NONE',  ( 0.000000000000000000, 0.000000000000000000, -1.000000000000000000 ) ) ;
#4613=AXIS2_PLACEMENT_3D ( 'NONE', #4451, #13478, #9061 ) ;
#4614=DIRECTION ( 'NONE',  ( 0.000000000000000000, 0.000000000000000000, 1.000000000000000000 ) ) ;
#4616=ORIENTED_EDGE ( 'NONE', *, *, #9543, .F. ) ;
#4619=EDGE_LOOP ( 'NONE', ( #7632, #2653, #2338, #15004 ) ) ;
#4620=CIRCLE ( 'NONE', #12372, 53.55662432702593634 ) ;
#4621=CARTESIAN_POINT ( 'NONE',  ( 11.55014193876178652, -53.26842454702432406, 8.000000000000000000 ) ) ;
#4622=DIRECTION ( 'NONE',  ( 0.000000000000000000, 0.000000000000000000, 1.000000000000000000 ) ) ;
#4623=ORIENTED_EDGE ( 'NONE', *, *, #5000, .F. ) ;
#4624=ORIENTED_EDGE ( 'NONE', *, *, #733, .F. ) ;
#4625=DIRECTION ( 'NONE',  ( 0.000000000000000000, 0.000000000000000000, 1.000000000000000000 ) ) ;
#4626=CIRCLE ( 'NONE', #14578, 100.0000000000000000 ) ;
#4627=ORIENTED_EDGE ( 'NONE', *, *, #363, .T. ) ;
#4628=CARTESIAN_POINT ( 'NONE',  ( 47.63108361037843252, 56.43380494353993271, -10.50000000000000000 ) ) ;
#4630=FACE_OUTER_BOUND ( 'NONE', #7313, .T. ) ;
#4633=ADVANCED_FACE ( 'NONE', ( #10155 ), #4555, .F. ) ;
#4634=ORIENTED_EDGE ( 'NONE', *, *, #11236, .F. ) ;
#4635=CIRCLE ( 'NONE', #1725, 0.5000000000000038858 ) ;
#4636=LINE ( 'NONE', #9253, #10656 ) ;
#4637=ADVANCED_FACE ( 'NONE', ( #4406 ), #1966, .T. ) ;
#4638=ORIENTED_EDGE ( 'NONE', *, *, #8145, .F. ) ;
#4639=AXIS2_PLACEMENT_3D ( 'NONE', #1490, #6247, #13260 ) ;
#4640=CIRCLE ( 'NONE', #9464, 60.50000000000000000 ) ;
#4641=FACE_OUTER_BOUND ( 'NONE', #11103, .T. ) ;
#4643=DIRECTION ( 'NONE',  ( 1.000000000000000000, 0.000000000000000000, 0.000000000000000000 ) ) ;
#4644=EDGE_CURVE ( 'NONE', #212, #11670, #9348, .T. ) ;
#4646=DIRECTION ( 'NONE',  ( 1.000000000000000000, 0.000000000000000000, 0.000000000000000000 ) ) ;
#4650=CARTESIAN_POINT ( 'NONE',  ( -1.674280531759317014, 94.51066581171355097, 8.000000000000000000 ) ) ;
#4651=LINE ( 'NONE', #9124, #1914 ) ;
#4652=EDGE_CURVE ( 'NONE', #9694, #11315, #2084, .T. ) ;
#4653=CARTESIAN_POINT ( 'NONE',  ( 0.000000000000000000, 0.000000000000000000, -10.50000000000000000 ) ) ;
#4654=AXIS2_PLACEMENT_3D ( 'NONE', #9728, #9882, #5192 ) ;
#4655=EDGE_LOOP ( 'NONE', ( #9559, #1562, #1389, #8757 ) ) ;
#4657=DIRECTION ( 'NONE',  ( 0.000000000000000000, 0.000000000000000000, -1.000000000000000000 ) ) ;
#4658=CIRCLE ( 'NONE', #5143, 0.5000000000000038858 ) ;
#4659=CYLINDRICAL_SURFACE ( 'NONE', #14134, 3.000000000000002665 ) ;
#4660=ORIENTED_EDGE ( 'NONE', *, *, #11960, .T. ) ;
#4661=DIRECTION ( 'NONE',  ( -1.000000000000000000, 0.000000000000000000, 0.000000000000000000 ) ) ;
#4663=CARTESIAN_POINT ( 'NONE',  ( -57.06275842387042729, 9.706953719246069312, -10.50000000000000000 ) ) ;
#4664=ORIENTED_EDGE ( 'NONE', *, *, #11417, .T. ) ;
#4665=CIRCLE ( 'NONE', #1509, 50.00000000000000000 ) ;
#4668=DIRECTION ( 'NONE',  ( 1.000000000000000000, 8.746504920891462850E-16, 0.000000000000000000 ) ) ;
#4669=VECTOR ( 'NONE', #6087, 1000.000000000000000 ) ;
#4670=DIRECTION ( 'NONE',  ( 0.000000000000000000, 0.000000000000000000, -1.000000000000000000 ) ) ;
#4671=ORIENTED_EDGE ( 'NONE', *, *, #10479, .F. ) ;
#4672=CYLINDRICAL_SURFACE ( 'NONE', #14710, 63.00000000000000000 ) ;
#4673=DIRECTION ( 'NONE',  ( 0.000000000000000000, 0.000000000000000000, 1.000000000000000000 ) ) ;
#4677=VERTEX_POINT ( 'NONE', #5005 ) ;
#4678=EDGE_CURVE ( 'NONE', #11559, #11449, #8331, .T. ) ;
#4679=AXIS2_PLACEMENT_3D ( 'NONE', #6686, #11340, #1844 ) ;
#4680=ORIENTED_EDGE ( 'NONE', *, *, #10839, .T. ) ;
#4681=ORIENTED_EDGE ( 'NONE', *, *, #12795, .F. ) ;
#4682=DIRECTION ( 'NONE',  ( 0.000000000000000000, 0.000000000000000000, -1.000000000000000000 ) ) ;
#4683=ADVANCED_FACE ( 'NONE', ( #3631 ), #9609, .F. ) ;
#4684=CIRCLE ( 'NONE', #7081, 60.50000000000000000 ) ;
#4685=LINE ( 'NONE', #10664, #13865 ) ;
#4688=CARTESIAN_POINT ( 'NONE',  ( -96.58511096861892042, -0.2790467552922097916, -10.50000000000000000 ) ) ;
#4691=VECTOR ( 'NONE', #6843, 1000.000000000000000 ) ;
#4692=ORIENTED_EDGE ( 'NONE', *, *, #3365, .F. ) ;
#4694=EDGE_LOOP ( 'NONE', ( #14505, #5457, #12060, #12065, #11607 ) ) ;
#4695=CARTESIAN_POINT ( 'NONE',  ( -47.21331623427138879, -33.48561063518577896, 8.000000000000000000 ) ) ;
#4697=AXIS2_PLACEMENT_3D ( 'NONE', #5227, #12213, #4091 ) ;
#4698=EDGE_CURVE ( 'NONE', #11561, #1107, #12517, .T. ) ;
#4699=ORIENTED_EDGE ( 'NONE', *, *, #12764, .F. ) ;
#4700=VECTOR ( 'NONE', #8546, 1000.000000000000000 ) ;
#4702=DIRECTION ( 'NONE',  ( 0.000000000000000000, 0.000000000000000000, -1.000000000000000000 ) ) ;
#4703=ORIENTED_EDGE ( 'NONE', *, *, #7162, .F. ) ;
#4704=VERTEX_POINT ( 'NONE', #11914 ) ;
#4706=DIRECTION ( 'NONE',  ( 0.000000000000000000, 0.000000000000000000, -1.000000000000000000 ) ) ;
#4707=VECTOR ( 'NONE', #5790, 1000.000000000000000 ) ;
#4708=CARTESIAN_POINT ( 'NONE',  ( 57.06275842387049835, -9.706953719245678514, -10.50000000000000000 ) ) ;
#4709=DIRECTION ( 'NONE',  ( 0.000000000000000000, 0.000000000000000000, 1.000000000000000000 ) ) ;
#4710=CARTESIAN_POINT ( 'NONE',  ( 70.20695371924547601, 57.06275842387054098, -10.50000000000000000 ) ) ;
#4712=ORIENTED_EDGE ( 'NONE', *, *, #4726, .T. ) ;
#4713=AXIS2_PLACEMENT_3D ( 'NONE', #5102, #14068, #10866 ) ;
#4714=CIRCLE ( 'NONE', #14409, 50.00000000000000000 ) ;
#4715=DIRECTION ( 'NONE',  ( 1.000000000000000000, 0.000000000000000000, 0.000000000000000000 ) ) ;
#4717=VERTEX_POINT ( 'NONE', #9387 ) ;
#4719=EDGE_CURVE ( 'NONE', #12763, #6431, #11692, .T. ) ;
#4720=ORIENTED_EDGE ( 'NONE', *, *, #4975, .F. ) ;
#4721=ADVANCED_FACE ( 'NONE', ( #5821 ), #3562, .F. ) ;
#4723=EDGE_CURVE ( 'NONE', #12781, #14062, #6642, .T. ) ;
#4724=ORIENTED_EDGE ( 'NONE', *, *, #14136, .T. ) ;
#4725=DIRECTION ( 'NONE',  ( 0.000000000000000000, 0.000000000000000000, 1.000000000000000000 ) ) ;
#4726=EDGE_CURVE ( 'NONE', #12336, #10098, #10781, .T. ) ;
#4728=DIRECTION ( 'NONE',  ( 0.000000000000000000, 0.000000000000000000, 1.000000000000000000 ) ) ;
#4729=DIRECTION ( 'NONE',  ( 1.000000000000000000, 0.000000000000000000, 0.000000000000000000 ) ) ;
#4731=AXIS2_PLACEMENT_3D ( 'NONE', #10765, #6200, #10838 ) ;
#4734=EDGE_CURVE ( 'NONE', #9852, #4717, #10297, .T. ) ;
#4735=CYLINDRICAL_SURFACE ( 'NONE', #13876, 2.649999999999992806 ) ;
#4740=DIRECTION ( 'NONE',  ( 1.000000000000000000, 0.000000000000000000, 0.000000000000000000 ) ) ;
#4741=CIRCLE ( 'NONE', #13955, 3.000000000000002665 ) ;
#4742=CARTESIAN_POINT ( 'NONE',  ( -32.26435573746199736, 42.04772703543562073, -8.000000000000000000 ) ) ;
#4743=EDGE_CURVE ( 'NONE', #12589, #1338, #2794, .T. ) ;
#4745=CARTESIAN_POINT ( 'NONE',  ( -65.58935777509570642, -68.58935777509452691, -8.000000000000000000 ) ) ;
#4748=FACE_OUTER_BOUND ( 'NONE', #15010, .T. ) ;
#4749=CIRCLE ( 'NONE', #5219, 53.55662432702593634 ) ;
#4751=DIRECTION ( 'NONE',  ( -1.000000000000000000, 0.000000000000000000, 0.000000000000000000 ) ) ;
#4752=CIRCLE ( 'NONE', #13236, 100.0000000000000000 ) ;
#4753=VERTEX_POINT ( 'NONE', #13970 ) ;
#4754=CARTESIAN_POINT ( 'NONE',  ( 9.706953719245472456, 57.06275842387054098, -10.50000000000000000 ) ) ;
#4757=AXIS2_PLACEMENT_3D ( 'NONE', #10449, #10305, #8092 ) ;
#4758=ORIENTED_EDGE ( 'NONE', *, *, #13726, .F. ) ;
#4759=VERTEX_POINT ( 'NONE', #10536 ) ;
#4764=EDGE_CURVE ( 'NONE', #6659, #8680, #1578, .T. ) ;
#4765=DIRECTION ( 'NONE',  ( 1.000000000000000000, 0.000000000000000000, 0.000000000000000000 ) ) ;
#4766=CIRCLE ( 'NONE', #12282, 60.50000000000000000 ) ;
#4768=ORIENTED_EDGE ( 'NONE', *, *, #6043, .F. ) ;
#4769=ORIENTED_EDGE ( 'NONE', *, *, #2760, .T. ) ;
#4771=CARTESIAN_POINT ( 'NONE',  ( 52.05085522212507243, -6.852625091552522640, -10.50000000000000000 ) ) ;
#4774=ORIENTED_EDGE ( 'NONE', *, *, #9164, .F. ) ;
#4776=ORIENTED_EDGE ( 'NONE', *, *, #8437, .T. ) ;
#4778=CARTESIAN_POINT ( 'NONE',  ( -89.33979373934396051, 36.70371619500605220, 10.49999999999999822 ) ) ;
#4779=CYLINDRICAL_SURFACE ( 'NONE', #10074, 56.99999999999999289 ) ;
#4780=DIRECTION ( 'NONE',  ( -1.000000000000000000, 0.000000000000000000, 0.000000000000000000 ) ) ;
#4781=EDGE_CURVE ( 'NONE', #10988, #6415, #2535, .T. ) ;
#4782=ADVANCED_FACE ( 'NONE', ( #1427 ), #6036, .T. ) ;
#4785=ORIENTED_EDGE ( 'NONE', *, *, #11918, .F. ) ;
#4786=DIRECTION ( 'NONE',  ( 0.000000000000000000, 0.000000000000000000, -1.000000000000000000 ) ) ;
#4787=VERTEX_POINT ( 'NONE', #13047 ) ;
#4788=EDGE_LOOP ( 'NONE', ( #6966, #12761, #4680, #13082, #4436 ) ) ;
#4789=FACE_OUTER_BOUND ( 'NONE', #4461, .T. ) ;
#4790=ORIENTED_EDGE ( 'NONE', *, *, #2319, .T. ) ;
#4791=CARTESIAN_POINT ( 'NONE',  ( -56.43380494354004639, -12.86891638962099549, -13.00000000000000178 ) ) ;
#4792=AXIS2_PLACEMENT_3D ( 'NONE', #10152, #2038, #1755 ) ;
#4793=DIRECTION ( 'NONE',  ( 1.000000000000000000, 0.000000000000000000, 0.000000000000000000 ) ) ;
#4794=DIRECTION ( 'NONE',  ( 0.000000000000000000, 0.000000000000000000, 1.000000000000000000 ) ) ;
#4803=CARTESIAN_POINT ( 'NONE',  ( -68.58935777509570642, -68.58935777509452691, 8.000000000000000000 ) ) ;
#4806=DIRECTION ( 'NONE',  ( 1.000000000000000000, 0.000000000000000000, 0.000000000000000000 ) ) ;
#4810=DIRECTION ( 'NONE',  ( 0.000000000000000000, 0.000000000000000000, -1.000000000000000000 ) ) ;
#4812=CARTESIAN_POINT ( 'NONE',  ( 57.06275842387049835, -9.706953719245678514, -10.50000000000000000 ) ) ;
#4813=CARTESIAN_POINT ( 'NONE',  ( 13.60620885621573883, -51.79945067148128146, -10.50000000000000000 ) ) ;
#4815=DIRECTION ( 'NONE',  ( 1.000000000000000000, -8.881784197001252323E-16, 0.000000000000000000 ) ) ;
#4816=ADVANCED_FACE ( 'NONE', ( #9839 ), #3936, .T. ) ;
#4817=ORIENTED_EDGE ( 'NONE', *, *, #11886, .T. ) ;
#4818=EDGE_CURVE ( 'NONE', #11004, #5663, #14183, .T. ) ;
#4822=VERTEX_POINT ( 'NONE', #8627 ) ;
#4823=ORIENTED_EDGE ( 'NONE', *, *, #5340, .F. ) ;
#4824=EDGE_CURVE ( 'NONE', #7919, #7026, #4254, .T. ) ;
#4827=FACE_OUTER_BOUND ( 'NONE', #8789, .T. ) ;
#4828=DIRECTION ( 'NONE',  ( 1.000000000000000000, 0.000000000000000000, 0.000000000000000000 ) ) ;
#4829=DIRECTION ( 'NONE',  ( 0.000000000000000000, 0.000000000000000000, 1.000000000000000000 ) ) ;
#4831=ORIENTED_EDGE ( 'NONE', *, *, #5960, .T. ) ;
#4835=AXIS2_PLACEMENT_3D ( 'NONE', #12477, #7686, #2140 ) ;
#4836=CARTESIAN_POINT ( 'NONE',  ( 86.67575032682076142, 37.71449950291080455, -13.00000000000000178 ) ) ;
#4838=ORIENTED_EDGE ( 'NONE', *, *, #1757, .F. ) ;
#4840=CARTESIAN_POINT ( 'NONE',  ( 0.000000000000000000, 0.000000000000000000, -8.000000000000000000 ) ) ;
#4841=EDGE_LOOP ( 'NONE', ( #2980, #5575, #7395, #9349, #10256 ) ) ;
#4843=LINE ( 'NONE', #9465, #13118 ) ;
#4845=DIRECTION ( 'NONE',  ( 0.000000000000000000, 0.000000000000000000, 1.000000000000000000 ) ) ;
#4849=ORIENTED_EDGE ( 'NONE', *, *, #2673, .T. ) ;
#4851=PLANE ( 'NONE',  #3874 ) ;
#4852=ORIENTED_EDGE ( 'NONE', *, *, #10378, .F. ) ;
#4854=CARTESIAN_POINT ( 'NONE',  ( -13.71740939043329277, 51.19406879332069593, -13.00000000000000178 ) ) ;
#4855=AXIS2_PLACEMENT_3D ( 'NONE', #9698, #2737, #6139 ) ;
#4857=AXIS2_PLACEMENT_3D ( 'NONE', #6688, #14830, #7752 ) ;
#4858=ORIENTED_EDGE ( 'NONE', *, *, #1246, .T. ) ;
#4859=ADVANCED_FACE ( 'NONE', ( #7333 ), #13272, .F. ) ;
#4861=ADVANCED_FACE ( 'NONE', ( #2864 ), #11993, .T. ) ;
#4865=EDGE_CURVE ( 'NONE', #10615, #3633, #9793, .T. ) ;
#4866=EDGE_CURVE ( 'NONE', #2406, #7029, #8837, .T. ) ;
#4867=DIRECTION ( 'NONE',  ( 0.000000000000000000, 0.000000000000000000, -1.000000000000000000 ) ) ;
#4868=ORIENTED_EDGE ( 'NONE', *, *, #642, .F. ) ;
#4873=DIRECTION ( 'NONE',  ( 1.000000000000000000, 0.000000000000000000, 0.000000000000000000 ) ) ;
#4874=AXIS2_PLACEMENT_3D ( 'NONE', #2429, #12775, #11577 ) ;
#4877=AXIS2_PLACEMENT_3D ( 'NONE', #9946, #7592, #11020 ) ;
#4878=CIRCLE ( 'NONE', #10935, 3.000000000000002665 ) ;
#4880=CARTESIAN_POINT ( 'NONE',  ( 0.000000000000000000, 0.000000000000000000, -8.000000000000000000 ) ) ;
#4881=ORIENTED_EDGE ( 'NONE', *, *, #11886, .F. ) ;
#4882=EDGE_CURVE ( 'NONE', #12788, #3583, #12731, .T. ) ;
#4883=AXIS2_PLACEMENT_3D ( 'NONE', #6130, #3949, #2807 ) ;
#4884=DIRECTION ( 'NONE',  ( -1.000000000000000000, 0.000000000000000000, 0.000000000000000000 ) ) ;
#4887=EDGE_CURVE ( 'NONE', #10576, #10355, #3998, .T. ) ;
#4888=CIRCLE ( 'NONE', #272, 3.000000000000002665 ) ;
#4889=DIRECTION ( 'NONE',  ( 1.000000000000000000, 0.000000000000000000, 0.000000000000000000 ) ) ;
#4890=EDGE_LOOP ( 'NONE', ( #7470, #6289, #13534, #10313, #4785, #1464, #2127, #14316, #13847, #5099, #10398, #4634, #1047, #12613, #1352, #12467, #12222, #14228, #10235, #10739 ) ) ;
#4891=CARTESIAN_POINT ( 'NONE',  ( -57.06275842387042729, 9.706953719246069312, -13.00000000000000178 ) ) ;
#4892=ORIENTED_EDGE ( 'NONE', *, *, #6543, .T. ) ;
#4894=DIRECTION ( 'NONE',  ( -0.000000000000000000, -0.000000000000000000, 1.000000000000000000 ) ) ;
#4898=EDGE_LOOP ( 'NONE', ( #12021, #6740, #5218, #10990 ) ) ;
#4900=DIRECTION ( 'NONE',  ( 0.000000000000000000, 0.000000000000000000, 1.000000000000000000 ) ) ;
#4901=DIRECTION ( 'NONE',  ( -1.000000000000000000, -1.065814103640150279E-14, 0.000000000000000000 ) ) ;
#4903=CIRCLE ( 'NONE', #13620, 3.000000000000002665 ) ;
#4904=ORIENTED_EDGE ( 'NONE', *, *, #404, .T. ) ;
#4905=ADVANCED_FACE ( 'NONE', ( #3146 ), #10121, .T. ) ;
#4906=VERTEX_POINT ( 'NONE', #12491 ) ;
#4907=ADVANCED_FACE ( 'NONE', ( #2796 ), #6696, .F. ) ;
#4909=VERTEX_POINT ( 'NONE', #11347 ) ;
#4913=DIRECTION ( 'NONE',  ( 0.000000000000000000, 0.000000000000000000, 1.000000000000000000 ) ) ;
#4919=VERTEX_POINT ( 'NONE', #5145 ) ;
#4921=CARTESIAN_POINT ( 'NONE',  ( 0.2790467552932288098, 97.41488903138106537, -13.00000000000000178 ) ) ;
#4923=AXIS2_PLACEMENT_3D ( 'NONE', #12099, #14151, #10644 ) ;
#4924=LINE ( 'NONE', #505, #4700 ) ;
#4925=ORIENTED_EDGE ( 'NONE', *, *, #2501, .F. ) ;
#4926=ORIENTED_EDGE ( 'NONE', *, *, #6700, .F. ) ;
#4927=DIRECTION ( 'NONE',  ( -1.000000000000000000, 2.678169576946649542E-15, 0.000000000000000000 ) ) ;
#4928=ORIENTED_EDGE ( 'NONE', *, *, #5776, .T. ) ;
#4929=VECTOR ( 'NONE', #10573, 1000.000000000000000 ) ;
#4930=ADVANCED_FACE ( 'NONE', ( #11724 ), #8147, .T. ) ;
#4934=ORIENTED_EDGE ( 'NONE', *, *, #7601, .F. ) ;
#4935=AXIS2_PLACEMENT_3D ( 'NONE', #13548, #5508, #4228 ) ;
#4936=LINE ( 'NONE', #5230, #8270 ) ;
#4939=DIRECTION ( 'NONE',  ( 0.000000000000000000, 0.000000000000000000, 1.000000000000000000 ) ) ;
#4940=CIRCLE ( 'NONE', #4457, 3.000000000000002665 ) ;
#4941=ORIENTED_EDGE ( 'NONE', *, *, #2793, .T. ) ;
#4943=CARTESIAN_POINT ( 'NONE',  ( -26.49999999999971578, -45.89934640057541060, -13.00000000000000178 ) ) ;
#4945=AXIS2_PLACEMENT_3D ( 'NONE', #14773, #14542, #6628 ) ;
#4946=CARTESIAN_POINT ( 'NONE',  ( 68.01302780753354682, -65.64523757230297463, 8.000000000000000000 ) ) ;
#4947=CARTESIAN_POINT ( 'NONE',  ( 36.14014761921570340, 11.74264578624841171, -25.50000000000000355 ) ) ;
#4948=DIRECTION ( 'NONE',  ( -1.000000000000000000, 0.000000000000000000, 0.000000000000000000 ) ) ;
#4949=DIRECTION ( 'NONE',  ( -0.000000000000000000, -0.000000000000000000, 1.000000000000000000 ) ) ;
#4950=FACE_OUTER_BOUND ( 'NONE', #2809, .T. ) ;
#4951=DIRECTION ( 'NONE',  ( 0.000000000000000000, 0.000000000000000000, 1.000000000000000000 ) ) ;
#4954=ADVANCED_FACE ( 'NONE', ( #1317 ), #3597, .F. ) ;
#4955=AXIS2_PLACEMENT_3D ( 'NONE', #10276, #13777, #5717 ) ;
#4957=EDGE_CURVE ( 'NONE', #7149, #14223, #7383, .T. ) ;
#4960=CARTESIAN_POINT ( 'NONE',  ( 45.89934640057532533, -26.49999999999987566, -8.000000000000000000 ) ) ;
#4961=DIRECTION ( 'NONE',  ( 0.000000000000000000, 0.000000000000000000, 1.000000000000000000 ) ) ;
#4962=CARTESIAN_POINT ( 'NONE',  ( -41.54772703543551415, -32.26435573746212526, -13.00000000000000178 ) ) ;
#4964=ORIENTED_EDGE ( 'NONE', *, *, #5737, .F. ) ;
#4967=AXIS2_PLACEMENT_3D ( 'NONE', #13956, #13642, #3550 ) ;
#4969=EDGE_CURVE ( 'NONE', #8885, #10986, #13697, .T. ) ;
#4971=DIRECTION ( 'NONE',  ( 1.000000000000000000, 0.000000000000000000, 0.000000000000000000 ) ) ;
#4973=DIRECTION ( 'NONE',  ( 0.000000000000000000, 0.000000000000000000, 1.000000000000000000 ) ) ;
#4974=ADVANCED_FACE ( 'NONE', ( #5782 ), #4519, .F. ) ;
#4975=EDGE_CURVE ( 'NONE', #511, #14, #12785, .T. ) ;
#4977=VERTEX_POINT ( 'NONE', #11586 ) ;
#4978=AXIS2_PLACEMENT_3D ( 'NONE', #655, #423, #2849 ) ;
#4979=FACE_BOUND ( 'NONE', #14570, .T. ) ;
#4980=DIRECTION ( 'NONE',  ( 1.000000000000000000, 0.000000000000000000, -0.000000000000000000 ) ) ;
#4981=AXIS2_PLACEMENT_3D ( 'NONE', #10338, #1383, #10627 ) ;
#4983=ORIENTED_EDGE ( 'NONE', *, *, #11746, .F. ) ;
#4985=VECTOR ( 'NONE', #11569, 1000.000000000000000 ) ;
#4986=ORIENTED_EDGE ( 'NONE', *, *, #8299, .T. ) ;
#4988=CIRCLE ( 'NONE', #581, 60.50000000000000000 ) ;
#4989=VECTOR ( 'NONE', #922, 1000.000000000000000 ) ;
#4990=DIRECTION ( 'NONE',  ( 0.000000000000000000, 0.000000000000000000, 1.000000000000000000 ) ) ;
#4991=CARTESIAN_POINT ( 'NONE',  ( -69.08004447556112382, -68.68541276968802833, -10.50000000000000000 ) ) ;
#4993=ORIENTED_EDGE ( 'NONE', *, *, #12309, .F. ) ;
#4994=ORIENTED_EDGE ( 'NONE', *, *, #12616, .F. ) ;
#4997=CARTESIAN_POINT ( 'NONE',  ( -36.62029293941440500, -89.61631465359452875, -13.00000000000000178 ) ) ;
#4998=CYLINDRICAL_SURFACE ( 'NONE', #12012, 0.5000000000000004441 ) ;
#4999=AXIS2_PLACEMENT_3D ( 'NONE', #9554, #12010, #11781 ) ;
#5000=EDGE_CURVE ( 'NONE', #12796, #219, #7861, .T. ) ;
#5003=EDGE_CURVE ( 'NONE', #6857, #9519, #1330, .T. ) ;
#5005=CARTESIAN_POINT ( 'NONE',  ( -89.33979373934396051, 36.70371619500605220, -10.50000000000000000 ) ) ;
#5007=CIRCLE ( 'NONE', #1374, 0.5000000000000022204 ) ;
#5008=CARTESIAN_POINT ( 'NONE',  ( -37.12029293941441210, -89.61631465359452875, 8.000000000000000000 ) ) ;
#5009=EDGE_CURVE ( 'NONE', #6265, #7513, #605, .T. ) ;
#5011=CARTESIAN_POINT ( 'NONE',  ( 23.50071946824040836, 45.96504489226015977, 8.000000000000000000 ) ) ;
#5012=CARTESIAN_POINT ( 'NONE',  ( 30.80502811811196295, 49.00442420936003174, -13.00000000000000178 ) ) ;
#5013=DIRECTION ( 'NONE',  ( 1.000000000000000000, 0.000000000000000000, 0.000000000000000000 ) ) ;
#5014=ORIENTED_EDGE ( 'NONE', *, *, #7200, .F. ) ;
#5015=FACE_OUTER_BOUND ( 'NONE', #8179, .T. ) ;
#5016=EDGE_CURVE ( 'NONE', #7285, #11296, #12245, .T. ) ;
#5017=EDGE_CURVE ( 'NONE', #3376, #14898, #14915, .T. ) ;
#5018=AXIS2_PLACEMENT_3D ( 'NONE', #9130, #1019, #2075 ) ;
#5020=ORIENTED_EDGE ( 'NONE', *, *, #11048, .T. ) ;
#5021=DIRECTION ( 'NONE',  ( -1.000000000000000000, 0.000000000000000000, 0.000000000000000000 ) ) ;
#5023=DIRECTION ( 'NONE',  ( 0.000000000000000000, 0.000000000000000000, 1.000000000000000000 ) ) ;
#5025=LINE ( 'NONE', #1604, #747 ) ;
#5027=PLANE ( 'NONE',  #6021 ) ;
#5029=EDGE_LOOP ( 'NONE', ( #9634, #3151 ) ) ;
#5033=CARTESIAN_POINT ( 'NONE',  ( 9.706953719245472456, 57.06275842387054098, 10.49999999999999822 ) ) ;
#5034=ORIENTED_EDGE ( 'NONE', *, *, #8593, .T. ) ;
#5035=DIRECTION ( 'NONE',  ( 0.000000000000000000, 0.000000000000000000, -1.000000000000000000 ) ) ;
#5036=ORIENTED_EDGE ( 'NONE', *, *, #883, .T. ) ;
#5037=CARTESIAN_POINT ( 'NONE',  ( -39.04772703543551415, -32.26435573746212526, -8.000000000000000000 ) ) ;
#5039=DIRECTION ( 'NONE',  ( 1.000000000000000000, 0.000000000000000000, 0.000000000000000000 ) ) ;
#5040=DIRECTION ( 'NONE',  ( -1.000000000000000000, 0.000000000000000000, 0.000000000000000000 ) ) ;
#5042=ORIENTED_EDGE ( 'NONE', *, *, #1167, .T. ) ;
#5043=FACE_OUTER_BOUND ( 'NONE', #7556, .T. ) ;
#5047=ORIENTED_EDGE ( 'NONE', *, *, #12369, .T. ) ;
#5048=ADVANCED_FACE ( 'NONE', ( #12851 ), #9134, .T. ) ;
#5049=EDGE_CURVE ( 'NONE', #2937, #5169, #7064, .T. ) ;
#5050=CARTESIAN_POINT ( 'NONE',  ( 51.19406879332056093, 13.71740939043382745, -10.50000000000000000 ) ) ;
#5052=CARTESIAN_POINT ( 'NONE',  ( -65.64523757230321621, -68.01302780753330524, 8.000000000000000000 ) ) ;
#5055=CARTESIAN_POINT ( 'NONE',  ( 30.43807145043610518, -39.66766701456170097, -8.000000000000000000 ) ) ;
#5056=AXIS2_PLACEMENT_3D ( 'NONE', #5764, #11399, #13984 ) ;
#5058=ORIENTED_EDGE ( 'NONE', *, *, #4433, .F. ) ;
#5059=FACE_OUTER_BOUND ( 'NONE', #5765, .T. ) ;
#5060=DIRECTION ( 'NONE',  ( -0.000000000000000000, -0.000000000000000000, 1.000000000000000000 ) ) ;
#5063=ORIENTED_EDGE ( 'NONE', *, *, #1707, .T. ) ;
#5064=DIRECTION ( 'NONE',  ( 0.000000000000000000, 0.000000000000000000, 1.000000000000000000 ) ) ;
#5065=ORIENTED_EDGE ( 'NONE', *, *, #8327, .F. ) ;
#5066=FACE_OUTER_BOUND ( 'NONE', #11729, .T. ) ;
#5067=EDGE_CURVE ( 'NONE', #1787, #10362, #12711, .T. ) ;
#5068=LINE ( 'NONE', #6261, #12474 ) ;
#5069=FILL_AREA_STYLE ('',( #440 ) ) ;
#5070=AXIS2_PLACEMENT_3D ( 'NONE', #9960, #6460, #8821 ) ;
#5075=CARTESIAN_POINT ( 'NONE',  ( -92.38795325112825196, 38.26834323651002023, -8.000000000000000000 ) ) ;
#5076=ORIENTED_EDGE ( 'NONE', *, *, #14627, .F. ) ;
#5078=ORIENTED_EDGE ( 'NONE', *, *, #12338, .F. ) ;
#5080=AXIS2_PLACEMENT_3D ( 'NONE', #6128, #10693, #5013 ) ;
#5082=EDGE_CURVE ( 'NONE', #5248, #9892, #12224, .T. ) ;
#5086=CARTESIAN_POINT ( 'NONE',  ( 52.54657765281197612, -6.917888187662545540, -8.000000000000000000 ) ) ;
#5087=VECTOR ( 'NONE', #12170, 1000.000000000000000 ) ;
#5088=AXIS2_PLACEMENT_3D ( 'NONE', #12143, #1516, #9619 ) ;
#5091=AXIS2_PLACEMENT_3D ( 'NONE', #6090, #10956, #14373 ) ;
#5092=CIRCLE ( 'NONE', #4140, 59.50000000000000000 ) ;
#5093=DIRECTION ( 'NONE',  ( 1.000000000000000000, 0.000000000000000000, 0.000000000000000000 ) ) ;
#5094=ORIENTED_EDGE ( 'NONE', *, *, #11313, .F. ) ;
#5096=EDGE_CURVE ( 'NONE', #5511, #4396, #5671, .T. ) ;
#5097=DIRECTION ( 'NONE',  ( 1.000000000000000000, 0.000000000000000000, -0.000000000000000000 ) ) ;
#5099=ORIENTED_EDGE ( 'NONE', *, *, #12668, .F. ) ;
#5100=DIRECTION ( 'NONE',  ( 1.000000000000000000, 0.000000000000000000, 0.000000000000000000 ) ) ;
#5101=AXIS2_PLACEMENT_3D ( 'NONE', #1987, #12320, #4202 ) ;
#5102=CARTESIAN_POINT ( 'NONE',  ( -89.61631465359441506, 37.12029293941468211, -10.50000000000000000 ) ) ;
#5103=ORIENTED_EDGE ( 'NONE', *, *, #43, .T. ) ;
#5104=CARTESIAN_POINT ( 'NONE',  ( 45.89934640057532533, -26.49999999999987566, -10.50000000000000000 ) ) ;
#5105=CIRCLE ( 'NONE', #11915, 53.55662432702593634 ) ;
#5106=ORIENTED_EDGE ( 'NONE', *, *, #10791, .T. ) ;
#5108=AXIS2_PLACEMENT_3D ( 'NONE', #296, #6125, #10768 ) ;
#5109=CARTESIAN_POINT ( 'NONE',  ( -2.449293598294708880E-16, 38.00000000000000000, -28.00000000000000000 ) ) ;
#5110=CARTESIAN_POINT ( 'NONE',  ( -13.58799986788203640, 50.71110588017617005, -10.50000000000000000 ) ) ;
#5112=CARTESIAN_POINT ( 'NONE',  ( 51.45950017607693638, -4.121772567811421872, 8.000000000000000000 ) ) ;
#5114=DIRECTION ( 'NONE',  ( 0.000000000000000000, 0.000000000000000000, -1.000000000000000000 ) ) ;
#5115=CIRCLE ( 'NONE', #13596, 3.000000000000002665 ) ;
#5116=ORIENTED_EDGE ( 'NONE', *, *, #12309, .T. ) ;
#5119=CIRCLE ( 'NONE', #8268, 56.99999999999999289 ) ;
#5121=AXIS2_PLACEMENT_3D ( 'NONE', #12359, #6493, #13425 ) ;
#5122=DIRECTION ( 'NONE',  ( 0.000000000000000000, 0.000000000000000000, 1.000000000000000000 ) ) ;
#5124=ORIENTED_EDGE ( 'NONE', *, *, #14735, .F. ) ;
#5125=CARTESIAN_POINT ( 'NONE',  ( -12.94095225512574920, 48.29629131445349799, 8.000000000000000000 ) ) ;
#5127=DIRECTION ( 'NONE',  ( 0.000000000000000000, 0.000000000000000000, -1.000000000000000000 ) ) ;
#5129=ORIENTED_EDGE ( 'NONE', *, *, #1477, .T. ) ;
#5130=CARTESIAN_POINT ( 'NONE',  ( -41.59008834022669987, -32.46576781417940794, -13.00000000000000178 ) ) ;
#5131=CIRCLE ( 'NONE', #14839, 60.50000000000000000 ) ;
#5132=DIRECTION ( 'NONE',  ( 0.000000000000000000, 0.000000000000000000, -1.000000000000000000 ) ) ;
#5135=VERTEX_POINT ( 'NONE', #6080 ) ;
#5136=EDGE_CURVE ( 'NONE', #11371, #7026, #3672, .T. ) ;
#5137=CARTESIAN_POINT ( 'NONE',  ( 52.54657765281197612, -6.917888187662545540, 8.000000000000000000 ) ) ;
#5138=DIRECTION ( 'NONE',  ( 0.000000000000000000, 0.000000000000000000, 1.000000000000000000 ) ) ;
#5139=EDGE_CURVE ( 'NONE', #11359, #6102, #468, .T. ) ;
#5141=FACE_OUTER_BOUND ( 'NONE', #10746, .T. ) ;
#5143=AXIS2_PLACEMENT_3D ( 'NONE', #10158, #10321, #5684 ) ;
#5144=VERTEX_POINT ( 'NONE', #400 ) ;
#5145=CARTESIAN_POINT ( 'NONE',  ( -92.38795325112907619, -38.26834323650805914, 8.000000000000000000 ) ) ;
#5149=AXIS2_PLACEMENT_3D ( 'NONE', #9294, #10365, #12868 ) ;
#5151=EDGE_CURVE ( 'NONE', #4677, #1124, #3250, .T. ) ;
#5152=EDGE_LOOP ( 'NONE', ( #3000, #966, #13481, #3902 ) ) ;
#5153=ORIENTED_EDGE ( 'NONE', *, *, #13690, .T. ) ;
#5154=CARTESIAN_POINT ( 'NONE',  ( 26.00011991137315803, 45.91029614918951296, -10.50000000000000000 ) ) ;
#5155=DIRECTION ( 'NONE',  ( 1.000000000000000000, 0.000000000000000000, -0.000000000000000000 ) ) ;
#5156=ORIENTED_EDGE ( 'NONE', *, *, #7393, .F. ) ;
#5158=CYLINDRICAL_SURFACE ( 'NONE', #5088, 60.50000000000000000 ) ;
#5159=VERTEX_POINT ( 'NONE', #9418 ) ;
#5160=AXIS2_PLACEMENT_3D ( 'NONE', #7983, #13776, #9050 ) ;
#5162=FACE_OUTER_BOUND ( 'NONE', #9531, .T. ) ;
#5163=CIRCLE ( 'NONE', #13655, 3.000000000000002665 ) ;
#5166=CARTESIAN_POINT ( 'NONE',  ( -32.26435573746199736, 42.04772703543562073, -13.00000000000000178 ) ) ;
#5169=VERTEX_POINT ( 'NONE', #7146 ) ;
#5170=CARTESIAN_POINT ( 'NONE',  ( 0.000000000000000000, 0.000000000000000000, 8.000000000000000000 ) ) ;
#5171=DIRECTION ( 'NONE',  ( 1.000000000000000000, 0.000000000000000000, 0.000000000000000000 ) ) ;
#5172=CARTESIAN_POINT ( 'NONE',  ( -51.19406879332065330, -13.71740939043347041, -10.50000000000000000 ) ) ;
#5175=EDGE_CURVE ( 'NONE', #4338, #7227, #840, .T. ) ;
#5176=ORIENTED_EDGE ( 'NONE', *, *, #2023, .T. ) ;
#5178=ORIENTED_EDGE ( 'NONE', *, *, #595, .T. ) ;
#5179=CARTESIAN_POINT ( 'NONE',  ( -37.12029293941441210, -89.61631465359452875, -10.50000000000000000 ) ) ;
#5181=ORIENTED_EDGE ( 'NONE', *, *, #14663, .T. ) ;
#5182=DIRECTION ( 'NONE',  ( 0.000000000000000000, 0.000000000000000000, 1.000000000000000000 ) ) ;
#5185=DIRECTION ( 'NONE',  ( 0.000000000000000000, 0.000000000000000000, 1.000000000000000000 ) ) ;
#5187=AXIS2_PLACEMENT_3D ( 'NONE', #174, #3897, #1619 ) ;
#5189=CIRCLE ( 'NONE', #11514, 100.0000000000000000 ) ;
#5190=DIRECTION ( 'NONE',  ( -0.000000000000000000, -0.000000000000000000, -1.000000000000000000 ) ) ;
#5192=DIRECTION ( 'NONE',  ( -1.000000000000000000, 0.000000000000000000, 0.000000000000000000 ) ) ;
#5194=ORIENTED_EDGE ( 'NONE', *, *, #2824, .T. ) ;
#5195=DIRECTION ( 'NONE',  ( 0.000000000000000000, 0.000000000000000000, 1.000000000000000000 ) ) ;
#5199=DIRECTION ( 'NONE',  ( -1.000000000000000000, -5.306212985340821979E-15, 0.000000000000000000 ) ) ;
#5200=VECTOR ( 'NONE', #3558, 1000.000000000000000 ) ;
#5202=ORIENTED_EDGE ( 'NONE', *, *, #6567, .F. ) ;
#5204=DIRECTION ( 'NONE',  ( -1.000000000000000000, 0.000000000000000000, 0.000000000000000000 ) ) ;
#5206=AXIS2_PLACEMENT_3D ( 'NONE', #13120, #14765, #6196 ) ;
#5211=CIRCLE ( 'NONE', #7132, 3.000000000000002665 ) ;
#5212=AXIS2_PLACEMENT_3D ( 'NONE', #7529, #12044, #4980 ) ;
#5213=CIRCLE ( 'NONE', #8361, 50.00000000000000000 ) ;
#5214=ORIENTED_EDGE ( 'NONE', *, *, #8567, .T. ) ;
#5215=DIRECTION ( 'NONE',  ( -1.000000000000000000, 0.000000000000000000, 0.000000000000000000 ) ) ;
#5216=DIRECTION ( 'NONE',  ( -1.000000000000000000, 0.000000000000000000, 0.000000000000000000 ) ) ;
#5217=FACE_OUTER_BOUND ( 'NONE', #2419, .T. ) ;
#5218=ORIENTED_EDGE ( 'NONE', *, *, #5549, .T. ) ;
#5219=AXIS2_PLACEMENT_3D ( 'NONE', #1539, #7143, #11800 ) ;
#5221=CARTESIAN_POINT ( 'NONE',  ( 9.706953719245472456, 57.06275842387054098, -8.000000000000000000 ) ) ;
#5222=AXIS2_PLACEMENT_3D ( 'NONE', #8153, #8300, #10580 ) ;
#5223=AXIS2_PLACEMENT_3D ( 'NONE', #4708, #6893, #5978 ) ;
#5225=EDGE_CURVE ( 'NONE', #7077, #7439, #2043, .T. ) ;
#5227=CARTESIAN_POINT ( 'NONE',  ( 36.14014761921570340, 11.74264578624841171, -28.00000000000000000 ) ) ;
#5230=CARTESIAN_POINT ( 'NONE',  ( -87.95718916809170196, 34.62083247296289557, -13.00000000000000178 ) ) ;
#5231=CARTESIAN_POINT ( 'NONE',  ( 0.000000000000000000, 0.000000000000000000, 8.000000000000000000 ) ) ;
#5232=EDGE_LOOP ( 'NONE', ( #9315, #10423, #6868, #8084, #329 ) ) ;
#5233=DIRECTION ( 'NONE',  ( -0.000000000000000000, -0.000000000000000000, 1.000000000000000000 ) ) ;
#5234=ORIENTED_EDGE ( 'NONE', *, *, #1131, .T. ) ;
#5235=VERTEX_POINT ( 'NONE', #2676 ) ;
#5238=DIRECTION ( 'NONE',  ( -0.000000000000000000, -0.000000000000000000, 1.000000000000000000 ) ) ;
#5240=EDGE_CURVE ( 'NONE', #1468, #8993, #1310, .T. ) ;
#5241=ADVANCED_FACE ( 'NONE', ( #8513 ), #13157, .T. ) ;
#5243=DIRECTION ( 'NONE',  ( 0.000000000000000000, 0.000000000000000000, 1.000000000000000000 ) ) ;
#5246=LINE ( 'NONE', #14739, #487 ) ;
#5247=DIRECTION ( 'NONE',  ( 0.000000000000000000, 0.000000000000000000, 1.000000000000000000 ) ) ;
#5248=VERTEX_POINT ( 'NONE', #8371 ) ;
#5250=DIRECTION ( 'NONE',  ( 0.000000000000000000, 0.000000000000000000, 1.000000000000000000 ) ) ;
#5254=ORIENTED_EDGE ( 'NONE', *, *, #8070, .T. ) ;
#5257=ORIENTED_EDGE ( 'NONE', *, *, #4353, .T. ) ;
#5258=AXIS2_PLACEMENT_3D ( 'NONE', #6758, #11583, #11644 ) ;
#5261=PLANE ( 'NONE',  #2785 ) ;
#5262=DIRECTION ( 'NONE',  ( 1.000000000000000000, 0.000000000000000000, 0.000000000000000000 ) ) ;
#5266=DIRECTION ( 'NONE',  ( 0.000000000000000000, 0.000000000000000000, -1.000000000000000000 ) ) ;
#5268=EDGE_CURVE ( 'NONE', #6561, #5962, #9872, .T. ) ;
#5271=PLANE ( 'NONE',  #4494 ) ;
#5272=CARTESIAN_POINT ( 'NONE',  ( -34.12029293941441210, -89.61631465359452875, 8.000000000000000000 ) ) ;
#5273=EDGE_LOOP ( 'NONE', ( #10271, #11563, #6555, #10631, #8283 ) ) ;
#5275=VERTEX_POINT ( 'NONE', #1838 ) ;
#5277=DIRECTION ( 'NONE',  ( -1.000000000000000000, 0.000000000000000000, 0.000000000000000000 ) ) ;
#5279=DIRECTION ( 'NONE',  ( 0.000000000000000000, 0.000000000000000000, 1.000000000000000000 ) ) ;
#5280=EDGE_CURVE ( 'NONE', #9491, #12422, #11741, .T. ) ;
#5283=ORIENTED_EDGE ( 'NONE', *, *, #5369, .T. ) ;
#5284=ORIENTED_EDGE ( 'NONE', *, *, #10369, .T. ) ;
#5285=DIRECTION ( 'NONE',  ( 0.000000000000000000, 0.000000000000000000, -1.000000000000000000 ) ) ;
#5286=DIRECTION ( 'NONE',  ( 1.000000000000000000, 0.000000000000000000, 0.000000000000000000 ) ) ;
#5288=ORIENTED_EDGE ( 'NONE', *, *, #8157, .F. ) ;
#5290=VECTOR ( 'NONE', #7506, 1000.000000000000000 ) ;
#5291=EDGE_LOOP ( 'NONE', ( #7391, #5930, #13969, #702, #12951, #2909, #8314, #14243, #6271, #5014, #13209, #12465, #4934, #10001, #8883, #13028, #1373, #4344, #5465, #4309 ) ) ;
#5292=EDGE_LOOP ( 'NONE', ( #10833, #12967, #4790, #1507, #7139 ) ) ;
#5294=ADVANCED_FACE ( 'NONE', ( #5323, #4346, #6370, #12390, #4200, #12246, #11177 ), #8732, .T. ) ;
#5295=DIRECTION ( 'NONE',  ( 0.000000000000000000, 0.000000000000000000, 1.000000000000000000 ) ) ;
#5298=DIRECTION ( 'NONE',  ( -1.000000000000000000, 0.000000000000000000, -0.000000000000000000 ) ) ;
#5299=CARTESIAN_POINT ( 'NONE',  ( -57.06275842387042729, 9.706953719246069312, -10.50000000000000000 ) ) ;
#5300=ORIENTED_EDGE ( 'NONE', *, *, #7634, .T. ) ;
#5301=CARTESIAN_POINT ( 'NONE',  ( 71.53347797788771345, 69.16568774265620334, -8.000000000000000000 ) ) ;
#5302=ORIENTED_EDGE ( 'NONE', *, *, #12983, .F. ) ;
#5304=ORIENTED_EDGE ( 'NONE', *, *, #10895, .T. ) ;
#5305=DIRECTION ( 'NONE',  ( -1.000000000000000000, 0.000000000000000000, 0.000000000000000000 ) ) ;
#5306=CARTESIAN_POINT ( 'NONE',  ( 0.000000000000000000, 0.000000000000000000, -8.000000000000000000 ) ) ;
#5307=CIRCLE ( 'NONE', #13808, 59.50000000000000000 ) ;
#5308=DIRECTION ( 'NONE',  ( 1.000000000000000000, 0.000000000000000000, 0.000000000000000000 ) ) ;
#5309=CARTESIAN_POINT ( 'NONE',  ( 0.000000000000000000, 0.000000000000000000, -10.50000000000000000 ) ) ;
#5310=DIRECTION ( 'NONE',  ( 0.000000000000000000, 0.000000000000000000, 1.000000000000000000 ) ) ;
#5311=ORIENTED_EDGE ( 'NONE', *, *, #1728, .T. ) ;
#5312=EDGE_CURVE ( 'NONE', #8196, #12042, #9053, .T. ) ;
#5314=CYLINDRICAL_SURFACE ( 'NONE', #9990, 2.649999999999992806 ) ;
#5315=EDGE_CURVE ( 'NONE', #9534, #13716, #3007, .T. ) ;
#5317=CARTESIAN_POINT ( 'NONE',  ( -97.00000000000000000, 1.015776140243522349E-12, -13.00000000000000178 ) ) ;
#5318=VECTOR ( 'NONE', #3640, 1000.000000000000000 ) ;
#5323=FACE_BOUND ( 'NONE', #2664, .T. ) ;
#5325=CARTESIAN_POINT ( 'NONE',  ( -14.07862063237857342, 50.84834283437004387, -10.50000000000000000 ) ) ;
#5327=VERTEX_POINT ( 'NONE', #1903 ) ;
#5328=CIRCLE ( 'NONE', #9443, 55.00000000000000000 ) ;
#5330=AXIS2_PLACEMENT_3D ( 'NONE', #15000, #5725, #1404 ) ;
#5331=CARTESIAN_POINT ( 'NONE',  ( 0.000000000000000000, 0.000000000000000000, 10.50000000000000000 ) ) ;
#5332=CARTESIAN_POINT ( 'NONE',  ( 26.99988008862626643, 45.88839665196127271, -13.00000000000000178 ) ) ;
#5335=AXIS2_PLACEMENT_3D ( 'NONE', #13439, #9860, #7499 ) ;
#5336=DIRECTION ( 'NONE',  ( -0.000000000000000000, -0.000000000000000000, 1.000000000000000000 ) ) ;
#5339=ORIENTED_EDGE ( 'NONE', *, *, #4866, .T. ) ;
#5340=EDGE_CURVE ( 'NONE', #7513, #13653, #10027, .T. ) ;
#5344=VECTOR ( 'NONE', #781, 1000.000000000000000 ) ;
#5345=DIRECTION ( 'NONE',  ( 0.000000000000000000, 0.000000000000000000, -1.000000000000000000 ) ) ;
#5346=AXIS2_PLACEMENT_3D ( 'NONE', #12326, #2071, #1847 ) ;
#5349=FACE_OUTER_BOUND ( 'NONE', #4386, .T. ) ;
#5351=FACE_OUTER_BOUND ( 'NONE', #4241, .T. ) ;
#5352=DIRECTION ( 'NONE',  ( 0.000000000000000000, 0.000000000000000000, 1.000000000000000000 ) ) ;
#5353=ORIENTED_EDGE ( 'NONE', *, *, #2586, .F. ) ;
#5354=CIRCLE ( 'NONE', #1475, 3.000000000000002665 ) ;
#5355=LINE ( 'NONE', #8838, #10179 ) ;
#5356=DIRECTION ( 'NONE',  ( 0.000000000000000000, 0.000000000000000000, -1.000000000000000000 ) ) ;
#5359=VECTOR ( 'NONE', #5992, 1000.000000000000000 ) ;
#5360=EDGE_LOOP ( 'NONE', ( #14598, #9876, #8048, #13619, #13252, #6808, #10240, #11892, #1706, #14871 ) ) ;
#5361=EDGE_LOOP ( 'NONE', ( #6682, #4333, #1666, #6470, #8363, #589 ) ) ;
#5362=AXIS2_PLACEMENT_3D ( 'NONE', #1736, #8702, #13277 ) ;
#5363=CARTESIAN_POINT ( 'NONE',  ( 52.36539807335608288, -6.451868917687384020, -13.00000000000000178 ) ) ;
#5365=CARTESIAN_POINT ( 'NONE',  ( 51.49712671369393746, 14.70911110638358466, -10.50000000000000000 ) ) ;
#5366=ORIENTED_EDGE ( 'NONE', *, *, #8976, .T. ) ;
#5368=CIRCLE ( 'NONE', #5842, 50.00000000000000000 ) ;
#5369=EDGE_CURVE ( 'NONE', #3649, #1924, #8093, .T. ) ;
#5370=ORIENTED_EDGE ( 'NONE', *, *, #2126, .F. ) ;
#5371=AXIS2_PLACEMENT_3D ( 'NONE', #2779, #4990, #14392 ) ;
#5372=ORIENTED_EDGE ( 'NONE', *, *, #5791, .T. ) ;
#5375=CIRCLE ( 'NONE', #13867, 100.0000000000000000 ) ;
#5376=DIRECTION ( 'NONE',  ( -0.5000000000000009992, 0.000000000000000000, 0.8660254037844380415 ) ) ;
#5377=DIRECTION ( 'NONE',  ( 1.000000000000000000, 0.000000000000000000, 0.000000000000000000 ) ) ;
#5379=DIRECTION ( 'NONE',  ( 0.000000000000000000, 0.000000000000000000, 1.000000000000000000 ) ) ;
#5380=EDGE_CURVE ( 'NONE', #11838, #9110, #2212, .T. ) ;
#5381=ORIENTED_EDGE ( 'NONE', *, *, #14406, .F. ) ;
#5382=CARTESIAN_POINT ( 'NONE',  ( -6.917888187662729393, -52.54657765281195481, -13.00000000000000178 ) ) ;
#5383=CIRCLE ( 'NONE', #12872, 3.000000000000004441 ) ;
#5384=DIRECTION ( 'NONE',  ( -0.000000000000000000, -0.000000000000000000, 1.000000000000000000 ) ) ;
#5385=VERTEX_POINT ( 'NONE', #12835 ) ;
#5387=AXIS2_PLACEMENT_3D ( 'NONE', #492, #7187, #146 ) ;
#5388=ORIENTED_EDGE ( 'NONE', *, *, #5815, .T. ) ;
#5389=EDGE_CURVE ( 'NONE', #10396, #4977, #98, .T. ) ;
#5390=ORIENTED_EDGE ( 'NONE', *, *, #3061, .T. ) ;
#5392=CARTESIAN_POINT ( 'NONE',  ( -92.55687898036933348, -36.52608637591544039, -13.00000000000000178 ) ) ;
#5393=AXIS2_PLACEMENT_3D ( 'NONE', #4590, #9211, #409 ) ;
#5394=PLANE ( 'NONE',  #3283 ) ;
#5395=DIRECTION ( 'NONE',  ( -0.000000000000000000, -0.000000000000000000, -1.000000000000000000 ) ) ;
#5397=ORIENTED_EDGE ( 'NONE', *, *, #11477, .T. ) ;
#5398=FACE_OUTER_BOUND ( 'NONE', #11693, .T. ) ;
#5405=ORIENTED_EDGE ( 'NONE', *, *, #7396, .F. ) ;
#5407=ORIENTED_EDGE ( 'NONE', *, *, #13792, .F. ) ;
#5409=EDGE_CURVE ( 'NONE', #7921, #14497, #10035, .T. ) ;
#5411=AXIS2_PLACEMENT_3D ( 'NONE', #5565, #2231, #4740 ) ;
#5412=CARTESIAN_POINT ( 'NONE',  ( -33.47282819776587814, 39.30189486418276346, -13.00000000000000178 ) ) ;
#5414=EDGE_CURVE ( 'NONE', #11092, #12492, #11995, .T. ) ;
#5416=EDGE_CURVE ( 'NONE', #9373, #12974, #6379, .T. ) ;
#5418=DIRECTION ( 'NONE',  ( 0.000000000000000000, 0.000000000000000000, 1.000000000000000000 ) ) ;
#5419=CARTESIAN_POINT ( 'NONE',  ( -1.674280531759317014, 94.51066581171355097, -13.00000000000000178 ) ) ;
#5420=DIRECTION ( 'NONE',  ( 0.000000000000000000, 0.000000000000000000, 1.000000000000000000 ) ) ;
#5422=LINE ( 'NONE', #6616, #8629 ) ;
#5423=CARTESIAN_POINT ( 'NONE',  ( -89.12622059913283579, -37.21932736666236963, 10.49999999999999822 ) ) ;
#5424=AXIS2_PLACEMENT_3D ( 'NONE', #12507, #11365, #7786 ) ;
#5425=CARTESIAN_POINT ( 'NONE',  ( -37.53686968382306333, -89.89283556784496909, -13.00000000000000178 ) ) ;
#5427=DIRECTION ( 'NONE',  ( 1.000000000000000000, 0.000000000000000000, 0.000000000000000000 ) ) ;
#5428=AXIS2_PLACEMENT_3D ( 'NONE', #4527, #7848, #12499 ) ;
#5429=ORIENTED_EDGE ( 'NONE', *, *, #4882, .F. ) ;
#5430=LINE ( 'NONE', #8909, #10061 ) ;
#5431=ADVANCED_FACE ( 'NONE', ( #12614 ), #6828, .F. ) ;
#5432=FACE_OUTER_BOUND ( 'NONE', #6015, .T. ) ;
#5435=CARTESIAN_POINT ( 'NONE',  ( 89.89283556784508278, -37.53686968382275779, -10.50000000000000000 ) ) ;
#5436=DIRECTION ( 'NONE',  ( 0.000000000000000000, 0.000000000000000000, -1.000000000000000000 ) ) ;
#5437=ORIENTED_EDGE ( 'NONE', *, *, #2548, .F. ) ;
#5438=ORIENTED_EDGE ( 'NONE', *, *, #14713, .T. ) ;
#5439=APPLICATION_CONTEXT ( 'automotive_design' ) ;
#5440=AXIS2_PLACEMENT_3D ( 'NONE', #10799, #10639, #14286 ) ;
#5444=AXIS2_PLACEMENT_3D ( 'NONE', #2456, #7303, #7075 ) ;
#5445=DIRECTION ( 'NONE',  ( 1.000000000000000000, 0.000000000000000000, 0.000000000000000000 ) ) ;
#5446=VERTEX_POINT ( 'NONE', #8052 ) ;
#5447=ORIENTED_EDGE ( 'NONE', *, *, #2605, .T. ) ;
#5449=AXIS2_PLACEMENT_3D ( 'NONE', #11573, #2134, #1007 ) ;
#5450=CARTESIAN_POINT ( 'NONE',  ( 0.000000000000000000, 0.000000000000000000, -10.50000000000000000 ) ) ;
#5453=DIRECTION ( 'NONE',  ( 1.000000000000000000, 0.000000000000000000, -0.000000000000000000 ) ) ;
#5454=DIRECTION ( 'NONE',  ( -1.000000000000000000, 0.000000000000000000, 0.000000000000000000 ) ) ;
#5455=CARTESIAN_POINT ( 'NONE',  ( 52.54657765281197612, -6.917888187662545540, 10.49999999999999822 ) ) ;
#5456=ADVANCED_FACE ( 'NONE', ( #9035 ), #7902, .F. ) ;
#5457=ORIENTED_EDGE ( 'NONE', *, *, #9427, .T. ) ;
#5458=CARTESIAN_POINT ( 'NONE',  ( 26.49999999999971578, 45.89934640057541060, -8.000000000000000000 ) ) ;
#5459=ORIENTED_EDGE ( 'NONE', *, *, #10927, .T. ) ;
#5463=ORIENTED_EDGE ( 'NONE', *, *, #4452, .T. ) ;
#5464=CIRCLE ( 'NONE', #1583, 56.99999999999999289 ) ;
#5465=ORIENTED_EDGE ( 'NONE', *, *, #9257, .F. ) ;
#5466=CARTESIAN_POINT ( 'NONE',  ( 0.000000000000000000, 0.000000000000000000, -8.000000000000000000 ) ) ;
#5467=ADVANCED_FACE ( 'NONE', ( #1157 ), #5767, .F. ) ;
#5468=DIRECTION ( 'NONE',  ( 0.000000000000000000, 0.000000000000000000, -1.000000000000000000 ) ) ;
#5469=AXIS2_PLACEMENT_3D ( 'NONE', #13832, #11487, #1085 ) ;
#5470=CARTESIAN_POINT ( 'NONE',  ( 87.95718916809192933, -34.62083247296232713, -8.000000000000000000 ) ) ;
#5471=CARTESIAN_POINT ( 'NONE',  ( -39.61975340586619865, -91.27544013909722764, -13.00000000000000178 ) ) ;
#5472=VECTOR ( 'NONE', #2411, 1000.000000000000000 ) ;
#5474=EDGE_CURVE ( 'NONE', #4441, #13877, #14271, .T. ) ;
#5477=VECTOR ( 'NONE', #4311, 1000.000000000000000 ) ;
#5478=LINE ( 'NONE', #5970, #7089 ) ;
#5479=DIRECTION ( 'NONE',  ( 1.000000000000000000, 0.000000000000000000, 0.000000000000000000 ) ) ;
#5480=CIRCLE ( 'NONE', #4999, 63.00000000000000000 ) ;
#5485=ORIENTED_EDGE ( 'NONE', *, *, #9890, .T. ) ;
#5487=DIRECTION ( 'NONE',  ( 0.000000000000000000, 0.000000000000000000, 1.000000000000000000 ) ) ;
#5488=CARTESIAN_POINT ( 'NONE',  ( -70.71067811865538033, -70.71067811865414399, -8.000000000000000000 ) ) ;
#5489=PLANE ( 'NONE',  #12680 ) ;
#5490=ORIENTED_EDGE ( 'NONE', *, *, #9090, .T. ) ;
#5491=CYLINDRICAL_SURFACE ( 'NONE', #3864, 3.000000000000002665 ) ;
#5493=DIRECTION ( 'NONE',  ( 0.000000000000000000, 0.000000000000000000, 1.000000000000000000 ) ) ;
#5494=ORIENTED_EDGE ( 'NONE', *, *, #6776, .F. ) ;
#5495=CARTESIAN_POINT ( 'NONE',  ( 14.07862063237891981, -50.84834283436993729, 10.49999999999999822 ) ) ;
#5497=CARTESIAN_POINT ( 'NONE',  ( 2.649999999999993250, 38.00000000000000000, -28.00000000000000000 ) ) ;
#5500=CARTESIAN_POINT ( 'NONE',  ( 0.000000000000000000, 0.000000000000000000, 10.50000000000000000 ) ) ;
#5501=VERTEX_POINT ( 'NONE', #4946 ) ;
#5503=DIRECTION ( 'NONE',  ( -1.000000000000000000, 0.000000000000000000, 0.000000000000000000 ) ) ;
#5505=CARTESIAN_POINT ( 'NONE',  ( 0.000000000000000000, 0.000000000000000000, -8.000000000000000000 ) ) ;
#5506=CARTESIAN_POINT ( 'NONE',  ( 68.58935777509523746, 68.58935777509499587, -8.000000000000000000 ) ) ;
#5508=DIRECTION ( 'NONE',  ( -0.000000000000000000, -0.000000000000000000, 1.000000000000000000 ) ) ;
#5510=ORIENTED_EDGE ( 'NONE', *, *, #4353, .F. ) ;
#5511=VERTEX_POINT ( 'NONE', #8493 ) ;
#5512=EDGE_CURVE ( 'NONE', #8402, #4906, #4482, .T. ) ;
#5513=DIRECTION ( 'NONE',  ( 0.000000000000000000, 0.000000000000000000, 1.000000000000000000 ) ) ;
#5514=CARTESIAN_POINT ( 'NONE',  ( -33.48561063518626923, 47.21331623427104063, -8.000000000000000000 ) ) ;
#5515=ADVANCED_FACE ( 'NONE', ( #4789 ), #6137, .F. ) ;
#5517=EDGE_CURVE ( 'NONE', #10139, #5169, #591, .T. ) ;
#5520=VERTEX_POINT ( 'NONE', #2656 ) ;
#5521=EDGE_LOOP ( 'NONE', ( #6783, #4119 ) ) ;
#5525=PLANE ( 'NONE',  #13936 ) ;
#5527=CARTESIAN_POINT ( 'NONE',  ( 7.383907457638312799, 52.72775723226772726, 10.49999999999999822 ) ) ;
#5529=ORIENTED_EDGE ( 'NONE', *, *, #744, .F. ) ;
#5531=AXIS2_PLACEMENT_3D ( 'NONE', #3852, #5060, #504 ) ;
#5532=VERTEX_POINT ( 'NONE', #7048 ) ;
#5533=ORIENTED_EDGE ( 'NONE', *, *, #13805, .F. ) ;
#5534=CARTESIAN_POINT ( 'NONE',  ( 0.000000000000000000, 0.000000000000000000, -10.50000000000000000 ) ) ;
#5535=EDGE_CURVE ( 'NONE', #452, #1155, #5925, .T. ) ;
#5538=FACE_OUTER_BOUND ( 'NONE', #9666, .T. ) ;
#5540=DIRECTION ( 'NONE',  ( -0.000000000000000000, -0.000000000000000000, -1.000000000000000000 ) ) ;
#5541=EDGE_LOOP ( 'NONE', ( #5854, #115, #7185, #1180, #11132, #6034, #8608, #13472, #9928, #9938, #2639, #8375 ) ) ;
#5542=CIRCLE ( 'NONE', #9410, 52.50000000000000711 ) ;
#5543=CARTESIAN_POINT ( 'NONE',  ( 49.00442420935993226, -30.80502811811213704, -13.00000000000000178 ) ) ;
#5544=ORIENTED_EDGE ( 'NONE', *, *, #1309, .F. ) ;
#5545=CARTESIAN_POINT ( 'NONE',  ( 47.21331623427115431, 33.48561063518610581, -13.00000000000000178 ) ) ;
#5548=DIRECTION ( 'NONE',  ( 1.000000000000000000, 0.000000000000000000, 0.000000000000000000 ) ) ;
#5549=EDGE_CURVE ( 'NONE', #1483, #14940, #7616, .T. ) ;
#5550=CARTESIAN_POINT ( 'NONE',  ( 92.61631465359468507, -37.12029293941410657, -13.00000000000000178 ) ) ;
#5551=ADVANCED_FACE ( 'NONE', ( #14054 ), #7274, .F. ) ;
#5552=EDGE_LOOP ( 'NONE', ( #6982, #347, #9488, #526, #13233, #11419 ) ) ;
#5553=DIRECTION ( 'NONE',  ( -1.000000000000000000, 0.000000000000000000, 0.000000000000000000 ) ) ;
#5554=LINE ( 'NONE', #5412, #1103 ) ;
#5555=DIRECTION ( 'NONE',  ( 1.000000000000000000, 0.000000000000000000, 0.000000000000000000 ) ) ;
#5556=DIRECTION ( 'NONE',  ( 1.000000000000000000, 0.000000000000000000, -0.000000000000000000 ) ) ;
#5557=DIRECTION ( 'NONE',  ( 0.000000000000000000, 0.000000000000000000, -1.000000000000000000 ) ) ;
#5558=CARTESIAN_POINT ( 'NONE',  ( 31.05588327715836527, -44.79355920668822932, 8.000000000000000000 ) ) ;
#5560=CIRCLE ( 'NONE', #8457, 0.5000000000000022204 ) ;
#5563=CARTESIAN_POINT ( 'NONE',  ( 33.48561063518626923, -47.21331623427104063, -10.50000000000000000 ) ) ;
#5564=FACE_OUTER_BOUND ( 'NONE', #7305, .T. ) ;
#5565=CARTESIAN_POINT ( 'NONE',  ( 33.48561063518626923, -47.21331623427104063, 8.000000000000000000 ) ) ;
#5567=EDGE_CURVE ( 'NONE', #7442, #203, #12914, .T. ) ;
#5568=ORIENTED_EDGE ( 'NONE', *, *, #7560, .T. ) ;
#5570=ORIENTED_EDGE ( 'NONE', *, *, #8166, .T. ) ;
#5571=DIRECTION ( 'NONE',  ( 0.000000000000000000, 0.000000000000000000, -1.000000000000000000 ) ) ;
#5573=LINE ( 'NONE', #956, #4379 ) ;
#5575=ORIENTED_EDGE ( 'NONE', *, *, #2233, .F. ) ;
#5576=ORIENTED_EDGE ( 'NONE', *, *, #6567, .T. ) ;
#5577=ORIENTED_EDGE ( 'NONE', *, *, #6609, .T. ) ;
#5578=ORIENTED_EDGE ( 'NONE', *, *, #10051, .T. ) ;
#5579=CIRCLE ( 'NONE', #9715, 0.5000000000000004441 ) ;
#5581=CYLINDRICAL_SURFACE ( 'NONE', #13686, 0.5000000000000073275 ) ;
#5586=ORIENTED_EDGE ( 'NONE', *, *, #6664, .T. ) ;
#5588=DIRECTION ( 'NONE',  ( 0.000000000000000000, 0.000000000000000000, 1.000000000000000000 ) ) ;
#5589=AXIS2_PLACEMENT_3D ( 'NONE', #3587, #11635, #13767 ) ;
#5590=CARTESIAN_POINT ( 'NONE',  ( 0.000000000000000000, 0.000000000000000000, -10.50000000000000000 ) ) ;
#5591=CIRCLE ( 'NONE', #14082, 3.000000000000002665 ) ;
#5593=EDGE_CURVE ( 'NONE', #10072, #10139, #14419, .T. ) ;
#5596=DIRECTION ( 'NONE',  ( -0.000000000000000000, -0.000000000000000000, 1.000000000000000000 ) ) ;
#5600=CARTESIAN_POINT ( 'NONE',  ( 37.21932736666271779, -89.12622059913267947, 10.49999999999999822 ) ) ;
#5603=AXIS2_PLACEMENT_3D ( 'NONE', #14646, #8929, #3177 ) ;
#5604=VERTEX_POINT ( 'NONE', #11685 ) ;
#5605=CARTESIAN_POINT ( 'NONE',  ( 41.65105036528968441, 31.95997502295806214, -10.50000000000000000 ) ) ;
#5606=ADVANCED_FACE ( 'NONE', ( #8177 ), #3481, .T. ) ;
#5607=CYLINDRICAL_SURFACE ( 'NONE', #1006, 60.50000000000000000 ) ;
#5608=FACE_OUTER_BOUND ( 'NONE', #9729, .T. ) ;
#5609=CIRCLE ( 'NONE', #4654, 59.49999999999999289 ) ;
#5610=CARTESIAN_POINT ( 'NONE',  ( 42.04772703543530099, 32.26435573746242369, -13.00000000000000178 ) ) ;
#5613=LINE ( 'NONE', #10249, #13329 ) ;
#5614=AXIS2_PLACEMENT_3D ( 'NONE', #1106, #3675, #8151 ) ;
#5616=PLANE ( 'NONE',  #14611 ) ;
#5619=CIRCLE ( 'NONE', #2712, 50.00000000000000000 ) ;
#5620=EDGE_LOOP ( 'NONE', ( #7997, #6337, #3108, #2116, #7547, #10335 ) ) ;
#5624=CIRCLE ( 'NONE', #13389, 50.00000000000000000 ) ;
#5625=CARTESIAN_POINT ( 'NONE',  ( 89.61631465359491244, 37.12029293941346708, -13.00000000000000178 ) ) ;
#5626=CARTESIAN_POINT ( 'NONE',  ( 68.58935777509523746, 68.58935777509499587, 10.49999999999999822 ) ) ;
#5627=CARTESIAN_POINT ( 'NONE',  ( -87.95718916809170196, 34.62083247296289557, -8.000000000000000000 ) ) ;
#5628=CARTESIAN_POINT ( 'NONE',  ( 71.53347797788772766, 69.16568774265620334, 8.000000000000000000 ) ) ;
#5629=CARTESIAN_POINT ( 'NONE',  ( -12.86891638962156215, 56.43380494353993271, -13.00000000000000178 ) ) ;
#5630=AXIS2_PLACEMENT_3D ( 'NONE', #10512, #2462, #9222 ) ;
#5632=EDGE_CURVE ( 'NONE', #5663, #11040, #9318, .T. ) ;
#5634=EDGE_CURVE ( 'NONE', #7442, #1613, #6885, .T. ) ;
#5635=VERTEX_POINT ( 'NONE', #1198 ) ;
#5636=EDGE_CURVE ( 'NONE', #12743, #13570, #1093, .T. ) ;
#5637=AXIS2_PLACEMENT_3D ( 'NONE', #10428, #10581, #10282 ) ;
#5638=DIRECTION ( 'NONE',  ( -1.000000000000000000, 1.826024711554534406E-15, 0.000000000000000000 ) ) ;
#5639=FACE_OUTER_BOUND ( 'NONE', #1411, .T. ) ;
#5640=CARTESIAN_POINT ( 'NONE',  ( -46.24878538001294004, 27.00670028307212078, -10.50000000000000000 ) ) ;
#5641=ORIENTED_EDGE ( 'NONE', *, *, #5016, .T. ) ;
#5643=CIRCLE ( 'NONE', #12922, 3.000000000000002665 ) ;
#5644=ORIENTED_EDGE ( 'NONE', *, *, #10561, .F. ) ;
#5645=EDGE_CURVE ( 'NONE', #14119, #9063, #9548, .T. ) ;
#5646=CARTESIAN_POINT ( 'NONE',  ( 2.449293598294700991E-16, -97.00000000000000000, -13.00000000000000178 ) ) ;
#5647=ORIENTED_EDGE ( 'NONE', *, *, #4734, .F. ) ;
#5648=AXIS2_PLACEMENT_3D ( 'NONE', #9570, #1459, #8580 ) ;
#5650=DIRECTION ( 'NONE',  ( 0.000000000000000000, 0.000000000000000000, -1.000000000000000000 ) ) ;
#5651=CIRCLE ( 'NONE', #3229, 3.000000000000002665 ) ;
#5652=DIRECTION ( 'NONE',  ( 0.000000000000000000, 0.000000000000000000, 1.000000000000000000 ) ) ;
#5653=DIRECTION ( 'NONE',  ( -1.000000000000000000, 0.000000000000000000, 0.000000000000000000 ) ) ;
#5654=VERTEX_POINT ( 'NONE', #8247 ) ;
#5655=ADVANCED_FACE ( 'NONE', ( #11544 ), #11611, .F. ) ;
#5656=VERTEX_POINT ( 'NONE', #1059 ) ;
#5657=VERTEX_POINT ( 'NONE', #4621 ) ;
#5658=CIRCLE ( 'NONE', #10748, 60.50000000000000000 ) ;
#5660=DIRECTION ( 'NONE',  ( 0.000000000000000000, 0.000000000000000000, 1.000000000000000000 ) ) ;
#5661=CARTESIAN_POINT ( 'NONE',  ( -30.80502811811232888, -49.00442420935981147, -10.50000000000000000 ) ) ;
#5662=CARTESIAN_POINT ( 'NONE',  ( -45.39934640057513349, 26.50000000000019540, -10.50000000000000000 ) ) ;
#5663=VERTEX_POINT ( 'NONE', #7020 ) ;
#5664=CIRCLE ( 'NONE', #14152, 63.00000000000000000 ) ;
#5666=VERTEX_POINT ( 'NONE', #12888 ) ;
#5669=DIRECTION ( 'NONE',  ( -1.000000000000000000, 0.000000000000000000, 0.000000000000000000 ) ) ;
#5670=DIRECTION ( 'NONE',  ( -1.000000000000000000, 0.000000000000000000, 0.000000000000000000 ) ) ;
#5671=CIRCLE ( 'NONE', #7361, 59.50000000000000711 ) ;
#5672=AXIS2_PLACEMENT_3D ( 'NONE', #7451, #12102, #1694 ) ;
#5674=FACE_OUTER_BOUND ( 'NONE', #12953, .T. ) ;
#5675=ORIENTED_EDGE ( 'NONE', *, *, #5877, .F. ) ;
#5677=CARTESIAN_POINT ( 'NONE',  ( 0.000000000000000000, 0.000000000000000000, 8.000000000000000000 ) ) ;
#5680=CARTESIAN_POINT ( 'NONE',  ( 92.38795325112852197, -38.26834323650938074, 8.000000000000000000 ) ) ;
#5681=EDGE_CURVE ( 'NONE', #5962, #6738, #3751, .T. ) ;
#5682=VECTOR ( 'NONE', #3875, 1000.000000000000000 ) ;
#5683=CARTESIAN_POINT ( 'NONE',  ( -32.26435573746199736, 42.04772703543562073, 10.49999999999999822 ) ) ;
#5684=DIRECTION ( 'NONE',  ( -1.000000000000000000, 0.000000000000000000, 0.000000000000000000 ) ) ;
#5685=CARTESIAN_POINT ( 'NONE',  ( 72.70695371924547601, 57.06275842387054098, -8.000000000000000000 ) ) ;
#5687=AXIS2_PLACEMENT_3D ( 'NONE', #9460, #14108, #11837 ) ;
#5688=FACE_OUTER_BOUND ( 'NONE', #4045, .T. ) ;
#5690=VECTOR ( 'NONE', #11830, 1000.000000000000000 ) ;
#5691=LINE ( 'NONE', #10327, #8262 ) ;
#5694=CARTESIAN_POINT ( 'NONE',  ( 0.000000000000000000, 0.000000000000000000, -10.50000000000000000 ) ) ;
#5696=ORIENTED_EDGE ( 'NONE', *, *, #6502, .F. ) ;
#5697=CYLINDRICAL_SURFACE ( 'NONE', #8596, 56.99999999999999289 ) ;
#5699=EDGE_CURVE ( 'NONE', #7929, #10605, #14953, .T. ) ;
#5700=AXIS2_PLACEMENT_3D ( 'NONE', #4943, #14125, #1598 ) ;
#5703=DIRECTION ( 'NONE',  ( 0.000000000000000000, 0.000000000000000000, 1.000000000000000000 ) ) ;
#5704=AXIS2_PLACEMENT_3D ( 'NONE', #6355, #2658, #616 ) ;
#5706=CARTESIAN_POINT ( 'NONE',  ( 0.000000000000000000, 0.000000000000000000, 13.00000000000000178 ) ) ;
#5707=CYLINDRICAL_SURFACE ( 'NONE', #3465, 3.000000000000002665 ) ;
#5709=PLANE ( 'NONE',  #14283 ) ;
#5710=AXIS2_PLACEMENT_3D ( 'NONE', #6794, #11680, #11457 ) ;
#5712=AXIS2_PLACEMENT_3D ( 'NONE', #8871, #5238, #7430 ) ;
#5713=EDGE_LOOP ( 'NONE', ( #3683, #10600, #13712, #8408 ) ) ;
#5717=DIRECTION ( 'NONE',  ( -1.000000000000000000, -4.625929269271481378E-15, 0.000000000000000000 ) ) ;
#5718=ORIENTED_EDGE ( 'NONE', *, *, #10613, .T. ) ;
#5719=AXIS2_PLACEMENT_3D ( 'NONE', #11443, #5660, #13793 ) ;
#5720=CYLINDRICAL_SURFACE ( 'NONE', #11196, 3.000000000000002665 ) ;
#5721=EDGE_LOOP ( 'NONE', ( #14078, #7150, #10060, #4284 ) ) ;
#5722=EDGE_CURVE ( 'NONE', #12796, #14448, #2399, .T. ) ;
#5723=DIRECTION ( 'NONE',  ( 1.000000000000000000, 0.000000000000000000, 0.000000000000000000 ) ) ;
#5724=EDGE_CURVE ( 'NONE', #9289, #7921, #8107, .T. ) ;
#5725=DIRECTION ( 'NONE',  ( -0.000000000000000000, -0.000000000000000000, -1.000000000000000000 ) ) ;
#5726=CARTESIAN_POINT ( 'NONE',  ( -11.55014193876141171, 53.26842454702440222, -13.00000000000000178 ) ) ;
#5727=ORIENTED_EDGE ( 'NONE', *, *, #13393, .F. ) ;
#5729=ORIENTED_EDGE ( 'NONE', *, *, #10091, .F. ) ;
#5731=AXIS2_PLACEMENT_3D ( 'NONE', #10635, #9495, #5097 ) ;
#5733=DIRECTION ( 'NONE',  ( 1.000000000000000000, 0.000000000000000000, 0.000000000000000000 ) ) ;
#5734=DIRECTION ( 'NONE',  ( -1.000000000000000000, 0.000000000000000000, 0.000000000000000000 ) ) ;
#5735=ORIENTED_EDGE ( 'NONE', *, *, #206, .F. ) ;
#5737=EDGE_CURVE ( 'NONE', #7405, #9994, #8543, .T. ) ;
#5739=EDGE_CURVE ( 'NONE', #3649, #12421, #6188, .T. ) ;
#5740=CIRCLE ( 'NONE', #4540, 60.50000000000000000 ) ;
#5741=DIRECTION ( 'NONE',  ( -0.000000000000000000, -0.000000000000000000, 1.000000000000000000 ) ) ;
#5743=DIRECTION ( 'NONE',  ( -1.000000000000000000, 0.000000000000000000, 0.000000000000000000 ) ) ;
#5746=CARTESIAN_POINT ( 'NONE',  ( -12.86891638962156215, 56.43380494353993271, -10.50000000000000000 ) ) ;
#5748=EDGE_CURVE ( 'NONE', #3199, #9900, #10045, .T. ) ;
#5749=CARTESIAN_POINT ( 'NONE',  ( 37.12029293941315444, -89.61631465359504034, 8.000000000000000000 ) ) ;
#5753=DIRECTION ( 'NONE',  ( 0.000000000000000000, 0.000000000000000000, -1.000000000000000000 ) ) ;
#5754=VERTEX_POINT ( 'NONE', #2788 ) ;
#5755=ADVANCED_FACE ( 'NONE', ( #5059 ), #3930, .T. ) ;
#5756=VERTEX_POINT ( 'NONE', #11987 ) ;
#5758=CARTESIAN_POINT ( 'NONE',  ( -31.76435573746199381, 42.04772703543562073, 10.49999999999999822 ) ) ;
#5759=FACE_OUTER_BOUND ( 'NONE', #5620, .T. ) ;
#5763=DIRECTION ( 'NONE',  ( -0.000000000000000000, -0.000000000000000000, 1.000000000000000000 ) ) ;
#5764=CARTESIAN_POINT ( 'NONE',  ( 0.000000000000000000, 0.000000000000000000, -10.50000000000000000 ) ) ;
#5765=EDGE_LOOP ( 'NONE', ( #14775, #6222, #2863, #8209 ) ) ;
#5766=DIRECTION ( 'NONE',  ( -1.000000000000000000, 0.000000000000000000, 0.000000000000000000 ) ) ;
#5767=CYLINDRICAL_SURFACE ( 'NONE', #12489, 0.5000000000000004441 ) ;
#5768=CARTESIAN_POINT ( 'NONE',  ( 32.26435573746228158, -42.04772703543541468, 8.000000000000000000 ) ) ;
#5769=DIRECTION ( 'NONE',  ( -1.000000000000000000, 0.000000000000000000, 0.000000000000000000 ) ) ;
#5770=DIRECTION ( 'NONE',  ( -0.000000000000000000, -0.000000000000000000, 1.000000000000000000 ) ) ;
#5772=EDGE_CURVE ( 'NONE', #12974, #13772, #9667, .T. ) ;
#5774=ADVANCED_FACE ( 'NONE', ( #10601 ), #14252, .T. ) ;
#5776=EDGE_CURVE ( 'NONE', #8180, #5501, #14433, .T. ) ;
#5777=VERTEX_POINT ( 'NONE', #2857 ) ;
#5779=DIRECTION ( 'NONE',  ( 0.000000000000000000, 0.000000000000000000, 1.000000000000000000 ) ) ;
#5780=DIRECTION ( 'NONE',  ( 1.000000000000000000, 0.000000000000000000, 0.000000000000000000 ) ) ;
#5782=FACE_OUTER_BOUND ( 'NONE', #2966, .T. ) ;
#5783=ORIENTED_EDGE ( 'NONE', *, *, #1875, .T. ) ;
#5784=DIRECTION ( 'NONE',  ( 1.000000000000000000, 0.000000000000000000, 0.000000000000000000 ) ) ;
#5785=ORIENTED_EDGE ( 'NONE', *, *, #13538, .T. ) ;
#5786=EDGE_CURVE ( 'NONE', #7296, #14250, #12250, .T. ) ;
#5787=CARTESIAN_POINT ( 'NONE',  ( -30.80502811811232888, -49.00442420935981147, -13.00000000000000178 ) ) ;
#5789=DIRECTION ( 'NONE',  ( 0.000000000000000000, 0.000000000000000000, 1.000000000000000000 ) ) ;
#5790=DIRECTION ( 'NONE',  ( 0.000000000000000000, 0.000000000000000000, 1.000000000000000000 ) ) ;
#5791=EDGE_CURVE ( 'NONE', #11551, #13490, #9811, .T. ) ;
#5795=LINE ( 'NONE', #13870, #608 ) ;
#5796=CARTESIAN_POINT ( 'NONE',  ( 0.000000000000000000, 0.000000000000000000, 8.000000000000000000 ) ) ;
#5797=ORIENTED_EDGE ( 'NONE', *, *, #12138, .F. ) ;
#5799=ORIENTED_EDGE ( 'NONE', *, *, #2576, .T. ) ;
#5800=ORIENTED_EDGE ( 'NONE', *, *, #7393, .T. ) ;
#5802=AXIS2_PLACEMENT_3D ( 'NONE', #6083, #10868, #14367 ) ;
#5803=CARTESIAN_POINT ( 'NONE',  ( -50.00000000000000000, 0.000000000000000000, -8.000000000000000000 ) ) ;
#5806=AXIS2_PLACEMENT_3D ( 'NONE', #11660, #12859, #31 ) ;
#5807=CARTESIAN_POINT ( 'NONE',  ( 51.19406879332056093, 13.71740939043382745, 10.49999999999999822 ) ) ;
#5810=VERTEX_POINT ( 'NONE', #10899 ) ;
#5812=VERTEX_POINT ( 'NONE', #2710 ) ;
#5813=CARTESIAN_POINT ( 'NONE',  ( 0.000000000000000000, 0.000000000000000000, 8.000000000000000000 ) ) ;
#5814=DIRECTION ( 'NONE',  ( -1.000000000000000000, 0.000000000000000000, 0.000000000000000000 ) ) ;
#5815=EDGE_CURVE ( 'NONE', #9297, #6889, #1581, .T. ) ;
#5816=EDGE_CURVE ( 'NONE', #9608, #1839, #7244, .T. ) ;
#5818=VECTOR ( 'NONE', #8055, 1000.000000000000000 ) ;
#5819=EDGE_CURVE ( 'NONE', #13345, #14403, #5211, .T. ) ;
#5820=ORIENTED_EDGE ( 'NONE', *, *, #1248, .F. ) ;
#5821=FACE_OUTER_BOUND ( 'NONE', #9284, .T. ) ;
#5822=CIRCLE ( 'NONE', #7763, 0.5000000000000022204 ) ;
#5823=ORIENTED_EDGE ( 'NONE', *, *, #2963, .F. ) ;
#5824=VERTEX_POINT ( 'NONE', #199 ) ;
#5827=EDGE_CURVE ( 'NONE', #12589, #7227, #14101, .T. ) ;
#5830=CYLINDRICAL_SURFACE ( 'NONE', #11656, 63.00000000000000000 ) ;
#5831=CIRCLE ( 'NONE', #1724, 100.0000000000000000 ) ;
#5832=VECTOR ( 'NONE', #3187, 1000.000000000000000 ) ;
#5833=CARTESIAN_POINT ( 'NONE',  ( 71.58935777509475429, -68.58935777509547904, 8.000000000000000000 ) ) ;
#5835=VECTOR ( 'NONE', #4468, 1000.000000000000000 ) ;
#5836=CARTESIAN_POINT ( 'NONE',  ( -33.49014761921588956, 11.74264578624790190, -28.00000000000000000 ) ) ;
#5837=VERTEX_POINT ( 'NONE', #8323 ) ;
#5839=DIRECTION ( 'NONE',  ( -0.000000000000000000, -0.000000000000000000, 1.000000000000000000 ) ) ;
#5841=DIRECTION ( 'NONE',  ( 0.000000000000000000, 0.000000000000000000, 1.000000000000000000 ) ) ;
#5842=AXIS2_PLACEMENT_3D ( 'NONE', #5231, #6427, #14492 ) ;
#5843=DIRECTION ( 'NONE',  ( 0.000000000000000000, 0.000000000000000000, 1.000000000000000000 ) ) ;
#5844=LINE ( 'NONE', #10483, #7024 ) ;
#5845=AXIS2_PLACEMENT_3D ( 'NONE', #2904, #7521, #12039 ) ;
#5846=AXIS2_PLACEMENT_3D ( 'NONE', #1922, #7768, #6699 ) ;
#5847=DIRECTION ( 'NONE',  ( 0.000000000000000000, 0.000000000000000000, -1.000000000000000000 ) ) ;
#5848=DIRECTION ( 'NONE',  ( -1.000000000000000000, 0.000000000000000000, 0.000000000000000000 ) ) ;
#5849=DIRECTION ( 'NONE',  ( -0.000000000000000000, -0.000000000000000000, 1.000000000000000000 ) ) ;
#5852=DIRECTION ( 'NONE',  ( -1.000000000000000000, 0.000000000000000000, 0.000000000000000000 ) ) ;
#5853=AXIS2_PLACEMENT_3D ( 'NONE', #7093, #2907, #6302 ) ;
#5854=ORIENTED_EDGE ( 'NONE', *, *, #12793, .F. ) ;
#5857=DIRECTION ( 'NONE',  ( 0.000000000000000000, 0.000000000000000000, 1.000000000000000000 ) ) ;
#5858=AXIS2_PLACEMENT_3D ( 'NONE', #4487, #991, #9103 ) ;
#5859=DIRECTION ( 'NONE',  ( 1.000000000000000000, 0.000000000000000000, 0.000000000000000000 ) ) ;
#5860=DIRECTION ( 'NONE',  ( 1.000000000000000000, 0.000000000000000000, 0.000000000000000000 ) ) ;
#5861=ORIENTED_EDGE ( 'NONE', *, *, #12371, .T. ) ;
#5862=EDGE_CURVE ( 'NONE', #1935, #4441, #3036, .T. ) ;
#5864=ORIENTED_EDGE ( 'NONE', *, *, #348, .F. ) ;
#5865=DIRECTION ( 'NONE',  ( 0.000000000000000000, 0.000000000000000000, 1.000000000000000000 ) ) ;
#5869=DIRECTION ( 'NONE',  ( 0.000000000000000000, 0.000000000000000000, 1.000000000000000000 ) ) ;
#5870=VERTEX_POINT ( 'NONE', #6245 ) ;
#5871=DIRECTION ( 'NONE',  ( 1.000000000000000000, 0.000000000000000000, 0.000000000000000000 ) ) ;
#5873=VECTOR ( 'NONE', #8163, 1000.000000000000000 ) ;
#5874=DIRECTION ( 'NONE',  ( 0.000000000000000000, 0.000000000000000000, -1.000000000000000000 ) ) ;
#5876=VERTEX_POINT ( 'NONE', #8459 ) ;
#5877=EDGE_CURVE ( 'NONE', #7439, #14780, #1487, .T. ) ;
#5878=EDGE_CURVE ( 'NONE', #8551, #6323, #368, .T. ) ;
#5879=AXIS2_PLACEMENT_3D ( 'NONE', #3621, #13801, #12807 ) ;
#5880=ORIENTED_EDGE ( 'NONE', *, *, #3255, .T. ) ;
#5881=CARTESIAN_POINT ( 'NONE',  ( 36.52608637591580987, -92.55687898036916295, -13.00000000000000178 ) ) ;
#5882=AXIS2_PLACEMENT_3D ( 'NONE', #14221, #9498, #4806 ) ;
#5883=DIRECTION ( 'NONE',  ( 0.000000000000000000, 0.000000000000000000, 1.000000000000000000 ) ) ;
#5886=CARTESIAN_POINT ( 'NONE',  ( -30.80502811811232888, -49.00442420935981147, -13.00000000000000178 ) ) ;
#5887=CARTESIAN_POINT ( 'NONE',  ( -33.48561063518626923, 47.21331623427104063, 8.000000000000000000 ) ) ;
#5888=AXIS2_PLACEMENT_3D ( 'NONE', #10796, #2827, #7508 ) ;
#5889=VERTEX_POINT ( 'NONE', #2701 ) ;
#5890=DIRECTION ( 'NONE',  ( 0.000000000000000000, 0.000000000000000000, 1.000000000000000000 ) ) ;
#5893=VERTEX_POINT ( 'NONE', #9824 ) ;
#5895=EDGE_LOOP ( 'NONE', ( #12402, #39, #6499, #4308, #10141, #12752 ) ) ;
#5896=DIRECTION ( 'NONE',  ( -0.000000000000000000, -0.000000000000000000, 1.000000000000000000 ) ) ;
#5897=ORIENTED_EDGE ( 'NONE', *, *, #13274, .F. ) ;
#5899=AXIS2_PLACEMENT_3D ( 'NONE', #8956, #7597, #7512 ) ;
#5900=DIRECTION ( 'NONE',  ( 1.000000000000000000, 0.000000000000000000, 0.000000000000000000 ) ) ;
#5901=CYLINDRICAL_SURFACE ( 'NONE', #2467, 60.50000000000000000 ) ;
#5902=CIRCLE ( 'NONE', #7109, 60.50000000000000000 ) ;
#5903=EDGE_CURVE ( 'NONE', #7149, #2085, #14469, .T. ) ;
#5904=DIRECTION ( 'NONE',  ( 0.000000000000000000, 0.000000000000000000, -1.000000000000000000 ) ) ;
#5906=CARTESIAN_POINT ( 'NONE',  ( 92.61631465359491244, 37.12029293941346708, -8.000000000000000000 ) ) ;
#5907=EDGE_CURVE ( 'NONE', #571, #14147, #14186, .T. ) ;
#5911=CIRCLE ( 'NONE', #14408, 60.50000000000000711 ) ;
#5912=CIRCLE ( 'NONE', #561, 3.000000000000002665 ) ;
#5913=EDGE_CURVE ( 'NONE', #7348, #4331, #12051, .T. ) ;
#5914=CIRCLE ( 'NONE', #7855, 3.000000000000002665 ) ;
#5916=DIRECTION ( 'NONE',  ( -0.000000000000000000, -0.000000000000000000, 1.000000000000000000 ) ) ;
#5917=EDGE_LOOP ( 'NONE', ( #10680, #3935, #13780, #1921, #5153 ) ) ;
#5918=DIRECTION ( 'NONE',  ( 1.000000000000000000, 0.000000000000000000, 0.000000000000000000 ) ) ;
#5919=ADVANCED_FACE ( 'NONE', ( #11893 ), #7397, .F. ) ;
#5920=VECTOR ( 'NONE', #2372, 1000.000000000000000 ) ;
#5921=ADVANCED_FACE ( 'NONE', ( #10822 ), #14309, .T. ) ;
#5925=CIRCLE ( 'NONE', #10774, 0.5000000000000073275 ) ;
#5926=AXIS2_PLACEMENT_3D ( 'NONE', #9219, #11666, #3380 ) ;
#5927=AXIS2_PLACEMENT_3D ( 'NONE', #9154, #4682, #1189 ) ;
#5928=FACE_OUTER_BOUND ( 'NONE', #1350, .T. ) ;
#5929=DIRECTION ( 'NONE',  ( 1.000000000000000000, 5.329070518200751394E-15, 0.000000000000000000 ) ) ;
#5930=ORIENTED_EDGE ( 'NONE', *, *, #3100, .T. ) ;
#5933=LINE ( 'NONE', #14914, #4691 ) ;
#5936=CIRCLE ( 'NONE', #119, 3.000000000000002665 ) ;
#5937=AXIS2_PLACEMENT_3D ( 'NONE', #5626, #7682, #4206 ) ;
#5938=CARTESIAN_POINT ( 'NONE',  ( -56.43380494354004639, -12.86891638962099549, -10.50000000000000000 ) ) ;
#5939=ORIENTED_EDGE ( 'NONE', *, *, #13742, .T. ) ;
#5945=DIRECTION ( 'NONE',  ( -1.000000000000000000, -1.198854274490189999E-13, 0.000000000000000000 ) ) ;
#5946=CARTESIAN_POINT ( 'NONE',  ( -37.12029293941441210, -89.61631465359452875, -8.000000000000000000 ) ) ;
#5948=DIRECTION ( 'NONE',  ( -1.000000000000000000, 0.000000000000000000, 0.000000000000000000 ) ) ;
#5949=FACE_OUTER_BOUND ( 'NONE', #7384, .T. ) ;
#5950=CARTESIAN_POINT ( 'NONE',  ( 33.48561063518626923, -47.21331623427104063, -13.00000000000000178 ) ) ;
#5951=VERTEX_POINT ( 'NONE', #491 ) ;
#5952=AXIS2_PLACEMENT_3D ( 'NONE', #8033, #4625, #3713 ) ;
#5953=VERTEX_POINT ( 'NONE', #5052 ) ;
#5954=VERTEX_POINT ( 'NONE', #6317 ) ;
#5955=DIRECTION ( 'NONE',  ( -1.000000000000000000, 0.000000000000000000, 0.000000000000000000 ) ) ;
#5956=CYLINDRICAL_SURFACE ( 'NONE', #8031, 63.00000000000000000 ) ;
#5959=CIRCLE ( 'NONE', #7173, 3.000000000000002665 ) ;
#5960=EDGE_CURVE ( 'NONE', #914, #11061, #4741, .T. ) ;
#5961=ORIENTED_EDGE ( 'NONE', *, *, #8522, .F. ) ;
#5962=VERTEX_POINT ( 'NONE', #13319 ) ;
#5966=ORIENTED_EDGE ( 'NONE', *, *, #3569, .F. ) ;
#5967=EDGE_CURVE ( 'NONE', #12052, #11984, #607, .T. ) ;
#5968=DIRECTION ( 'NONE',  ( 1.000000000000000000, 0.000000000000000000, 0.000000000000000000 ) ) ;
#5969=CYLINDRICAL_SURFACE ( 'NONE', #7455, 60.50000000000000000 ) ;
#5970=CARTESIAN_POINT ( 'NONE',  ( 7.383907457638312799, 52.72775723226772726, -13.00000000000000178 ) ) ;
#5972=ORIENTED_EDGE ( 'NONE', *, *, #13417, .T. ) ;
#5973=CARTESIAN_POINT ( 'NONE',  ( -12.86891638962156215, 56.43380494353993271, 8.000000000000000000 ) ) ;
#5974=AXIS2_PLACEMENT_3D ( 'NONE', #5317, #695, #8725 ) ;
#5975=EDGE_LOOP ( 'NONE', ( #832, #2142, #3274, #11881, #2800 ) ) ;
#5976=DIRECTION ( 'NONE',  ( 1.000000000000000000, 0.000000000000000000, 0.000000000000000000 ) ) ;
#5978=DIRECTION ( 'NONE',  ( -1.000000000000000000, 0.000000000000000000, 0.000000000000000000 ) ) ;
#5979=DIRECTION ( 'NONE',  ( 1.000000000000000000, 0.000000000000000000, 0.000000000000000000 ) ) ;
#5981=DIRECTION ( 'NONE',  ( -1.000000000000000000, 0.000000000000000000, 0.000000000000000000 ) ) ;
#5985=ORIENTED_EDGE ( 'NONE', *, *, #12293, .F. ) ;
#5988=VERTEX_POINT ( 'NONE', #3920 ) ;
#5991=FACE_OUTER_BOUND ( 'NONE', #9621, .T. ) ;
#5992=DIRECTION ( 'NONE',  ( 0.000000000000000000, 0.000000000000000000, 1.000000000000000000 ) ) ;
#5993=CARTESIAN_POINT ( 'NONE',  ( -49.00442420935969778, 30.80502811811250297, 10.49999999999999822 ) ) ;
#5994=CARTESIAN_POINT ( 'NONE',  ( 89.61631465359468507, -37.12029293941410657, 10.49999999999999822 ) ) ;
#5995=ORIENTED_EDGE ( 'NONE', *, *, #4698, .T. ) ;
#5996=DIRECTION ( 'NONE',  ( 1.000000000000000000, 0.000000000000000000, 0.000000000000000000 ) ) ;
#5997=VERTEX_POINT ( 'NONE', #14244 ) ;
#5998=CARTESIAN_POINT ( 'NONE',  ( 37.02125851216354846, -90.10640870805738700, -13.00000000000000178 ) ) ;
#6000=ADVANCED_FACE ( 'NONE', ( #7318 ), #13544, .F. ) ;
#6001=VECTOR ( 'NONE', #1200, 1000.000000000000000 ) ;
#6002=ADVANCED_FACE ( 'NONE', ( #7697 ), #6768, .F. ) ;
#6005=EDGE_CURVE ( 'NONE', #8680, #198, #5936, .T. ) ;
#6007=CARTESIAN_POINT ( 'NONE',  ( 53.26842454702428142, 11.55014193876197126, -8.000000000000000000 ) ) ;
#6009=ORIENTED_EDGE ( 'NONE', *, *, #5645, .F. ) ;
#6010=CARTESIAN_POINT ( 'NONE',  ( 0.000000000000000000, 0.000000000000000000, -13.00000000000000178 ) ) ;
#6011=DIRECTION ( 'NONE',  ( 1.000000000000000000, 0.000000000000000000, 0.000000000000000000 ) ) ;
#6013=DIRECTION ( 'NONE',  ( 1.000000000000000000, 0.000000000000000000, 0.000000000000000000 ) ) ;
#6015=EDGE_LOOP ( 'NONE', ( #12579, #116, #2466, #10217 ) ) ;
#6016=DIRECTION ( 'NONE',  ( 0.000000000000000000, 0.000000000000000000, 1.000000000000000000 ) ) ;
#6017=DIRECTION ( 'NONE',  ( -1.000000000000000000, 0.000000000000000000, 0.000000000000000000 ) ) ;
#6020=ORIENTED_EDGE ( 'NONE', *, *, #1398, .F. ) ;
#6021=AXIS2_PLACEMENT_3D ( 'NONE', #12157, #7435, #1452 ) ;
#6022=ORIENTED_EDGE ( 'NONE', *, *, #11662, .F. ) ;
#6023=DIRECTION ( 'NONE',  ( 0.000000000000000000, 0.000000000000000000, -1.000000000000000000 ) ) ;
#6024=DIRECTION ( 'NONE',  ( 0.000000000000000000, 0.000000000000000000, 1.000000000000000000 ) ) ;
#6027=ORIENTED_EDGE ( 'NONE', *, *, #6611, .T. ) ;
#6029=ORIENTED_EDGE ( 'NONE', *, *, #10659, .F. ) ;
#6031=VECTOR ( 'NONE', #11858, 1000.000000000000000 ) ;
#6032=CARTESIAN_POINT ( 'NONE',  ( -3.492805317593278058, 46.55633131742322917, -10.50000000000000000 ) ) ;
#6033=DIRECTION ( 'NONE',  ( 0.000000000000000000, 0.000000000000000000, 1.000000000000000000 ) ) ;
#6034=ORIENTED_EDGE ( 'NONE', *, *, #13624, .T. ) ;
#6035=ORIENTED_EDGE ( 'NONE', *, *, #6274, .T. ) ;
#6036=CYLINDRICAL_SURFACE ( 'NONE', #11026, 100.0000000000000000 ) ;
#6037=ORIENTED_EDGE ( 'NONE', *, *, #3161, .T. ) ;
#6038=VECTOR ( 'NONE', #6294, 1000.000000000000000 ) ;
#6039=EDGE_CURVE ( 'NONE', #2732, #6497, #5430, .T. ) ;
#6043=EDGE_CURVE ( 'NONE', #14940, #5135, #12016, .T. ) ;
#6044=AXIS2_PLACEMENT_3D ( 'NONE', #5309, #14503, #4103 ) ;
#6046=LINE ( 'NONE', #10543, #10196 ) ;
#6047=CARTESIAN_POINT ( 'NONE',  ( -49.00442420935969778, 30.80502811811250297, -10.50000000000000000 ) ) ;
#6050=ORIENTED_EDGE ( 'NONE', *, *, #9543, .T. ) ;
#6051=CYLINDRICAL_SURFACE ( 'NONE', #2418, 56.99999999999999289 ) ;
#6052=AXIS2_PLACEMENT_3D ( 'NONE', #8796, #763, #13435 ) ;
#6054=ORIENTED_EDGE ( 'NONE', *, *, #5139, .T. ) ;
#6055=VECTOR ( 'NONE', #6298, 1000.000000000000000 ) ;
#6059=CARTESIAN_POINT ( 'NONE',  ( -56.43380494354004639, -12.86891638962099549, -8.000000000000000000 ) ) ;
#6061=ADVANCED_FACE ( 'NONE', ( #3082 ), #11124, .T. ) ;
#6062=DIRECTION ( 'NONE',  ( 0.000000000000000000, 0.000000000000000000, 1.000000000000000000 ) ) ;
#6063=AXIS2_PLACEMENT_3D ( 'NONE', #8722, #6589, #10100 ) ;
#6065=CARTESIAN_POINT ( 'NONE',  ( -33.48561063518626923, 47.21331623427104063, -8.000000000000000000 ) ) ;
#6066=DIRECTION ( 'NONE',  ( 1.000000000000000000, 0.000000000000000000, 0.000000000000000000 ) ) ;
#6067=FACE_OUTER_BOUND ( 'NONE', #14436, .T. ) ;
#6068=CIRCLE ( 'NONE', #14080, 50.00000000000000000 ) ;
#6069=CARTESIAN_POINT ( 'NONE',  ( 33.47282819776613394, -39.30189486418255740, -8.000000000000000000 ) ) ;
#6071=EDGE_LOOP ( 'NONE', ( #11836, #4164, #13029, #2550 ) ) ;
#6073=ORIENTED_EDGE ( 'NONE', *, *, #14425, .F. ) ;
#6074=VECTOR ( 'NONE', #2201, 1000.000000000000000 ) ;
#6076=LINE ( 'NONE', #3823, #1773 ) ;
#6077=AXIS2_PLACEMENT_3D ( 'NONE', #13737, #10450, #10307 ) ;
#6080=CARTESIAN_POINT ( 'NONE',  ( 36.70371619500516402, 89.33979373934434420, 10.49999999999999822 ) ) ;
#6081=AXIS2_PLACEMENT_3D ( 'NONE', #25, #9283, #13937 ) ;
#6082=ORIENTED_EDGE ( 'NONE', *, *, #9654, .F. ) ;
#6083=CARTESIAN_POINT ( 'NONE',  ( 2.449293598294700991E-16, -97.00000000000000000, 8.000000000000000000 ) ) ;
#6086=DIRECTION ( 'NONE',  ( 1.000000000000000000, 0.000000000000000000, 0.000000000000000000 ) ) ;
#6087=DIRECTION ( 'NONE',  ( 0.000000000000000000, 0.000000000000000000, 1.000000000000000000 ) ) ;
#6088=EDGE_CURVE ( 'NONE', #5824, #1620, #4013, .T. ) ;
#6089=AXIS2_PLACEMENT_3D ( 'NONE', #6981, #8063, #13 ) ;
#6090=CARTESIAN_POINT ( 'NONE',  ( -47.21331623427138879, -33.48561063518577896, -10.50000000000000000 ) ) ;
#6093=EDGE_LOOP ( 'NONE', ( #14197, #7471, #6272, #5785, #12288 ) ) ;
#6094=AXIS2_PLACEMENT_3D ( 'NONE', #11056, #4706, #7108 ) ;
#6095=EDGE_LOOP ( 'NONE', ( #4474, #10084, #7049, #4567 ) ) ;
#6096=DIRECTION ( 'NONE',  ( 1.000000000000000000, 0.000000000000000000, 0.000000000000000000 ) ) ;
#6098=CARTESIAN_POINT ( 'NONE',  ( 68.09867107462983427, 68.49330278050145182, 10.49999999999999822 ) ) ;
#6099=EDGE_CURVE ( 'NONE', #11061, #9394, #14917, .T. ) ;
#6102=VERTEX_POINT ( 'NONE', #14770 ) ;
#6103=AXIS2_PLACEMENT_3D ( 'NONE', #14451, #4057, #13304 ) ;
#6104=CARTESIAN_POINT ( 'NONE',  ( 68.58935777509475429, -68.58935777509547904, -8.000000000000000000 ) ) ;
#6105=ORIENTED_EDGE ( 'NONE', *, *, #1890, .T. ) ;
#6106=CARTESIAN_POINT ( 'NONE',  ( 0.000000000000000000, 0.000000000000000000, -10.50000000000000000 ) ) ;
#6107=EDGE_CURVE ( 'NONE', #14931, #9719, #1816, .T. ) ;
#6110=DIRECTION ( 'NONE',  ( 0.000000000000000000, 0.000000000000000000, -1.000000000000000000 ) ) ;
#6111=DIRECTION ( 'NONE',  ( 1.000000000000000000, 0.000000000000000000, 0.000000000000000000 ) ) ;
#6113=ORIENTED_EDGE ( 'NONE', *, *, #559, .T. ) ;
#6114=AXIS2_PLACEMENT_3D ( 'NONE', #7230, #8310, #7311 ) ;
#6116=CARTESIAN_POINT ( 'NONE',  ( 0.000000000000000000, 0.000000000000000000, -25.50000000000000355 ) ) ;
#6118=CARTESIAN_POINT ( 'NONE',  ( -45.89934640057513349, 26.50000000000019540, -10.50000000000000000 ) ) ;
#6120=ORIENTED_EDGE ( 'NONE', *, *, #8414, .T. ) ;
#6122=EDGE_LOOP ( 'NONE', ( #5727, #14745, #13789, #6073, #11543 ) ) ;
#6123=DIRECTION ( 'NONE',  ( -1.000000000000000000, 0.000000000000000000, 0.000000000000000000 ) ) ;
#6124=DIRECTION ( 'NONE',  ( -0.000000000000000000, -0.000000000000000000, 1.000000000000000000 ) ) ;
#6125=DIRECTION ( 'NONE',  ( 0.000000000000000000, 0.000000000000000000, 1.000000000000000000 ) ) ;
#6127=CARTESIAN_POINT ( 'NONE',  ( 56.43380494353997534, 12.86891638962136319, -8.000000000000000000 ) ) ;
#6128=CARTESIAN_POINT ( 'NONE',  ( -33.48561063518626923, 47.21331623427104063, 8.000000000000000000 ) ) ;
#6130=CARTESIAN_POINT ( 'NONE',  ( 0.000000000000000000, 0.000000000000000000, 10.50000000000000000 ) ) ;
#6131=AXIS2_PLACEMENT_3D ( 'NONE', #9670, #14401, #2713 ) ;
#6132=EDGE_LOOP ( 'NONE', ( #5729, #8329, #951, #2668, #5696 ) ) ;
#6133=ORIENTED_EDGE ( 'NONE', *, *, #7648, .F. ) ;
#6134=DIRECTION ( 'NONE',  ( 0.000000000000000000, 0.000000000000000000, -1.000000000000000000 ) ) ;
#6135=ORIENTED_EDGE ( 'NONE', *, *, #13259, .T. ) ;
#6137=CYLINDRICAL_SURFACE ( 'NONE', #14169, 0.5000000000000004441 ) ;
#6138=VERTEX_POINT ( 'NONE', #7923 ) ;
#6139=DIRECTION ( 'NONE',  ( 1.000000000000000000, 0.000000000000000000, 0.000000000000000000 ) ) ;
#6142=DIRECTION ( 'NONE',  ( 0.000000000000000000, 0.000000000000000000, 1.000000000000000000 ) ) ;
#6143=FACE_OUTER_BOUND ( 'NONE', #3431, .T. ) ;
#6144=ORIENTED_EDGE ( 'NONE', *, *, #1944, .T. ) ;
#6145=AXIS2_PLACEMENT_3D ( 'NONE', #13391, #4439, #12265 ) ;
#6147=AXIS2_PLACEMENT_3D ( 'NONE', #9858, #4101, #8569 ) ;
#6148=CARTESIAN_POINT ( 'NONE',  ( 68.58935777509523746, 68.58935777509499587, -13.00000000000000178 ) ) ;
#6150=EDGE_LOOP ( 'NONE', ( #568, #6349, #9056, #12004, #13815, #2484, #3704, #12411 ) ) ;
#6151=EDGE_CURVE ( 'NONE', #13119, #2051, #7144, .T. ) ;
#6152=ADVANCED_FACE ( 'NONE', ( #5351 ), #1862, .F. ) ;
#6153=ADVANCED_FACE ( 'NONE', ( #8834 ), #13476, .F. ) ;
#6155=CARTESIAN_POINT ( 'NONE',  ( -41.54772703543551415, -32.26435573746212526, 10.49999999999999822 ) ) ;
#6156=DIRECTION ( 'NONE',  ( 1.000000000000000000, 0.000000000000000000, -0.000000000000000000 ) ) ;
#6160=CIRCLE ( 'NONE', #14667, 60.50000000000000000 ) ;
#6163=ORIENTED_EDGE ( 'NONE', *, *, #619, .F. ) ;
#6165=LINE ( 'NONE', #14294, #4669 ) ;
#6166=CARTESIAN_POINT ( 'NONE',  ( -68.01302780753309207, 65.64523757230344359, -13.00000000000000178 ) ) ;
#6170=ORIENTED_EDGE ( 'NONE', *, *, #7648, .T. ) ;
#6171=VECTOR ( 'NONE', #14936, 1000.000000000000000 ) ;
#6172=DIRECTION ( 'NONE',  ( 0.000000000000000000, 0.000000000000000000, -1.000000000000000000 ) ) ;
#6180=VERTEX_POINT ( 'NONE', #12938 ) ;
#6186=CARTESIAN_POINT ( 'NONE',  ( 32.26435573746228158, -42.04772703543541468, -13.00000000000000178 ) ) ;
#6187=ORIENTED_EDGE ( 'NONE', *, *, #6107, .T. ) ;
#6188=LINE ( 'NONE', #4997, #3020 ) ;
#6189=DIRECTION ( 'NONE',  ( 1.000000000000000000, 0.000000000000000000, 0.000000000000000000 ) ) ;
#6193=EDGE_CURVE ( 'NONE', #7026, #14497, #13713, .T. ) ;
#6194=ADVANCED_FACE ( 'NONE', ( #3369 ), #9139, .T. ) ;
#6195=VERTEX_POINT ( 'NONE', #10503 ) ;
#6196=DIRECTION ( 'NONE',  ( 1.000000000000000000, 0.000000000000000000, 0.000000000000000000 ) ) ;
#6197=ORIENTED_EDGE ( 'NONE', *, *, #12432, .F. ) ;
#6199=AXIS2_PLACEMENT_3D ( 'NONE', #14378, #3985, #8600 ) ;
#6200=DIRECTION ( 'NONE',  ( -0.000000000000000000, -0.000000000000000000, 1.000000000000000000 ) ) ;
#6202=EDGE_CURVE ( 'NONE', #11991, #7285, #486, .T. ) ;
#6203=ORIENTED_EDGE ( 'NONE', *, *, #1164, .F. ) ;
#6204=CARTESIAN_POINT ( 'NONE',  ( 12.94095225512611869, -48.29629131445339851, 8.000000000000000000 ) ) ;
#6205=CARTESIAN_POINT ( 'NONE',  ( 1.674280531759324342, 99.48933418828643482, 8.000000000000000000 ) ) ;
#6206=ORIENTED_EDGE ( 'NONE', *, *, #13962, .T. ) ;
#6207=DIRECTION ( 'NONE',  ( 1.000000000000000000, 0.000000000000000000, 0.000000000000000000 ) ) ;
#6208=CIRCLE ( 'NONE', #5258, 3.000000000000002665 ) ;
#6211=ORIENTED_EDGE ( 'NONE', *, *, #8437, .F. ) ;
#6212=DIRECTION ( 'NONE',  ( 0.000000000000000000, 0.000000000000000000, 1.000000000000000000 ) ) ;
#6213=DIRECTION ( 'NONE',  ( -1.000000000000000000, 0.000000000000000000, 0.000000000000000000 ) ) ;
#6216=DIRECTION ( 'NONE',  ( 1.000000000000000000, 0.000000000000000000, 0.000000000000000000 ) ) ;
#6217=CARTESIAN_POINT ( 'NONE',  ( -53.26842454702436669, -11.55014193876159645, -8.000000000000000000 ) ) ;
#6218=ORIENTED_EDGE ( 'NONE', *, *, #4652, .T. ) ;
#6219=EDGE_LOOP ( 'NONE', ( #7937, #14520, #3359, #1904, #1295, #7931 ) ) ;
#6221=DIRECTION ( 'NONE',  ( -0.000000000000000000, -0.000000000000000000, 1.000000000000000000 ) ) ;
#6222=ORIENTED_EDGE ( 'NONE', *, *, #619, .T. ) ;
#6223=DIRECTION ( 'NONE',  ( -0.000000000000000000, -0.000000000000000000, 1.000000000000000000 ) ) ;
#6224=ORIENTED_EDGE ( 'NONE', *, *, #5312, .T. ) ;
#6225=DIRECTION ( 'NONE',  ( -0.000000000000000000, -0.000000000000000000, 1.000000000000000000 ) ) ;
#6226=ORIENTED_EDGE ( 'NONE', *, *, #7724, .T. ) ;
#6228=EDGE_LOOP ( 'NONE', ( #6678, #3740, #4597, #7694, #12186, #9214, #10672, #5641, #6120, #5407 ) ) ;
#6235=FACE_OUTER_BOUND ( 'NONE', #7787, .T. ) ;
#6236=ORIENTED_EDGE ( 'NONE', *, *, #125, .T. ) ;
#6237=FACE_OUTER_BOUND ( 'NONE', #3467, .T. ) ;
#6238=ADVANCED_FACE ( 'NONE', ( #10356 ), #7071, .T. ) ;
#6239=DIRECTION ( 'NONE',  ( 1.000000000000000000, 0.000000000000000000, 0.000000000000000000 ) ) ;
#6241=EDGE_LOOP ( 'NONE', ( #5437, #6630, #327, #4299 ) ) ;
#6245=CARTESIAN_POINT ( 'NONE',  ( -92.38795325112907619, -38.26834323650804492, -8.000000000000000000 ) ) ;
#6246=ADVANCED_FACE ( 'NONE', ( #9210 ), #2238, .T. ) ;
#6247=DIRECTION ( 'NONE',  ( 0.000000000000000000, 0.000000000000000000, 1.000000000000000000 ) ) ;
#6250=DIRECTION ( 'NONE',  ( 1.000000000000000000, 0.000000000000000000, 0.000000000000000000 ) ) ;
#6251=AXIS2_PLACEMENT_3D ( 'NONE', #2205, #11627, #1000 ) ;
#6253=DIRECTION ( 'NONE',  ( -1.000000000000000000, 0.000000000000000000, 0.000000000000000000 ) ) ;
#6254=DIRECTION ( 'NONE',  ( -0.000000000000000000, -0.000000000000000000, -1.000000000000000000 ) ) ;
#6256=ORIENTED_EDGE ( 'NONE', *, *, #3345, .T. ) ;
#6257=ORIENTED_EDGE ( 'NONE', *, *, #3663, .T. ) ;
#6259=EDGE_LOOP ( 'NONE', ( #14986, #14402, #3865, #2699 ) ) ;
#6260=FACE_OUTER_BOUND ( 'NONE', #6095, .T. ) ;
#6261=CARTESIAN_POINT ( 'NONE',  ( -15.88467684210512942, 49.11971303961693280, -13.00000000000000178 ) ) ;
#6263=EDGE_CURVE ( 'NONE', #2119, #1055, #14305, .T. ) ;
#6264=ORIENTED_EDGE ( 'NONE', *, *, #8414, .F. ) ;
#6265=VERTEX_POINT ( 'NONE', #11516 ) ;
#6266=DIRECTION ( 'NONE',  ( 1.000000000000000000, 0.000000000000000000, 0.000000000000000000 ) ) ;
#6268=EDGE_CURVE ( 'NONE', #197, #12197, #5092, .T. ) ;
#6270=DIRECTION ( 'NONE',  ( 1.000000000000000000, 0.000000000000000000, 0.000000000000000000 ) ) ;
#6271=ORIENTED_EDGE ( 'NONE', *, *, #1752, .F. ) ;
#6272=ORIENTED_EDGE ( 'NONE', *, *, #10515, .T. ) ;
#6274=EDGE_CURVE ( 'NONE', #8032, #1839, #12622, .T. ) ;
#6277=CARTESIAN_POINT ( 'NONE',  ( -13.21740939043329099, 51.19406879332069593, -13.00000000000000178 ) ) ;
#6278=CARTESIAN_POINT ( 'NONE',  ( -26.49999999999971578, -45.89934640057541060, -10.50000000000000000 ) ) ;
#6280=AXIS2_PLACEMENT_3D ( 'NONE', #5458, #5233, #680 ) ;
#6281=DIRECTION ( 'NONE',  ( 0.000000000000000000, 0.000000000000000000, 1.000000000000000000 ) ) ;
#6283=VERTEX_POINT ( 'NONE', #5037 ) ;
#6284=AXIS2_PLACEMENT_3D ( 'NONE', #7994, #11592, #6930 ) ;
#6285=CYLINDRICAL_SURFACE ( 'NONE', #13848, 56.99999999999999289 ) ;
#6286=ORIENTED_EDGE ( 'NONE', *, *, #14274, .F. ) ;
#6287=LINE ( 'NONE', #11097, #14234 ) ;
#6288=LINE ( 'NONE', #464, #14139 ) ;
#6289=ORIENTED_EDGE ( 'NONE', *, *, #8284, .T. ) ;
#6290=CARTESIAN_POINT ( 'NONE',  ( -32.26435573746199736, 42.04772703543562073, 8.000000000000000000 ) ) ;
#6291=CIRCLE ( 'NONE', #9690, 3.000000000000002665 ) ;
#6293=ORIENTED_EDGE ( 'NONE', *, *, #5967, .F. ) ;
#6294=DIRECTION ( 'NONE',  ( 0.000000000000000000, 0.000000000000000000, 1.000000000000000000 ) ) ;
#6295=AXIS2_PLACEMENT_3D ( 'NONE', #10784, #229, #12919 ) ;
#6296=ORIENTED_EDGE ( 'NONE', *, *, #3604, .F. ) ;
#6298=DIRECTION ( 'NONE',  ( 0.000000000000000000, 0.000000000000000000, 1.000000000000000000 ) ) ;
#6301=CARTESIAN_POINT ( 'NONE',  ( 53.63365512954693770, -9.714003807513686084, -8.000000000000000000 ) ) ;
#6302=DIRECTION ( 'NONE',  ( -1.000000000000000000, 0.000000000000000000, 0.000000000000000000 ) ) ;
#6305=FACE_OUTER_BOUND ( 'NONE', #12311, .T. ) ;
#6307=CYLINDRICAL_SURFACE ( 'NONE', #11765, 3.000000000000002665 ) ;
#6311=EDGE_LOOP ( 'NONE', ( #10914, #7549, #8455, #4624 ) ) ;
#6313=ORIENTED_EDGE ( 'NONE', *, *, #2179, .F. ) ;
#6314=CARTESIAN_POINT ( 'NONE',  ( 0.000000000000000000, 0.000000000000000000, -10.50000000000000000 ) ) ;
#6315=EDGE_LOOP ( 'NONE', ( #6935, #802, #8505, #7360 ) ) ;
#6317=CARTESIAN_POINT ( 'NONE',  ( 1.674280531759324342, 99.48933418828643482, -8.000000000000000000 ) ) ;
#6319=FACE_OUTER_BOUND ( 'NONE', #6219, .T. ) ;
#6320=DIRECTION ( 'NONE',  ( 0.000000000000000000, 0.000000000000000000, 1.000000000000000000 ) ) ;
#6322=CARTESIAN_POINT ( 'NONE',  ( 0.000000000000000000, 0.000000000000000000, -10.50000000000000000 ) ) ;
#6323=VERTEX_POINT ( 'NONE', #3976 ) ;
#6326=DIRECTION ( 'NONE',  ( 0.000000000000000000, 0.000000000000000000, 1.000000000000000000 ) ) ;
#6328=EDGE_CURVE ( 'NONE', #9063, #11311, #9450, .T. ) ;
#6329=CYLINDRICAL_SURFACE ( 'NONE', #3244, 63.00000000000000000 ) ;
#6330=ADVANCED_FACE ( 'NONE', ( #8520 ), #9644, .F. ) ;
#6331=ADVANCED_FACE ( 'NONE', ( #13087 ), #1547, .F. ) ;
#6332=ORIENTED_EDGE ( 'NONE', *, *, #1110, .T. ) ;
#6333=AXIS2_PLACEMENT_3D ( 'NONE', #656, #9980, #11352 ) ;
#6334=VERTEX_POINT ( 'NONE', #12035 ) ;
#6335=DIRECTION ( 'NONE',  ( -1.000000000000000000, 0.000000000000000000, 0.000000000000000000 ) ) ;
#6337=ORIENTED_EDGE ( 'NONE', *, *, #5913, .F. ) ;
#6339=AXIS2_PLACEMENT_3D ( 'NONE', #12428, #7856, #14481 ) ;
#6340=DIRECTION ( 'NONE',  ( 0.000000000000000000, 0.000000000000000000, 1.000000000000000000 ) ) ;
#6341=CARTESIAN_POINT ( 'NONE',  ( 6.526309611002977462, 49.57224306869046870, -8.000000000000000000 ) ) ;
#6343=VECTOR ( 'NONE', #637, 1000.000000000000000 ) ;
#6347=CIRCLE ( 'NONE', #4757, 60.50000000000000000 ) ;
#6348=CIRCLE ( 'NONE', #2488, 0.5000000000000004441 ) ;
#6349=ORIENTED_EDGE ( 'NONE', *, *, #9257, .T. ) ;
#6350=FACE_OUTER_BOUND ( 'NONE', #7756, .T. ) ;
#6351=ADVANCED_FACE ( 'NONE', ( #14293 ), #9802, .T. ) ;
#6353=CIRCLE ( 'NONE', #14875, 2.649999999999985700 ) ;
#6355=CARTESIAN_POINT ( 'NONE',  ( -49.00442420935969778, 30.80502811811250297, -10.50000000000000000 ) ) ;
#6356=CYLINDRICAL_SURFACE ( 'NONE', #9969, 50.00000000000000000 ) ;
#6357=DIRECTION ( 'NONE',  ( 0.000000000000000000, 0.000000000000000000, 1.000000000000000000 ) ) ;
#6360=ORIENTED_EDGE ( 'NONE', *, *, #9126, .T. ) ;
#6362=DIRECTION ( 'NONE',  ( 1.000000000000000000, 0.000000000000000000, 0.000000000000000000 ) ) ;
#6363=DIRECTION ( 'NONE',  ( 0.000000000000000000, 0.000000000000000000, 1.000000000000000000 ) ) ;
#6364=DIRECTION ( 'NONE',  ( 0.000000000000000000, 0.000000000000000000, 1.000000000000000000 ) ) ;
#6365=AXIS2_PLACEMENT_3D ( 'NONE', #8684, #13322, #11058 ) ;
#6366=EDGE_LOOP ( 'NONE', ( #5675, #989, #12701, #6503 ) ) ;
#6368=EDGE_LOOP ( 'NONE', ( #2724, #10694, #984, #8376, #12732, #2349, #2041, #11802, #13467 ) ) ;
#6369=EDGE_CURVE ( 'NONE', #1906, #8030, #7378, .T. ) ;
#6370=FACE_BOUND ( 'NONE', #4277, .T. ) ;
#6372=EDGE_CURVE ( 'NONE', #14250, #14615, #14229, .T. ) ;
#6373=ORIENTED_EDGE ( 'NONE', *, *, #11619, .T. ) ;
#6374=CARTESIAN_POINT ( 'NONE',  ( -51.45950017607691507, 4.121772567811807342, -8.000000000000000000 ) ) ;
#6376=CARTESIAN_POINT ( 'NONE',  ( 0.000000000000000000, 0.000000000000000000, 13.00000000000000178 ) ) ;
#6377=CARTESIAN_POINT ( 'NONE',  ( -51.53979475227126983, -13.35619814848815601, 10.49999999999999822 ) ) ;
#6378=CYLINDRICAL_SURFACE ( 'NONE', #2734, 100.0000000000000000 ) ;
#6379=CIRCLE ( 'NONE', #14893, 59.50000000000000000 ) ;
#6380=VECTOR ( 'NONE', #10067, 1000.000000000000000 ) ;
#6383=DIRECTION ( 'NONE',  ( 0.000000000000000000, 0.000000000000000000, 1.000000000000000000 ) ) ;
#6384=EDGE_CURVE ( 'NONE', #11004, #1282, #4381, .T. ) ;
#6385=CARTESIAN_POINT ( 'NONE',  ( -37.21932736666205699, 89.12622059913296368, 10.49999999999999822 ) ) ;
#6386=EDGE_LOOP ( 'NONE', ( #12300, #6360, #5020, #7840, #4817, #5397, #9607, #1668, #12715 ) ) ;
#6391=AXIS2_PLACEMENT_3D ( 'NONE', #10231, #1278, #12814 ) ;
#6395=ORIENTED_EDGE ( 'NONE', *, *, #8159, .T. ) ;
#6397=CARTESIAN_POINT ( 'NONE',  ( -36.52608637591512775, 92.55687898036946137, -13.00000000000000178 ) ) ;
#6399=AXIS2_PLACEMENT_3D ( 'NONE', #6988, #8069, #14992 ) ;
#6400=PLANE ( 'NONE',  #1239 ) ;
#6403=ORIENTED_EDGE ( 'NONE', *, *, #8969, .T. ) ;
#6404=AXIS2_PLACEMENT_3D ( 'NONE', #572, #11055, #12113 ) ;
#6405=AXIS2_PLACEMENT_3D ( 'NONE', #9652, #339, #8385 ) ;
#6406=AXIS2_PLACEMENT_3D ( 'NONE', #9701, #12154, #311 ) ;
#6408=VERTEX_POINT ( 'NONE', #8377 ) ;
#6409=LINE ( 'NONE', #5363, #5477 ) ;
#6410=FACE_OUTER_BOUND ( 'NONE', #14923, .T. ) ;
#6411=DIRECTION ( 'NONE',  ( 0.000000000000000000, 0.000000000000000000, 1.000000000000000000 ) ) ;
#6412=ORIENTED_EDGE ( 'NONE', *, *, #10049, .F. ) ;
#6413=ORIENTED_EDGE ( 'NONE', *, *, #2159, .F. ) ;
#6414=CIRCLE ( 'NONE', #14200, 100.0000000000000000 ) ;
#6415=VERTEX_POINT ( 'NONE', #8666 ) ;
#6416=CARTESIAN_POINT ( 'NONE',  ( -68.58935777509570642, -68.58935777509452691, 8.000000000000000000 ) ) ;
#6418=CARTESIAN_POINT ( 'NONE',  ( -65.58935777509570642, -68.58935777509452691, -13.00000000000000178 ) ) ;
#6420=EDGE_CURVE ( 'NONE', #12891, #9888, #8003, .T. ) ;
#6421=CARTESIAN_POINT ( 'NONE',  ( 0.000000000000000000, 0.000000000000000000, 10.50000000000000000 ) ) ;
#6422=CIRCLE ( 'NONE', #14938, 3.000000000000002665 ) ;
#6424=ORIENTED_EDGE ( 'NONE', *, *, #12806, .T. ) ;
#6426=DIRECTION ( 'NONE',  ( 0.000000000000000000, 0.000000000000000000, -1.000000000000000000 ) ) ;
#6427=DIRECTION ( 'NONE',  ( 0.000000000000000000, 0.000000000000000000, 1.000000000000000000 ) ) ;
#6428=ORIENTED_EDGE ( 'NONE', *, *, #6384, .F. ) ;
#6429=ADVANCED_FACE ( 'NONE', ( #10871 ), #1402, .T. ) ;
#6431=VERTEX_POINT ( 'NONE', #14150 ) ;
#6432=VERTEX_POINT ( 'NONE', #13015 ) ;
#6434=CIRCLE ( 'NONE', #9357, 0.5000000000000004441 ) ;
#6435=ADVANCED_FACE ( 'NONE', ( #11874 ), #13683, .F. ) ;
#6436=DIRECTION ( 'NONE',  ( -0.000000000000000000, -0.000000000000000000, 1.000000000000000000 ) ) ;
#6437=CARTESIAN_POINT ( 'NONE',  ( 0.000000000000000000, 0.000000000000000000, -8.000000000000000000 ) ) ;
#6438=LINE ( 'NONE', #12231, #8967 ) ;
#6439=ADVANCED_FACE ( 'NONE', ( #7519 ), #14685, .F. ) ;
#6442=VECTOR ( 'NONE', #1314, 1000.000000000000000 ) ;
#6443=CARTESIAN_POINT ( 'NONE',  ( -37.12029293941441210, -89.61631465359452875, 8.000000000000000000 ) ) ;
#6446=DIRECTION ( 'NONE',  ( 0.000000000000000000, 0.000000000000000000, 1.000000000000000000 ) ) ;
#6447=DIRECTION ( 'NONE',  ( 1.000000000000000000, 0.000000000000000000, -0.000000000000000000 ) ) ;
#6448=ORIENTED_EDGE ( 'NONE', *, *, #5913, .T. ) ;
#6449=SURFACE_STYLE_USAGE ( .BOTH. , #1836 ) ;
#6450=AXIS2_PLACEMENT_3D ( 'NONE', #751, #8783, #7796 ) ;
#6451=VERTEX_POINT ( 'NONE', #4351 ) ;
#6453=ORIENTED_EDGE ( 'NONE', *, *, #2576, .F. ) ;
#6454=CIRCLE ( 'NONE', #14969, 0.5000000000000004441 ) ;
#6455=CARTESIAN_POINT ( 'NONE',  ( -69.08004447556112382, -68.68541276968802833, -13.00000000000000178 ) ) ;
#6457=DIRECTION ( 'NONE',  ( 1.000000000000000000, 0.000000000000000000, -0.000000000000000000 ) ) ;
#6458=DIRECTION ( 'NONE',  ( 0.000000000000000000, 0.000000000000000000, 1.000000000000000000 ) ) ;
#6459=CARTESIAN_POINT ( 'NONE',  ( -46.33974596215558961, 0.000000000000000000, -28.00000000000000000 ) ) ;
#6460=DIRECTION ( 'NONE',  ( 0.000000000000000000, 0.000000000000000000, 1.000000000000000000 ) ) ;
#6461=CARTESIAN_POINT ( 'NONE',  ( 6.917888187663118416, 52.54657765281190507, 8.000000000000000000 ) ) ;
#6462=EDGE_CURVE ( 'NONE', #9943, #5837, #9681, .T. ) ;
#6463=VERTEX_POINT ( 'NONE', #9878 ) ;
#6464=EDGE_CURVE ( 'NONE', #10294, #8906, #6778, .T. ) ;
#6465=CARTESIAN_POINT ( 'NONE',  ( -89.61631465359441506, 37.12029293941468211, -13.00000000000000178 ) ) ;
#6466=CARTESIAN_POINT ( 'NONE',  ( 65.64523757230274725, 68.01302780753375998, -8.000000000000000000 ) ) ;
#6467=EDGE_CURVE ( 'NONE', #11040, #9943, #9206, .T. ) ;
#6468=ADVANCED_FACE ( 'NONE', ( #4207 ), #11258, .F. ) ;
#6470=ORIENTED_EDGE ( 'NONE', *, *, #4326, .F. ) ;
#6472=CYLINDRICAL_SURFACE ( 'NONE', #8277, 0.5000000000000004441 ) ;
#6473=ORIENTED_EDGE ( 'NONE', *, *, #4360, .T. ) ;
#6474=CARTESIAN_POINT ( 'NONE',  ( 33.48561063518626923, -47.21331623427104063, -13.00000000000000178 ) ) ;
#6476=DIRECTION ( 'NONE',  ( 0.000000000000000000, 0.000000000000000000, 1.000000000000000000 ) ) ;
#6477=DIRECTION ( 'NONE',  ( -0.000000000000000000, -0.000000000000000000, 1.000000000000000000 ) ) ;
#6479=ORIENTED_EDGE ( 'NONE', *, *, #14004, .T. ) ;
#6480=ORIENTED_EDGE ( 'NONE', *, *, #12023, .T. ) ;
#6481=EDGE_CURVE ( 'NONE', #11386, #3826, #866, .T. ) ;
#6482=DIRECTION ( 'NONE',  ( 0.000000000000000000, 0.000000000000000000, -1.000000000000000000 ) ) ;
#6484=CARTESIAN_POINT ( 'NONE',  ( 89.61631465359468507, -37.12029293941410657, 8.000000000000000000 ) ) ;
#6485=ORIENTED_EDGE ( 'NONE', *, *, #7532, .F. ) ;
#6486=AXIS2_PLACEMENT_3D ( 'NONE', #10602, #3482, #13966 ) ;
#6488=VERTEX_POINT ( 'NONE', #11107 ) ;
#6489=DIRECTION ( 'NONE',  ( -1.000000000000000000, 0.000000000000000000, 0.000000000000000000 ) ) ;
#6490=CARTESIAN_POINT ( 'NONE',  ( 0.000000000000000000, 0.000000000000000000, -8.000000000000000000 ) ) ;
#6492=VERTEX_POINT ( 'NONE', #939 ) ;
#6493=DIRECTION ( 'NONE',  ( 0.000000000000000000, 0.000000000000000000, 1.000000000000000000 ) ) ;
#6495=VERTEX_POINT ( 'NONE', #5488 ) ;
#6497=VERTEX_POINT ( 'NONE', #6377 ) ;
#6499=ORIENTED_EDGE ( 'NONE', *, *, #5409, .F. ) ;
#6500=DIRECTION ( 'NONE',  ( -1.000000000000000000, 0.000000000000000000, 0.000000000000000000 ) ) ;
#6502=EDGE_CURVE ( 'NONE', #8412, #13856, #11889, .T. ) ;
#6503=ORIENTED_EDGE ( 'NONE', *, *, #8373, .F. ) ;
#6504=DIRECTION ( 'NONE',  ( 0.000000000000000000, 0.000000000000000000, 1.000000000000000000 ) ) ;
#6505=AXIS2_PLACEMENT_3D ( 'NONE', #1163, #13994, #12841 ) ;
#6507=CARTESIAN_POINT ( 'NONE',  ( -39.30189486418265687, -33.47282819776598473, -13.00000000000000178 ) ) ;
#6509=VERTEX_POINT ( 'NONE', #706 ) ;
#6510=CYLINDRICAL_SURFACE ( 'NONE', #9259, 60.50000000000000000 ) ;
#6511=EDGE_CURVE ( 'NONE', #10004, #14269, #10682, .T. ) ;
#6513=AXIS2_PLACEMENT_3D ( 'NONE', #8419, #12003, #10844 ) ;
#6515=VERTEX_POINT ( 'NONE', #13527 ) ;
#6518=ADVANCED_FACE ( 'NONE', ( #2982 ), #7604, .F. ) ;
#6521=ORIENTED_EDGE ( 'NONE', *, *, #13254, .T. ) ;
#6522=LINE ( 'NONE', #2136, #2185 ) ;
#6526=DIRECTION ( 'NONE',  ( 0.000000000000000000, 0.000000000000000000, -1.000000000000000000 ) ) ;
#6527=CARTESIAN_POINT ( 'NONE',  ( 0.000000000000000000, 0.000000000000000000, 10.50000000000000000 ) ) ;
#6529=AXIS2_PLACEMENT_3D ( 'NONE', #2836, #13303, #473 ) ;
#6530=DIRECTION ( 'NONE',  ( 0.000000000000000000, 0.000000000000000000, 1.000000000000000000 ) ) ;
#6531=CIRCLE ( 'NONE', #7991, 3.000000000000002665 ) ;
#6532=CARTESIAN_POINT ( 'NONE',  ( -6.917888187662729393, -52.54657765281195481, -10.50000000000000000 ) ) ;
#6534=DIRECTION ( 'NONE',  ( 1.000000000000000000, 0.000000000000000000, 0.000000000000000000 ) ) ;
#6538=AXIS2_PLACEMENT_3D ( 'NONE', #7679, #3207, #10262 ) ;
#6540=ORIENTED_EDGE ( 'NONE', *, *, #9620, .T. ) ;
#6541=DIRECTION ( 'NONE',  ( 0.000000000000000000, 0.000000000000000000, -1.000000000000000000 ) ) ;
#6542=EDGE_LOOP ( 'NONE', ( #9046, #5304, #13728, #9199, #2893 ) ) ;
#6543=EDGE_CURVE ( 'NONE', #6775, #2732, #10921, .T. ) ;
#6544=DIRECTION ( 'NONE',  ( -0.000000000000000000, -0.000000000000000000, 1.000000000000000000 ) ) ;
#6545=DIRECTION ( 'NONE',  ( 1.000000000000000000, 0.000000000000000000, 0.000000000000000000 ) ) ;
#6546=AXIS2_PLACEMENT_3D ( 'NONE', #5008, #3861, #14331 ) ;
#6547=EDGE_CURVE ( 'NONE', #11546, #1207, #13586, .T. ) ;
#6548=DIRECTION ( 'NONE',  ( 0.000000000000000000, 0.000000000000000000, 1.000000000000000000 ) ) ;
#6549=CARTESIAN_POINT ( 'NONE',  ( -52.04657765281192638, 6.917888187662934563, -10.50000000000000000 ) ) ;
#6551=VERTEX_POINT ( 'NONE', #5627 ) ;
#6554=EDGE_LOOP ( 'NONE', ( #11534, #9356, #7322, #9108, #10154, #7526, #7007, #9419, #3079, #12109 ) ) ;
#6555=ORIENTED_EDGE ( 'NONE', *, *, #5772, .T. ) ;
#6556=AXIS2_PLACEMENT_3D ( 'NONE', #7716, #6573, #8865 ) ;
#6557=ADVANCED_FACE ( 'NONE', ( #8 ), #85, .F. ) ;
#6560=DIRECTION ( 'NONE',  ( 0.000000000000000000, 0.000000000000000000, 1.000000000000000000 ) ) ;
#6561=VERTEX_POINT ( 'NONE', #9341 ) ;
#6562=AXIS2_PLACEMENT_3D ( 'NONE', #14647, #12296, #7568 ) ;
#6563=ORIENTED_EDGE ( 'NONE', *, *, #13638, .T. ) ;
#6565=EDGE_CURVE ( 'NONE', #11838, #3039, #4152, .T. ) ;
#6567=EDGE_CURVE ( 'NONE', #6561, #7296, #4391, .T. ) ;
#6568=CIRCLE ( 'NONE', #4418, 0.5000000000000004441 ) ;
#6570=CYLINDRICAL_SURFACE ( 'NONE', #4697, 2.649999999999992806 ) ;
#6572=ORIENTED_EDGE ( 'NONE', *, *, #4069, .T. ) ;
#6573=DIRECTION ( 'NONE',  ( 0.000000000000000000, 0.000000000000000000, 1.000000000000000000 ) ) ;
#6578=DIRECTION ( 'NONE',  ( 0.000000000000000000, 0.000000000000000000, 1.000000000000000000 ) ) ;
#6579=AXIS2_PLACEMENT_3D ( 'NONE', #11769, #3717, #13320 ) ;
#6580=ORIENTED_EDGE ( 'NONE', *, *, #11918, .T. ) ;
#6581=ORIENTED_EDGE ( 'NONE', *, *, #14792, .T. ) ;
#6582=CARTESIAN_POINT ( 'NONE',  ( -45.89934640057513349, 26.50000000000019540, -13.00000000000000178 ) ) ;
#6583=DIRECTION ( 'NONE',  ( 1.000000000000000000, 0.000000000000000000, 0.000000000000000000 ) ) ;
#6584=CIRCLE ( 'NONE', #9739, 50.00000000000000000 ) ;
#6585=CARTESIAN_POINT ( 'NONE',  ( 94.51066581171355097, 1.674280531758986834, -8.000000000000000000 ) ) ;
#6586=CARTESIAN_POINT ( 'NONE',  ( 0.000000000000000000, 0.000000000000000000, -10.50000000000000000 ) ) ;
#6588=ORIENTED_EDGE ( 'NONE', *, *, #11370, .F. ) ;
#6589=DIRECTION ( 'NONE',  ( 0.000000000000000000, 0.000000000000000000, 1.000000000000000000 ) ) ;
#6590=CIRCLE ( 'NONE', #12436, 3.000000000000004441 ) ;
#6591=CARTESIAN_POINT ( 'NONE',  ( -14.07862063237857342, 50.84834283437004387, -13.00000000000000178 ) ) ;
#6592=CARTESIAN_POINT ( 'NONE',  ( -3.492805317593278058, 46.55633131742322917, -10.50000000000000000 ) ) ;
#6594=VERTEX_POINT ( 'NONE', #3438 ) ;
#6596=ORIENTED_EDGE ( 'NONE', *, *, #2830, .F. ) ;
#6597=VECTOR ( 'NONE', #14167, 1000.000000000000000 ) ;
#6600=DIRECTION ( 'NONE',  ( 0.000000000000000000, 0.000000000000000000, 1.000000000000000000 ) ) ;
#6604=CARTESIAN_POINT ( 'NONE',  ( 87.95718916809192933, -34.62083247296232713, -13.00000000000000178 ) ) ;
#6605=FACE_OUTER_BOUND ( 'NONE', #12330, .T. ) ;
#6606=VECTOR ( 'NONE', #2747, 1000.000000000000000 ) ;
#6609=EDGE_CURVE ( 'NONE', #2014, #9738, #4626, .T. ) ;
#6610=DIRECTION ( 'NONE',  ( 1.000000000000000000, 0.000000000000000000, 0.000000000000000000 ) ) ;
#6611=EDGE_CURVE ( 'NONE', #5951, #964, #14979, .T. ) ;
#6612=EDGE_CURVE ( 'NONE', #836, #3842, #12630, .T. ) ;
#6616=CARTESIAN_POINT ( 'NONE',  ( 68.49330278050122445, -68.09867107463004743, -13.00000000000000178 ) ) ;
#6617=CARTESIAN_POINT ( 'NONE',  ( -52.54657765281192638, 6.917888187662934563, -13.00000000000000178 ) ) ;
#6619=FACE_OUTER_BOUND ( 'NONE', #782, .T. ) ;
#6621=EDGE_LOOP ( 'NONE', ( #3088, #5302, #14385, #9902 ) ) ;
#6624=ORIENTED_EDGE ( 'NONE', *, *, #8286, .T. ) ;
#6625=CARTESIAN_POINT ( 'NONE',  ( 9.706953719245472456, 57.06275842387054098, -13.00000000000000178 ) ) ;
#6626=DIRECTION ( 'NONE',  ( 0.000000000000000000, 0.000000000000000000, -1.000000000000000000 ) ) ;
#6627=DIRECTION ( 'NONE',  ( -0.000000000000000000, -0.000000000000000000, 1.000000000000000000 ) ) ;
#6628=DIRECTION ( 'NONE',  ( 1.000000000000000000, 0.000000000000000000, 0.000000000000000000 ) ) ;
#6630=ORIENTED_EDGE ( 'NONE', *, *, #10346, .T. ) ;
#6631=VERTEX_POINT ( 'NONE', #2221 ) ;
#6632=EDGE_LOOP ( 'NONE', ( #3744, #2449, #160, #2583 ) ) ;
#6633=AXIS2_PLACEMENT_3D ( 'NONE', #9951, #13376, #4049 ) ;
#6634=VECTOR ( 'NONE', #6340, 1000.000000000000000 ) ;
#6635=CARTESIAN_POINT ( 'NONE',  ( 68.58935777509523746, 68.58935777509499587, -10.50000000000000000 ) ) ;
#6637=CIRCLE ( 'NONE', #1082, 60.50000000000000000 ) ;
#6639=CARTESIAN_POINT ( 'NONE',  ( 41.94820822869167642, 33.29654390035863543, -10.50000000000000000 ) ) ;
#6640=ORIENTED_EDGE ( 'NONE', *, *, #8025, .F. ) ;
#6641=ORIENTED_EDGE ( 'NONE', *, *, #2437, .F. ) ;
#6642=CIRCLE ( 'NONE', #2302, 60.50000000000000000 ) ;
#6646=CIRCLE ( 'NONE', #10776, 2.649999999999992806 ) ;
#6647=DIRECTION ( 'NONE',  ( 0.000000000000000000, 0.000000000000000000, 1.000000000000000000 ) ) ;
#6648=DIRECTION ( 'NONE',  ( 0.000000000000000000, 0.000000000000000000, 1.000000000000000000 ) ) ;
#6650=ORIENTED_EDGE ( 'NONE', *, *, #83, .T. ) ;
#6651=CARTESIAN_POINT ( 'NONE',  ( 53.55662432702593634, -6.558794855522958910E-15, -10.50000000000000000 ) ) ;
#6652=CARTESIAN_POINT ( 'NONE',  ( 19.68583958711425552, -30.74264578624780597, -25.50000000000000355 ) ) ;
#6657=EDGE_CURVE ( 'NONE', #4183, #13408, #12864, .T. ) ;
#6659=VERTEX_POINT ( 'NONE', #10485 ) ;
#6662=DIRECTION ( 'NONE',  ( 0.000000000000000000, 0.000000000000000000, -1.000000000000000000 ) ) ;
#6663=CARTESIAN_POINT ( 'NONE',  ( -13.71740939043329277, 51.19406879332069593, 8.000000000000000000 ) ) ;
#6664=EDGE_CURVE ( 'NONE', #8869, #11469, #2200, .T. ) ;
#6666=AXIS2_PLACEMENT_3D ( 'NONE', #384, #6134, #5021 ) ;
#6670=CARTESIAN_POINT ( 'NONE',  ( 0.000000000000000000, 0.000000000000000000, -10.50000000000000000 ) ) ;
#6671=ORIENTED_EDGE ( 'NONE', *, *, #12649, .F. ) ;
#6673=EDGE_CURVE ( 'NONE', #13021, #2940, #6068, .T. ) ;
#6674=AXIS2_PLACEMENT_3D ( 'NONE', #2331, #13802, #13884 ) ;
#6678=ORIENTED_EDGE ( 'NONE', *, *, #9759, .T. ) ;
#6679=DIRECTION ( 'NONE',  ( 0.000000000000000000, 0.000000000000000000, -1.000000000000000000 ) ) ;
#6680=VERTEX_POINT ( 'NONE', #13068 ) ;
#6682=ORIENTED_EDGE ( 'NONE', *, *, #2631, .F. ) ;
#6683=DIRECTION ( 'NONE',  ( 0.000000000000000000, 0.000000000000000000, 1.000000000000000000 ) ) ;
#6685=DIRECTION ( 'NONE',  ( -1.000000000000000000, 0.000000000000000000, 0.000000000000000000 ) ) ;
#6686=CARTESIAN_POINT ( 'NONE',  ( 68.58935777509475429, -68.58935777509547904, 10.49999999999999822 ) ) ;
#6687=CIRCLE ( 'NONE', #8149, 3.000000000000002665 ) ;
#6688=CARTESIAN_POINT ( 'NONE',  ( -12.86891638962156215, 56.43380494353993271, 10.49999999999999822 ) ) ;
#6691=ORIENTED_EDGE ( 'NONE', *, *, #11166, .F. ) ;
#6693=DIRECTION ( 'NONE',  ( 0.000000000000000000, 0.000000000000000000, -1.000000000000000000 ) ) ;
#6695=CIRCLE ( 'NONE', #14720, 56.99999999999998579 ) ;
#6696=CYLINDRICAL_SURFACE ( 'NONE', #3524, 56.99999999999999289 ) ;
#6698=EDGE_CURVE ( 'NONE', #836, #4561, #1228, .T. ) ;
#6699=DIRECTION ( 'NONE',  ( 1.000000000000000000, 0.000000000000000000, 0.000000000000000000 ) ) ;
#6700=EDGE_CURVE ( 'NONE', #7016, #3633, #499, .T. ) ;
#6701=ORIENTED_EDGE ( 'NONE', *, *, #14248, .T. ) ;
#6703=DIRECTION ( 'NONE',  ( 0.000000000000000000, 0.000000000000000000, 1.000000000000000000 ) ) ;
#6704=ORIENTED_EDGE ( 'NONE', *, *, #458, .T. ) ;
#6709=ORIENTED_EDGE ( 'NONE', *, *, #6609, .F. ) ;
#6717=DIRECTION ( 'NONE',  ( -1.000000000000000000, 0.000000000000000000, 0.000000000000000000 ) ) ;
#6718=FACE_OUTER_BOUND ( 'NONE', #5541, .T. ) ;
#6719=CARTESIAN_POINT ( 'NONE',  ( 92.61631465359468507, -37.12029293941410657, -8.000000000000000000 ) ) ;
#6721=CARTESIAN_POINT ( 'NONE',  ( 12.86891638962116247, -56.43380494354001087, -13.00000000000000178 ) ) ;
#6722=PLANE ( 'NONE',  #2226 ) ;
#6724=DIRECTION ( 'NONE',  ( -0.000000000000000000, -0.000000000000000000, 1.000000000000000000 ) ) ;
#6727=ORIENTED_EDGE ( 'NONE', *, *, #7008, .F. ) ;
#6728=PLANE ( 'NONE',  #4513 ) ;
#6729=ORIENTED_EDGE ( 'NONE', *, *, #8145, .T. ) ;
#6731=ADVANCED_FACE ( 'NONE', ( #9702 ), #10856, .F. ) ;
#6732=DIRECTION ( 'NONE',  ( -0.000000000000000000, -0.000000000000000000, 1.000000000000000000 ) ) ;
#6733=ADVANCED_FACE ( 'NONE', ( #9630 ), #14131, .F. ) ;
#6735=LINE ( 'NONE', #11391, #9814 ) ;
#6736=FACE_OUTER_BOUND ( 'NONE', #6386, .T. ) ;
#6738=VERTEX_POINT ( 'NONE', #14350 ) ;
#6740=ORIENTED_EDGE ( 'NONE', *, *, #6900, .T. ) ;
#6741=EDGE_CURVE ( 'NONE', #8488, #13671, #8570, .T. ) ;
#6742=DIRECTION ( 'NONE',  ( 0.000000000000000000, 0.000000000000000000, 1.000000000000000000 ) ) ;
#6743=DIRECTION ( 'NONE',  ( -0.000000000000000000, -0.000000000000000000, -1.000000000000000000 ) ) ;
#6744=ORIENTED_EDGE ( 'NONE', *, *, #14274, .T. ) ;
#6747=FACE_OUTER_BOUND ( 'NONE', #2102, .T. ) ;
#6748=EDGE_CURVE ( 'NONE', #11386, #11838, #10194, .T. ) ;
#6749=ADVANCED_FACE ( 'NONE', ( #13145 ), #8431, .F. ) ;
#6750=CARTESIAN_POINT ( 'NONE',  ( -2.449293598294700991E-16, 97.00000000000000000, 8.000000000000000000 ) ) ;
#6753=DIRECTION ( 'NONE',  ( 0.000000000000000000, 0.000000000000000000, 1.000000000000000000 ) ) ;
#6755=AXIS2_PLACEMENT_3D ( 'NONE', #9705, #1530, #3959 ) ;
#6757=ORIENTED_EDGE ( 'NONE', *, *, #5000, .T. ) ;
#6758=CARTESIAN_POINT ( 'NONE',  ( 68.58935777509475429, -68.58935777509547904, 8.000000000000000000 ) ) ;
#6759=CARTESIAN_POINT ( 'NONE',  ( 68.01302780753354682, -65.64523757230297463, -8.000000000000000000 ) ) ;
#6760=CYLINDRICAL_SURFACE ( 'NONE', #9513, 3.000000000000002665 ) ;
#6761=AXIS2_PLACEMENT_3D ( 'NONE', #524, #12072, #9767 ) ;
#6763=EDGE_LOOP ( 'NONE', ( #13353, #12260, #2034, #4699 ) ) ;
#6765=CIRCLE ( 'NONE', #6513, 0.5000000000000004441 ) ;
#6767=AXIS2_PLACEMENT_3D ( 'NONE', #5166, #9934, #1895 ) ;
#6768=PLANE ( 'NONE',  #2538 ) ;
#6771=CARTESIAN_POINT ( 'NONE',  ( 12.86891638962116247, -56.43380494354001087, -13.00000000000000178 ) ) ;
#6774=AXIS2_PLACEMENT_3D ( 'NONE', #5768, #4725, #13989 ) ;
#6775=VERTEX_POINT ( 'NONE', #9484 ) ;
#6776=EDGE_CURVE ( 'NONE', #2714, #7044, #9461, .T. ) ;
#6777=CARTESIAN_POINT ( 'NONE',  ( 44.79355920668812274, 31.05588327715851449, 8.000000000000000000 ) ) ;
#6778=CIRCLE ( 'NONE', #987, 63.00000000000000000 ) ;
#6780=( GEOMETRIC_REPRESENTATION_CONTEXT ( 3 ) GLOBAL_UNCERTAINTY_ASSIGNED_CONTEXT ( ( #765 ) ) GLOBAL_UNIT_ASSIGNED_CONTEXT ( ( #9684, #8555, #9542 ) ) REPRESENTATION_CONTEXT ( 'NONE', 'WORKASPACE' ) );
#6781=CARTESIAN_POINT ( 'NONE',  ( -52.36539807335606156, 6.451868917687758831, 10.49999999999999822 ) ) ;
#6783=ORIENTED_EDGE ( 'NONE', *, *, #5907, .F. ) ;
#6785=ORIENTED_EDGE ( 'NONE', *, *, #7198, .T. ) ;
#6788=AXIS2_PLACEMENT_3D ( 'NONE', #5331, #9958, #14607 ) ;
#6789=DIRECTION ( 'NONE',  ( -0.000000000000000000, -0.000000000000000000, -1.000000000000000000 ) ) ;
#6790=AXIS2_PLACEMENT_3D ( 'NONE', #6592, #6364, #6447 ) ;
#6794=CARTESIAN_POINT ( 'NONE',  ( 89.61631465359468507, -37.12029293941410657, 8.000000000000000000 ) ) ;
#6795=ORIENTED_EDGE ( 'NONE', *, *, #4726, .F. ) ;
#6796=FACE_OUTER_BOUND ( 'NONE', #11905, .T. ) ;
#6799=EDGE_CURVE ( 'NONE', #1338, #11078, #5105, .T. ) ;
#6801=CIRCLE ( 'NONE', #11434, 56.99999999999999289 ) ;
#6803=CARTESIAN_POINT ( 'NONE',  ( 0.000000000000000000, 0.000000000000000000, 8.000000000000000000 ) ) ;
#6804=CIRCLE ( 'NONE', #9950, 56.99999999999999289 ) ;
#6807=AXIS2_PLACEMENT_3D ( 'NONE', #3223, #13618, #1029 ) ;
#6808=ORIENTED_EDGE ( 'NONE', *, *, #252, .T. ) ;
#6809=CARTESIAN_POINT ( 'NONE',  ( 2.449293598294700991E-16, -97.00000000000000000, -10.50000000000000000 ) ) ;
#6810=EDGE_CURVE ( 'NONE', #11429, #8704, #1385, .T. ) ;
#6811=CYLINDRICAL_SURFACE ( 'NONE', #12628, 60.50000000000000000 ) ;
#6812=DIRECTION ( 'NONE',  ( 0.000000000000000000, 0.000000000000000000, 1.000000000000000000 ) ) ;
#6813=CIRCLE ( 'NONE', #8509, 3.000000000000002665 ) ;
#6815=DIRECTION ( 'NONE',  ( -1.000000000000000000, 0.000000000000000000, 0.000000000000000000 ) ) ;
#6818=ORIENTED_EDGE ( 'NONE', *, *, #13781, .T. ) ;
#6819=CARTESIAN_POINT ( 'NONE',  ( 0.000000000000000000, 0.000000000000000000, -8.000000000000000000 ) ) ;
#6821=DIRECTION ( 'NONE',  ( -1.000000000000000000, 0.000000000000000000, 0.000000000000000000 ) ) ;
#6822=AXIS2_PLACEMENT_3D ( 'NONE', #13692, #13771, #14832 ) ;
#6824=EDGE_CURVE ( 'NONE', #7767, #10678, #5025, .T. ) ;
#6825=EDGE_LOOP ( 'NONE', ( #14028, #10727, #5178, #11515 ) ) ;
#6826=CARTESIAN_POINT ( 'NONE',  ( 0.000000000000000000, 0.000000000000000000, -10.50000000000000000 ) ) ;
#6828=CYLINDRICAL_SURFACE ( 'NONE', #2526, 0.5000000000000073275 ) ;
#6829=ADVANCED_FACE ( 'NONE', ( #12999 ), #2589, .T. ) ;
#6830=CIRCLE ( 'NONE', #11473, 50.00000000000000000 ) ;
#6831=ORIENTED_EDGE ( 'NONE', *, *, #3646, .T. ) ;
#6834=DIRECTION ( 'NONE',  ( 1.000000000000000000, 0.000000000000000000, 0.000000000000000000 ) ) ;
#6835=CARTESIAN_POINT ( 'NONE',  ( -97.00000000000000000, 1.015776140243522349E-12, -8.000000000000000000 ) ) ;
#6838=AXIS2_PLACEMENT_3D ( 'NONE', #4534, #12575, #11597 ) ;
#6839=DIRECTION ( 'NONE',  ( 0.000000000000000000, 0.000000000000000000, -1.000000000000000000 ) ) ;
#6840=ORIENTED_EDGE ( 'NONE', *, *, #8925, .F. ) ;
#6842=FACE_OUTER_BOUND ( 'NONE', #4619, .T. ) ;
#6843=DIRECTION ( 'NONE',  ( 0.000000000000000000, 0.000000000000000000, 1.000000000000000000 ) ) ;
#6844=EDGE_CURVE ( 'NONE', #8906, #4183, #9218, .T. ) ;
#6846=FACE_OUTER_BOUND ( 'NONE', #6071, .T. ) ;
#6847=DIRECTION ( 'NONE',  ( -1.000000000000000000, 0.000000000000000000, 0.000000000000000000 ) ) ;
#6848=CIRCLE ( 'NONE', #9756, 53.55662432702593634 ) ;
#6849=EDGE_LOOP ( 'NONE', ( #2577, #2413, #4660, #1439 ) ) ;
#6850=CARTESIAN_POINT ( 'NONE',  ( -37.12029293941441210, -89.61631465359452875, -13.00000000000000178 ) ) ;
#6855=CARTESIAN_POINT ( 'NONE',  ( -68.09867107463028901, -68.49330278050098286, -10.50000000000000000 ) ) ;
#6857=VERTEX_POINT ( 'NONE', #2881 ) ;
#6858=ORIENTED_EDGE ( 'NONE', *, *, #4537, .T. ) ;
#6859=VERTEX_POINT ( 'NONE', #617 ) ;
#6860=DIRECTION ( 'NONE',  ( 0.000000000000000000, 0.000000000000000000, 1.000000000000000000 ) ) ;
#6862=EDGE_CURVE ( 'NONE', #14718, #13762, #10, .T. ) ;
#6865=EDGE_LOOP ( 'NONE', ( #3916, #9371, #7326, #7618 ) ) ;
#6867=EDGE_LOOP ( 'NONE', ( #3158, #932, #4226, #2890, #11599, #683, #1324, #5372, #5214, #12034 ) ) ;
#6868=ORIENTED_EDGE ( 'NONE', *, *, #14202, .F. ) ;
#6869=CARTESIAN_POINT ( 'NONE',  ( 0.000000000000000000, 0.000000000000000000, -10.50000000000000000 ) ) ;
#6870=DIRECTION ( 'NONE',  ( -0.000000000000000000, -0.000000000000000000, 1.000000000000000000 ) ) ;
#6872=CIRCLE ( 'NONE', #340, 60.49999999999999289 ) ;
#6873=CARTESIAN_POINT ( 'NONE',  ( -42.04772703543551415, -32.26435573746212526, -13.00000000000000178 ) ) ;
#6875=CIRCLE ( 'NONE', #5672, 3.000000000000002665 ) ;
#6876=VERTEX_POINT ( 'NONE', #1130 ) ;
#6879=CARTESIAN_POINT ( 'NONE',  ( -68.58935777509570642, -68.58935777509452691, -10.50000000000000000 ) ) ;
#6880=CARTESIAN_POINT ( 'NONE',  ( 44.79355920668812274, 31.05588327715851449, -13.00000000000000178 ) ) ;
#6881=ORIENTED_EDGE ( 'NONE', *, *, #4866, .F. ) ;
#6882=ORIENTED_EDGE ( 'NONE', *, *, #6741, .F. ) ;
#6883=CIRCLE ( 'NONE', #7128, 53.55662432702593634 ) ;
#6885=CIRCLE ( 'NONE', #4244, 0.5000000000000004441 ) ;
#6886=AXIS2_PLACEMENT_3D ( 'NONE', #8162, #112, #6017 ) ;
#6887=EDGE_CURVE ( 'NONE', #2976, #5777, #5822, .T. ) ;
#6888=CIRCLE ( 'NONE', #11529, 53.55662432702593634 ) ;
#6889=VERTEX_POINT ( 'NONE', #11302 ) ;
#6890=EDGE_CURVE ( 'NONE', #14223, #11178, #8978, .T. ) ;
#6891=DIRECTION ( 'NONE',  ( -1.000000000000000000, 0.000000000000000000, 0.000000000000000000 ) ) ;
#6893=DIRECTION ( 'NONE',  ( 0.000000000000000000, 0.000000000000000000, -1.000000000000000000 ) ) ;
#6894=PLANE ( 'NONE',  #8005 ) ;
#6895=AXIS2_PLACEMENT_3D ( 'NONE', #2486, #5896, #12818 ) ;
#6898=CIRCLE ( 'NONE', #10782, 3.000000000000004441 ) ;
#6899=AXIS2_PLACEMENT_3D ( 'NONE', #3774, #2620, #7234 ) ;
#6900=EDGE_CURVE ( 'NONE', #10355, #1483, #12155, .T. ) ;
#6901=DIRECTION ( 'NONE',  ( 1.000000000000000000, 0.000000000000000000, 0.000000000000000000 ) ) ;
#6902=CIRCLE ( 'NONE', #7631, 53.55662432702593634 ) ;
#6903=CARTESIAN_POINT ( 'NONE',  ( -25.99999999999971223, -45.89934640057541060, 10.49999999999999822 ) ) ;
#6904=ORIENTED_EDGE ( 'NONE', *, *, #6511, .T. ) ;
#6905=EDGE_CURVE ( 'NONE', #7720, #12891, #5119, .T. ) ;
#6906=DIRECTION ( 'NONE',  ( 0.000000000000000000, 0.000000000000000000, 1.000000000000000000 ) ) ;
#6908=DIRECTION ( 'NONE',  ( -1.000000000000000000, 0.000000000000000000, 0.000000000000000000 ) ) ;
#6909=ADVANCED_FACE ( 'NONE', ( #6718 ), #6356, .F. ) ;
#6911=CIRCLE ( 'NONE', #9096, 52.50000000000000711 ) ;
#6912=CARTESIAN_POINT ( 'NONE',  ( -45.88839665196098849, 26.99988008862674960, -13.00000000000000178 ) ) ;
#6913=CARTESIAN_POINT ( 'NONE',  ( 0.000000000000000000, 0.000000000000000000, -8.000000000000000000 ) ) ;
#6914=CARTESIAN_POINT ( 'NONE',  ( -29.26435573746199381, 42.04772703543562073, 8.000000000000000000 ) ) ;
#6915=FACE_OUTER_BOUND ( 'NONE', #10640, .T. ) ;
#6917=DIRECTION ( 'NONE',  ( -0.000000000000000000, -0.000000000000000000, -1.000000000000000000 ) ) ;
#6918=AXIS2_PLACEMENT_3D ( 'NONE', #10552, #221, #9623 ) ;
#6921=CARTESIAN_POINT ( 'NONE',  ( 26.01438936481372721, 47.21331623427104063, 10.49999999999999822 ) ) ;
#6922=CARTESIAN_POINT ( 'NONE',  ( -10.71740939043329099, 51.19406879332069593, 8.000000000000000000 ) ) ;
#6923=CARTESIAN_POINT ( 'NONE',  ( 0.000000000000000000, 0.000000000000000000, 8.000000000000000000 ) ) ;
#6925=CYLINDRICAL_SURFACE ( 'NONE', #13366, 0.5000000000000073275 ) ;
#6926=ORIENTED_EDGE ( 'NONE', *, *, #321, .T. ) ;
#6929=EDGE_CURVE ( 'NONE', #2714, #7912, #10444, .T. ) ;
#6930=DIRECTION ( 'NONE',  ( 1.000000000000000000, 1.765157221169382931E-15, 0.000000000000000000 ) ) ;
#6932=DIRECTION ( 'NONE',  ( -0.000000000000000000, -0.000000000000000000, 1.000000000000000000 ) ) ;
#6933=ORIENTED_EDGE ( 'NONE', *, *, #5369, .F. ) ;
#6934=CIRCLE ( 'NONE', #1384, 0.5000000000000004441 ) ;
#6935=ORIENTED_EDGE ( 'NONE', *, *, #321, .F. ) ;
#6936=VECTOR ( 'NONE', #3142, 1000.000000000000000 ) ;
#6937=CARTESIAN_POINT ( 'NONE',  ( 90.11631465359468507, -37.12029293941410657, 10.49999999999999822 ) ) ;
#6938=CARTESIAN_POINT ( 'NONE',  ( 97.00000000000000000, -3.384287605079545030E-13, 8.000000000000000000 ) ) ;
#6939=CYLINDRICAL_SURFACE ( 'NONE', #59, 50.00000000000000000 ) ;
#6940=EDGE_LOOP ( 'NONE', ( #11935, #1456, #13044, #190, #11643 ) ) ;
#6943=ORIENTED_EDGE ( 'NONE', *, *, #11550, .F. ) ;
#6944=ORIENTED_EDGE ( 'NONE', *, *, #10831, .F. ) ;
#6946=DIRECTION ( 'NONE',  ( 0.000000000000000000, 0.000000000000000000, 1.000000000000000000 ) ) ;
#6950=CARTESIAN_POINT ( 'NONE',  ( -37.12029293941441210, -89.61631465359452875, -13.00000000000000178 ) ) ;
#6951=ORIENTED_EDGE ( 'NONE', *, *, #6263, .T. ) ;
#6952=DIRECTION ( 'NONE',  ( 1.000000000000000000, 0.000000000000000000, 0.000000000000000000 ) ) ;
#6953=ORIENTED_EDGE ( 'NONE', *, *, #10812, .F. ) ;
#6954=DIRECTION ( 'NONE',  ( 0.000000000000000000, 0.000000000000000000, 1.000000000000000000 ) ) ;
#6955=CARTESIAN_POINT ( 'NONE',  ( 37.02125851216354846, -90.10640870805738700, 10.49999999999999822 ) ) ;
#6956=EDGE_LOOP ( 'NONE', ( #3660, #282, #13658, #12189 ) ) ;
#6957=ORIENTED_EDGE ( 'NONE', *, *, #2721, .T. ) ;
#6958=CARTESIAN_POINT ( 'NONE',  ( 13.35619814848834075, -51.53979475227123430, -13.00000000000000178 ) ) ;
#6959=ORIENTED_EDGE ( 'NONE', *, *, #9036, .F. ) ;
#6965=DIRECTION ( 'NONE',  ( 0.000000000000000000, 0.000000000000000000, 1.000000000000000000 ) ) ;
#6966=ORIENTED_EDGE ( 'NONE', *, *, #8762, .F. ) ;
#6969=ADVANCED_FACE ( 'NONE', ( #8716 ), #9155, .F. ) ;
#6970=DIRECTION ( 'NONE',  ( -1.000000000000000000, 0.000000000000000000, 0.000000000000000000 ) ) ;
#6971=EDGE_CURVE ( 'NONE', #13693, #6509, #10210, .T. ) ;
#6973=VERTEX_POINT ( 'NONE', #13645 ) ;
#6975=ORIENTED_EDGE ( 'NONE', *, *, #4723, .T. ) ;
#6976=DIRECTION ( 'NONE',  ( 0.000000000000000000, 0.000000000000000000, -1.000000000000000000 ) ) ;
#6981=CARTESIAN_POINT ( 'NONE',  ( 32.26435573746228158, -42.04772703543541468, -8.000000000000000000 ) ) ;
#6982=ORIENTED_EDGE ( 'NONE', *, *, #3838, .F. ) ;
#6983=EDGE_CURVE ( 'NONE', #9441, #13119, #2692, .T. ) ;
#6986=DIRECTION ( 'NONE',  ( 0.000000000000000000, 0.000000000000000000, 1.000000000000000000 ) ) ;
#6987=CYLINDRICAL_SURFACE ( 'NONE', #5160, 63.00000000000000000 ) ;
#6988=CARTESIAN_POINT ( 'NONE',  ( -3.492805317593278058, 46.55633131742322917, -10.50000000000000000 ) ) ;
#6990=DIRECTION ( 'NONE',  ( 0.000000000000000000, 0.000000000000000000, 1.000000000000000000 ) ) ;
#6991=ORIENTED_EDGE ( 'NONE', *, *, #4069, .F. ) ;
#6996=CARTESIAN_POINT ( 'NONE',  ( 0.000000000000000000, 0.000000000000000000, -10.50000000000000000 ) ) ;
#6997=ORIENTED_EDGE ( 'NONE', *, *, #12618, .T. ) ;
#6998=ORIENTED_EDGE ( 'NONE', *, *, #3671, .T. ) ;
#7001=DIRECTION ( 'NONE',  ( -0.000000000000000000, -0.000000000000000000, -1.000000000000000000 ) ) ;
#7006=EDGE_LOOP ( 'NONE', ( #7543, #1520, #6671, #13297, #1805, #13660 ) ) ;
#7007=ORIENTED_EDGE ( 'NONE', *, *, #9123, .T. ) ;
#7008=EDGE_CURVE ( 'NONE', #1677, #10850, #12643, .T. ) ;
#7009=CARTESIAN_POINT ( 'NONE',  ( 0.000000000000000000, 0.000000000000000000, -10.50000000000000000 ) ) ;
#7010=CIRCLE ( 'NONE', #12365, 56.99999999999999289 ) ;
#7013=DIRECTION ( 'NONE',  ( 0.000000000000000000, 0.000000000000000000, 1.000000000000000000 ) ) ;
#7014=EDGE_CURVE ( 'NONE', #11546, #9586, #14092, .T. ) ;
#7016=VERTEX_POINT ( 'NONE', #7090 ) ;
#7017=CARTESIAN_POINT ( 'NONE',  ( 4.121772567811984089, 51.45950017607689375, -8.000000000000000000 ) ) ;
#7018=EDGE_LOOP ( 'NONE', ( #3934, #7425, #11379, #10122, #2175, #3243, #5797, #1419, #2476, #1817, #5985 ) ) ;
#7019=AXIS2_PLACEMENT_3D ( 'NONE', #9631, #6142, #2816 ) ;
#7020=CARTESIAN_POINT ( 'NONE',  ( -23.49999999999971223, -45.89934640057541060, -8.000000000000000000 ) ) ;
#7021=LINE ( 'NONE', #12965, #14500 ) ;
#7022=ORIENTED_EDGE ( 'NONE', *, *, #2823, .F. ) ;
#7023=EDGE_CURVE ( 'NONE', #3583, #12891, #8169, .T. ) ;
#7024=VECTOR ( 'NONE', #14977, 1000.000000000000000 ) ;
#7025=EDGE_CURVE ( 'NONE', #12545, #4523, #8991, .T. ) ;
#7026=VERTEX_POINT ( 'NONE', #5803 ) ;
#7027=DIRECTION ( 'NONE',  ( -0.000000000000000000, -0.000000000000000000, 1.000000000000000000 ) ) ;
#7028=AXIS2_PLACEMENT_3D ( 'NONE', #3737, #3881, #3957 ) ;
#7029=VERTEX_POINT ( 'NONE', #11896 ) ;
#7030=CARTESIAN_POINT ( 'NONE',  ( 0.000000000000000000, 0.000000000000000000, -8.000000000000000000 ) ) ;
#7031=DIRECTION ( 'NONE',  ( 1.000000000000000000, 0.000000000000000000, 0.000000000000000000 ) ) ;
#7032=CARTESIAN_POINT ( 'NONE',  ( 0.000000000000000000, 0.000000000000000000, -8.000000000000000000 ) ) ;
#7036=ORIENTED_EDGE ( 'NONE', *, *, #4326, .T. ) ;
#7037=DIRECTION ( 'NONE',  ( 0.000000000000000000, 0.000000000000000000, 1.000000000000000000 ) ) ;
#7038=CIRCLE ( 'NONE', #758, 3.000000000000002665 ) ;
#7039=DIRECTION ( 'NONE',  ( 0.000000000000000000, 0.000000000000000000, 1.000000000000000000 ) ) ;
#7043=CIRCLE ( 'NONE', #4404, 0.5000000000000004441 ) ;
#7044=VERTEX_POINT ( 'NONE', #1346 ) ;
#7045=CARTESIAN_POINT ( 'NONE',  ( 9.706953719245472456, 57.06275842387054098, -10.50000000000000000 ) ) ;
#7046=ORIENTED_EDGE ( 'NONE', *, *, #9431, .F. ) ;
#7048=CARTESIAN_POINT ( 'NONE',  ( 38.26834323650837888, -92.38795325112893408, 8.000000000000000000 ) ) ;
#7049=ORIENTED_EDGE ( 'NONE', *, *, #13360, .T. ) ;
#7052=DIRECTION ( 'NONE',  ( 0.000000000000000000, 0.000000000000000000, 1.000000000000000000 ) ) ;
#7053=DIRECTION ( 'NONE',  ( -1.000000000000000000, 0.000000000000000000, 0.000000000000000000 ) ) ;
#7055=CYLINDRICAL_SURFACE ( 'NONE', #6505, 60.50000000000000711 ) ;
#7057=CARTESIAN_POINT ( 'NONE',  ( 45.96504489226007450, -23.50071946824056823, -8.000000000000000000 ) ) ;
#7060=CARTESIAN_POINT ( 'NONE',  ( 0.2790467552932217044, -96.58511096861892042, -13.00000000000000178 ) ) ;
#7062=VECTOR ( 'NONE', #4412, 1000.000000000000000 ) ;
#7064=LINE ( 'NONE', #12559, #7841 ) ;
#7066=EDGE_CURVE ( 'NONE', #7077, #13418, #3551, .T. ) ;
#7067=CYLINDRICAL_SURFACE ( 'NONE', #1257, 52.50000000000000711 ) ;
#7069=AXIS2_PLACEMENT_3D ( 'NONE', #5950, #12107, #14159 ) ;
#7071=CYLINDRICAL_SURFACE ( 'NONE', #12370, 3.000000000000002665 ) ;
#7072=EDGE_CURVE ( 'NONE', #10615, #4717, #4685, .T. ) ;
#7074=CYLINDRICAL_SURFACE ( 'NONE', #10459, 3.000000000000002665 ) ;
#7075=DIRECTION ( 'NONE',  ( -1.000000000000000000, 0.000000000000000000, 0.000000000000000000 ) ) ;
#7077=VERTEX_POINT ( 'NONE', #13033 ) ;
#7078=DIRECTION ( 'NONE',  ( 0.000000000000000000, 0.000000000000000000, -1.000000000000000000 ) ) ;
#7079=CARTESIAN_POINT ( 'NONE',  ( 45.46633369868310837, -26.24999999999987921, -10.50000000000000000 ) ) ;
#7080=AXIS2_PLACEMENT_3D ( 'NONE', #4471, #12809, #5670 ) ;
#7081=AXIS2_PLACEMENT_3D ( 'NONE', #4295, #5345, #10120 ) ;
#7082=DIRECTION ( 'NONE',  ( 1.000000000000000000, 0.000000000000000000, 0.000000000000000000 ) ) ;
#7084=VERTEX_POINT ( 'NONE', #2392 ) ;
#7085=CIRCLE ( 'NONE', #13915, 100.0000000000000000 ) ;
#7086=EDGE_LOOP ( 'NONE', ( #4, #8691, #14482, #11683 ) ) ;
#7088=FACE_OUTER_BOUND ( 'NONE', #12869, .T. ) ;
#7089=VECTOR ( 'NONE', #10167, 1000.000000000000000 ) ;
#7090=CARTESIAN_POINT ( 'NONE',  ( 9.154234823626464946E-15, 100.0000000000000000, -8.000000000000000000 ) ) ;
#7092=CARTESIAN_POINT ( 'NONE',  ( -13.60620885621536935, 51.79945067148138094, -10.50000000000000000 ) ) ;
#7093=CARTESIAN_POINT ( 'NONE',  ( -2.449293598294708880E-16, 38.00000000000000000, -28.00000000000000000 ) ) ;
#7094=ADVANCED_FACE ( 'NONE', ( #4827 ), #5956, .T. ) ;
#7098=AXIS2_PLACEMENT_3D ( 'NONE', #12794, #3538, #5653 ) ;
#7099=DIRECTION ( 'NONE',  ( 0.000000000000000000, 0.000000000000000000, 1.000000000000000000 ) ) ;
#7100=ORIENTED_EDGE ( 'NONE', *, *, #13393, .T. ) ;
#7101=CIRCLE ( 'NONE', #574, 63.00000000000000000 ) ;
#7102=ORIENTED_EDGE ( 'NONE', *, *, #3186, .F. ) ;
#7104=ORIENTED_EDGE ( 'NONE', *, *, #10575, .F. ) ;
#7106=AXIS2_PLACEMENT_3D ( 'NONE', #5514, #12349, #14778 ) ;
#7108=DIRECTION ( 'NONE',  ( 1.000000000000000000, 0.000000000000000000, 0.000000000000000000 ) ) ;
#7109=AXIS2_PLACEMENT_3D ( 'NONE', #14757, #14042, #7113 ) ;
#7111=CARTESIAN_POINT ( 'NONE',  ( -44.79355920668832880, -31.05588327715819474, -13.00000000000000178 ) ) ;
#7112=EDGE_CURVE ( 'NONE', #5604, #3464, #9474, .T. ) ;
#7113=DIRECTION ( 'NONE',  ( -1.000000000000000000, 0.000000000000000000, 0.000000000000000000 ) ) ;
#7114=DIRECTION ( 'NONE',  ( 0.000000000000000000, 0.000000000000000000, -1.000000000000000000 ) ) ;
#7116=ORIENTED_EDGE ( 'NONE', *, *, #13743, .F. ) ;
#7117=DIRECTION ( 'NONE',  ( -1.000000000000000000, 0.000000000000000000, 0.000000000000000000 ) ) ;
#7118=EDGE_CURVE ( 'NONE', #2051, #345, #4888, .T. ) ;
#7123=EDGE_CURVE ( 'NONE', #7242, #6515, #8751, .T. ) ;
#7124=DIRECTION ( 'NONE',  ( -1.000000000000000000, 0.000000000000000000, 0.000000000000000000 ) ) ;
#7126=DIRECTION ( 'NONE',  ( 1.000000000000000000, -1.765157221169382931E-15, 0.000000000000000000 ) ) ;
#7127=AXIS2_PLACEMENT_3D ( 'NONE', #4742, #4442, #1240 ) ;
#7128=AXIS2_PLACEMENT_3D ( 'NONE', #14319, #6254, #3931 ) ;
#7130=DIRECTION ( 'NONE',  ( 1.000000000000000000, 0.000000000000000000, 0.000000000000000000 ) ) ;
#7131=CARTESIAN_POINT ( 'NONE',  ( 13.71740939043365337, -51.19406879332061067, -8.000000000000000000 ) ) ;
#7132=AXIS2_PLACEMENT_3D ( 'NONE', #5137, #430, #5968 ) ;
#7137=EDGE_LOOP ( 'NONE', ( #3254, #953, #13048, #11096 ) ) ;
#7138=CARTESIAN_POINT ( 'NONE',  ( -15.88467684210512942, 49.11971303961693280, -8.000000000000000000 ) ) ;
#7139=ORIENTED_EDGE ( 'NONE', *, *, #700, .F. ) ;
#7141=DIRECTION ( 'NONE',  ( 1.000000000000000000, 0.000000000000000000, 0.000000000000000000 ) ) ;
#7143=DIRECTION ( 'NONE',  ( -0.000000000000000000, -0.000000000000000000, -1.000000000000000000 ) ) ;
#7144=CIRCLE ( 'NONE', #12985, 3.000000000000002665 ) ;
#7145=AXIS2_PLACEMENT_3D ( 'NONE', #14039, #5904, #148 ) ;
#7146=CARTESIAN_POINT ( 'NONE',  ( -4.121772567811602173, -51.45950017607692217, 8.000000000000000000 ) ) ;
#7149=VERTEX_POINT ( 'NONE', #9743 ) ;
#7150=ORIENTED_EDGE ( 'NONE', *, *, #3112, .T. ) ;
#7151=CARTESIAN_POINT ( 'NONE',  ( -6.917888187662729393, -52.54657765281195481, 8.000000000000000000 ) ) ;
#7152=DIRECTION ( 'NONE',  ( 1.000000000000000000, 0.000000000000000000, 0.000000000000000000 ) ) ;
#7154=AXIS2_PLACEMENT_3D ( 'NONE', #2271, #11549, #10236 ) ;
#7155=DIRECTION ( 'NONE',  ( 1.000000000000000000, 0.000000000000000000, 0.000000000000000000 ) ) ;
#7156=CARTESIAN_POINT ( 'NONE',  ( -92.55687898036933348, -36.52608637591544039, -8.000000000000000000 ) ) ;
#7159=DIRECTION ( 'NONE',  ( 1.000000000000000000, 0.000000000000000000, 0.000000000000000000 ) ) ;
#7160=DIRECTION ( 'NONE',  ( 0.000000000000000000, 0.000000000000000000, 1.000000000000000000 ) ) ;
#7162=EDGE_CURVE ( 'NONE', #13279, #4787, #20, .T. ) ;
#7163=AXIS2_PLACEMENT_3D ( 'NONE', #5886, #14026, #8171 ) ;
#7164=ORIENTED_EDGE ( 'NONE', *, *, #12941, .F. ) ;
#7165=EDGE_CURVE ( 'NONE', #14898, #7167, #3912, .T. ) ;
#7167=VERTEX_POINT ( 'NONE', #7319 ) ;
#7169=CARTESIAN_POINT ( 'NONE',  ( 89.61631465359491244, 37.12029293941346708, 8.000000000000000000 ) ) ;
#7170=PLANE ( 'NONE',  #2495 ) ;
#7173=AXIS2_PLACEMENT_3D ( 'NONE', #9292, #10214, #1120 ) ;
#7176=DIRECTION ( 'NONE',  ( -1.000000000000000000, 0.000000000000000000, 0.000000000000000000 ) ) ;
#7177=CARTESIAN_POINT ( 'NONE',  ( -51.19406879332065330, -13.71740939043347041, -8.000000000000000000 ) ) ;
#7178=CARTESIAN_POINT ( 'NONE',  ( -9.706953719245875689, -57.06275842387046993, -10.50000000000000000 ) ) ;
#7180=EDGE_CURVE ( 'NONE', #3301, #6492, #2925, .T. ) ;
#7181=ORIENTED_EDGE ( 'NONE', *, *, #5724, .T. ) ;
#7182=VERTEX_POINT ( 'NONE', #2851 ) ;
#7183=CARTESIAN_POINT ( 'NONE',  ( -49.11971303961688307, -15.88467684210530528, -13.00000000000000178 ) ) ;
#7185=ORIENTED_EDGE ( 'NONE', *, *, #42, .T. ) ;
#7186=DIRECTION ( 'NONE',  ( 0.000000000000000000, 0.000000000000000000, 1.000000000000000000 ) ) ;
#7187=DIRECTION ( 'NONE',  ( 0.000000000000000000, 0.000000000000000000, -1.000000000000000000 ) ) ;
#7189=DIRECTION ( 'NONE',  ( 0.000000000000000000, 0.000000000000000000, 1.000000000000000000 ) ) ;
#7192=CARTESIAN_POINT ( 'NONE',  ( -71.53347797788821083, -69.16568774265570596, 8.000000000000000000 ) ) ;
#7194=DIRECTION ( 'NONE',  ( 1.000000000000000000, 0.000000000000000000, 0.000000000000000000 ) ) ;
#7198=EDGE_CURVE ( 'NONE', #12633, #5385, #7281, .T. ) ;
#7200=EDGE_CURVE ( 'NONE', #8562, #2510, #13121, .T. ) ;
#7201=CARTESIAN_POINT ( 'NONE',  ( 49.00442420935993226, -30.80502811811213704, 8.000000000000000000 ) ) ;
#7202=EDGE_CURVE ( 'NONE', #6323, #5248, #1963, .T. ) ;
#7203=CARTESIAN_POINT ( 'NONE',  ( 9.706953719245472456, 57.06275842387054098, -8.000000000000000000 ) ) ;
#7204=CIRCLE ( 'NONE', #3833, 100.0000000000000000 ) ;
#7206=DIRECTION ( 'NONE',  ( -0.000000000000000000, -0.000000000000000000, -1.000000000000000000 ) ) ;
#7208=FACE_OUTER_BOUND ( 'NONE', #401, .T. ) ;
#7209=ORIENTED_EDGE ( 'NONE', *, *, #8944, .F. ) ;
#7211=CARTESIAN_POINT ( 'NONE',  ( -12.86891638962156215, 56.43380494353993271, -13.00000000000000178 ) ) ;
#7212=ORIENTED_EDGE ( 'NONE', *, *, #6151, .F. ) ;
#7213=CARTESIAN_POINT ( 'NONE',  ( 90.11631465359491244, 37.12029293941346708, -10.50000000000000000 ) ) ;
#7214=CARTESIAN_POINT ( 'NONE',  ( 27.01438936481372721, 47.21331623427104063, -13.00000000000000178 ) ) ;
#7217=EDGE_CURVE ( 'NONE', #9394, #3039, #14328, .T. ) ;
#7219=ADVANCED_FACE ( 'NONE', ( #6319 ), #6400, .F. ) ;
#7221=DIRECTION ( 'NONE',  ( -0.000000000000000000, -0.000000000000000000, 1.000000000000000000 ) ) ;
#7222=ORIENTED_EDGE ( 'NONE', *, *, #12075, .F. ) ;
#7224=DIRECTION ( 'NONE',  ( -0.000000000000000000, -0.000000000000000000, 1.000000000000000000 ) ) ;
#7225=DIRECTION ( 'NONE',  ( -0.000000000000000000, -0.000000000000000000, -1.000000000000000000 ) ) ;
#7226=DIRECTION ( 'NONE',  ( -0.000000000000000000, -0.000000000000000000, -1.000000000000000000 ) ) ;
#7227=VERTEX_POINT ( 'NONE', #1641 ) ;
#7228=CYLINDRICAL_SURFACE ( 'NONE', #2819, 59.50000000000000000 ) ;
#7229=DIRECTION ( 'NONE',  ( 0.000000000000000000, 0.000000000000000000, 1.000000000000000000 ) ) ;
#7230=CARTESIAN_POINT ( 'NONE',  ( -57.06275842387042729, 9.706953719246069312, -10.50000000000000000 ) ) ;
#7233=ORIENTED_EDGE ( 'NONE', *, *, #7066, .T. ) ;
#7234=DIRECTION ( 'NONE',  ( 1.000000000000000000, 0.000000000000000000, 0.000000000000000000 ) ) ;
#7237=CARTESIAN_POINT ( 'NONE',  ( -53.55662432702593634, 0.000000000000000000, -10.50000000000000000 ) ) ;
#7242=VERTEX_POINT ( 'NONE', #4075 ) ;
#7243=VERTEX_POINT ( 'NONE', #13321 ) ;
#7244=LINE ( 'NONE', #10829, #5690 ) ;
#7245=AXIS2_PLACEMENT_3D ( 'NONE', #4491, #13822, #13752 ) ;
#7248=ORIENTED_EDGE ( 'NONE', *, *, #12793, .T. ) ;
#7250=DIRECTION ( 'NONE',  ( 1.000000000000000000, 0.000000000000000000, 0.000000000000000000 ) ) ;
#7251=PRODUCT_DEFINITION_FORMATION_WITH_SPECIFIED_SOURCE ( 'ANY', '', #7917, .NOT_KNOWN. ) ;
#7252=ORIENTED_EDGE ( 'NONE', *, *, #12933, .T. ) ;
#7253=CIRCLE ( 'NONE', #7791, 0.5000000000000073275 ) ;
#7254=FACE_OUTER_BOUND ( 'NONE', #13944, .T. ) ;
#7255=EDGE_CURVE ( 'NONE', #1613, #6509, #10129, .T. ) ;
#7256=VECTOR ( 'NONE', #14431, 1000.000000000000000 ) ;
#7258=DIRECTION ( 'NONE',  ( 0.000000000000000000, 0.000000000000000000, 1.000000000000000000 ) ) ;
#7260=EDGE_CURVE ( 'NONE', #5893, #7516, #5355, .T. ) ;
#7261=ORIENTED_EDGE ( 'NONE', *, *, #14579, .F. ) ;
#7262=DIRECTION ( 'NONE',  ( 0.000000000000000000, 0.000000000000000000, -1.000000000000000000 ) ) ;
#7264=ORIENTED_EDGE ( 'NONE', *, *, #4500, .T. ) ;
#7265=DIRECTION ( 'NONE',  ( 1.000000000000000000, 0.000000000000000000, 0.000000000000000000 ) ) ;
#7266=VECTOR ( 'NONE', #12531, 1000.000000000000000 ) ;
#7267=CIRCLE ( 'NONE', #9939, 59.50000000000000000 ) ;
#7268=EDGE_CURVE ( 'NONE', #11211, #4485, #5573, .T. ) ;
#7269=VERTEX_POINT ( 'NONE', #3231 ) ;
#7270=AXIS2_PLACEMENT_3D ( 'NONE', #10033, #11035, #5262 ) ;
#7271=COLOUR_RGB ( '', 0.09019608, 0.27058824, 0.51372549) ;
#7272=ORIENTED_EDGE ( 'NONE', *, *, #62, .T. ) ;
#7274=CYLINDRICAL_SURFACE ( 'NONE', #354, 0.5000000000000004441 ) ;
#7277=AXIS2_PLACEMENT_3D ( 'NONE', #371, #13124, #5976 ) ;
#7278=DIRECTION ( 'NONE',  ( -1.000000000000000000, 0.000000000000000000, 0.000000000000000000 ) ) ;
#7281=CIRCLE ( 'NONE', #760, 60.49999999999999289 ) ;
#7282=CARTESIAN_POINT ( 'NONE',  ( -49.57224306869049713, 6.526309611002760747, -8.000000000000000000 ) ) ;
#7284=AXIS2_PLACEMENT_3D ( 'NONE', #8456, #12049, #346 ) ;
#7285=VERTEX_POINT ( 'NONE', #9982 ) ;
#7287=ORIENTED_EDGE ( 'NONE', *, *, #3575, .T. ) ;
#7288=ADVANCED_FACE ( 'NONE', ( #7775 ), #12417, .T. ) ;
#7290=DIRECTION ( 'NONE',  ( -1.000000000000000000, 0.000000000000000000, 0.000000000000000000 ) ) ;
#7291=AXIS2_PLACEMENT_3D ( 'NONE', #14117, #14337, #2805 ) ;
#7292=DIRECTION ( 'NONE',  ( 1.000000000000000000, 0.000000000000000000, 0.000000000000000000 ) ) ;
#7296=VERTEX_POINT ( 'NONE', #14628 ) ;
#7297=DIRECTION ( 'NONE',  ( 0.000000000000000000, 0.000000000000000000, -1.000000000000000000 ) ) ;
#7298=ORIENTED_EDGE ( 'NONE', *, *, #6905, .T. ) ;
#7299=CARTESIAN_POINT ( 'NONE',  ( 9.706953719245472456, 57.06275842387054098, 8.000000000000000000 ) ) ;
#7301=AXIS2_PLACEMENT_3D ( 'NONE', #1630, #12884, #12041 ) ;
#7303=DIRECTION ( 'NONE',  ( 0.000000000000000000, 0.000000000000000000, -1.000000000000000000 ) ) ;
#7304=ADVANCED_FACE ( 'NONE', ( #11285 ), #4526, .F. ) ;
#7305=EDGE_LOOP ( 'NONE', ( #5533, #4712, #4219, #13744, #3310 ) ) ;
#7309=CARTESIAN_POINT ( 'NONE',  ( 56.43380494353997534, 12.86891638962136319, -13.00000000000000178 ) ) ;
#7311=DIRECTION ( 'NONE',  ( -1.000000000000000000, 8.746504920891464822E-16, 0.000000000000000000 ) ) ;
#7313=EDGE_LOOP ( 'NONE', ( #10166, #3037, #10289, #14124, #6795, #6313, #1360 ) ) ;
#7314=ADVANCED_FACE ( 'NONE', ( #4227 ), #14929, .T. ) ;
#7315=FACE_OUTER_BOUND ( 'NONE', #549, .T. ) ;
#7316=ORIENTED_EDGE ( 'NONE', *, *, #171, .T. ) ;
#7317=AXIS2_PLACEMENT_3D ( 'NONE', #3132, #10181, #3210 ) ;
#7318=FACE_OUTER_BOUND ( 'NONE', #6122, .T. ) ;
#7319=CARTESIAN_POINT ( 'NONE',  ( -52.72775723226775568, 7.383907457638128058, 10.49999999999999822 ) ) ;
#7322=ORIENTED_EDGE ( 'NONE', *, *, #4882, .T. ) ;
#7324=AXIS2_PLACEMENT_3D ( 'NONE', #8454, #3769, #10738 ) ;
#7325=EDGE_CURVE ( 'NONE', #3583, #877, #12853, .T. ) ;
#7326=ORIENTED_EDGE ( 'NONE', *, *, #5151, .F. ) ;
#7328=CARTESIAN_POINT ( 'NONE',  ( 51.45950017607693638, -4.121772567811421872, -13.00000000000000178 ) ) ;
#7329=AXIS2_PLACEMENT_3D ( 'NONE', #14755, #12256, #2070 ) ;
#7331=ORIENTED_EDGE ( 'NONE', *, *, #9057, .F. ) ;
#7332=ORIENTED_EDGE ( 'NONE', *, *, #13781, .F. ) ;
#7333=FACE_OUTER_BOUND ( 'NONE', #14135, .T. ) ;
#7334=ORIENTED_EDGE ( 'NONE', *, *, #10063, .F. ) ;
#7335=AXIS2_PLACEMENT_3D ( 'NONE', #8369, #2749, #399 ) ;
#7337=CIRCLE ( 'NONE', #816, 3.000000000000002665 ) ;
#7339=FACE_OUTER_BOUND ( 'NONE', #4890, .T. ) ;
#7341=AXIS2_PLACEMENT_3D ( 'NONE', #13034, #2705, #9744 ) ;
#7342=DIRECTION ( 'NONE',  ( 1.000000000000000000, 0.000000000000000000, 0.000000000000000000 ) ) ;
#7344=ORIENTED_EDGE ( 'NONE', *, *, #6502, .T. ) ;
#7345=CARTESIAN_POINT ( 'NONE',  ( -32.06294366074467206, 42.50536573064442081, 10.49999999999999822 ) ) ;
#7348=VERTEX_POINT ( 'NONE', #2154 ) ;
#7349=DIRECTION ( 'NONE',  ( -1.000000000000000000, 1.953992523340275196E-14, 0.000000000000000000 ) ) ;
#7350=EDGE_CURVE ( 'NONE', #9753, #1331, #808, .T. ) ;
#7351=VERTEX_POINT ( 'NONE', #5435 ) ;
#7353=CIRCLE ( 'NONE', #10756, 0.5000000000000004441 ) ;
#7354=PLANE ( 'NONE',  #494 ) ;
#7358=EDGE_CURVE ( 'NONE', #9310, #4530, #9203, .T. ) ;
#7360=ORIENTED_EDGE ( 'NONE', *, *, #7072, .F. ) ;
#7361=AXIS2_PLACEMENT_3D ( 'NONE', #3825, #6225, #1685 ) ;
#7362=AXIS2_PLACEMENT_3D ( 'NONE', #11224, #11144, #7564 ) ;
#7364=ORIENTED_EDGE ( 'NONE', *, *, #6741, .T. ) ;
#7366=CYLINDRICAL_SURFACE ( 'NONE', #2579, 3.000000000000002665 ) ;
#7367=CARTESIAN_POINT ( 'NONE',  ( -56.43380494354004639, -12.86891638962099549, -8.000000000000000000 ) ) ;
#7371=EDGE_LOOP ( 'NONE', ( #3712, #4928, #13196, #1377, #9432, #14846, #4399, #4724, #13588 ) ) ;
#7373=AXIS2_PLACEMENT_3D ( 'NONE', #4695, #2478, #980 ) ;
#7375=CARTESIAN_POINT ( 'NONE',  ( 6.451868917687939131, 52.36539807335604024, -10.50000000000000000 ) ) ;
#7377=ORIENTED_EDGE ( 'NONE', *, *, #3615, .T. ) ;
#7378=LINE ( 'NONE', #10953, #6055 ) ;
#7383=CIRCLE ( 'NONE', #8356, 59.50000000000000711 ) ;
#7384=EDGE_LOOP ( 'NONE', ( #10482, #11929, #3857, #12570, #2846, #6944 ) ) ;
#7386=AXIS2_PLACEMENT_3D ( 'NONE', #11884, #3836, #10816 ) ;
#7387=DIRECTION ( 'NONE',  ( 0.000000000000000000, 0.000000000000000000, 1.000000000000000000 ) ) ;
#7388=FACE_OUTER_BOUND ( 'NONE', #6241, .T. ) ;
#7389=CIRCLE ( 'NONE', #14681, 100.0000000000000000 ) ;
#7390=DIRECTION ( 'NONE',  ( 0.000000000000000000, 0.000000000000000000, 1.000000000000000000 ) ) ;
#7391=ORIENTED_EDGE ( 'NONE', *, *, #5907, .T. ) ;
#7393=EDGE_CURVE ( 'NONE', #13229, #8152, #768, .T. ) ;
#7395=ORIENTED_EDGE ( 'NONE', *, *, #2224, .F. ) ;
#7396=EDGE_CURVE ( 'NONE', #14, #8885, #11888, .T. ) ;
#7397=CYLINDRICAL_SURFACE ( 'NONE', #6404, 0.5000000000000004441 ) ;
#7399=AXIS2_PLACEMENT_3D ( 'NONE', #12599, #2194, #1072 ) ;
#7401=CARTESIAN_POINT ( 'NONE',  ( 0.000000000000000000, 0.000000000000000000, -8.000000000000000000 ) ) ;
#7405=VERTEX_POINT ( 'NONE', #1178 ) ;
#7406=ORIENTED_EDGE ( 'NONE', *, *, #7260, .F. ) ;
#7409=DIRECTION ( 'NONE',  ( 1.000000000000000000, 0.000000000000000000, 0.000000000000000000 ) ) ;
#7410=FACE_OUTER_BOUND ( 'NONE', #14605, .T. ) ;
#7412=CYLINDRICAL_SURFACE ( 'NONE', #6131, 3.000000000000002665 ) ;
#7413=VERTEX_POINT ( 'NONE', #12719 ) ;
#7416=VERTEX_POINT ( 'NONE', #8077 ) ;
#7417=EDGE_CURVE ( 'NONE', #12179, #12421, #7253, .T. ) ;
#7418=AXIS2_PLACEMENT_3D ( 'NONE', #3460, #8081, #9367 ) ;
#7419=CYLINDRICAL_SURFACE ( 'NONE', #8986, 59.50000000000000000 ) ;
#7423=DIRECTION ( 'NONE',  ( -1.000000000000000000, 0.000000000000000000, 0.000000000000000000 ) ) ;
#7425=ORIENTED_EDGE ( 'NONE', *, *, #4089, .T. ) ;
#7426=CARTESIAN_POINT ( 'NONE',  ( 92.55687898036906347, 36.52608637591612961, 8.000000000000000000 ) ) ;
#7427=VECTOR ( 'NONE', #12847, 1000.000000000000000 ) ;
#7428=ORIENTED_EDGE ( 'NONE', *, *, #1664, .F. ) ;
#7429=ORIENTED_EDGE ( 'NONE', *, *, #142, .T. ) ;
#7430=DIRECTION ( 'NONE',  ( -1.000000000000000000, 0.000000000000000000, 0.000000000000000000 ) ) ;
#7433=DIRECTION ( 'NONE',  ( 0.000000000000000000, 0.000000000000000000, -1.000000000000000000 ) ) ;
#7435=DIRECTION ( 'NONE',  ( 0.000000000000000000, 0.000000000000000000, 1.000000000000000000 ) ) ;
#7437=EDGE_CURVE ( 'NONE', #9373, #11092, #10420, .T. ) ;
#7438=LINE ( 'NONE', #12161, #1235 ) ;
#7439=VERTEX_POINT ( 'NONE', #12640 ) ;
#7440=CARTESIAN_POINT ( 'NONE',  ( 37.53686968382241673, 89.89283556784525331, -13.00000000000000178 ) ) ;
#7441=CYLINDRICAL_SURFACE ( 'NONE', #3718, 2.649999999999992806 ) ;
#7442=VERTEX_POINT ( 'NONE', #6855 ) ;
#7443=LINE ( 'NONE', #545, #7640 ) ;
#7445=ORIENTED_EDGE ( 'NONE', *, *, #13960, .T. ) ;
#7446=FACE_OUTER_BOUND ( 'NONE', #829, .T. ) ;
#7447=ORIENTED_EDGE ( 'NONE', *, *, #6698, .T. ) ;
#7450=DIRECTION ( 'NONE',  ( -1.000000000000000000, 0.000000000000000000, 0.000000000000000000 ) ) ;
#7451=CARTESIAN_POINT ( 'NONE',  ( -26.49999999999971578, -45.89934640057541060, -8.000000000000000000 ) ) ;
#7452=EDGE_CURVE ( 'NONE', #1677, #10590, #12368, .T. ) ;
#7454=CARTESIAN_POINT ( 'NONE',  ( 68.58935777509475429, -68.58935777509547904, -10.50000000000000000 ) ) ;
#7455=AXIS2_PLACEMENT_3D ( 'NONE', #8406, #4622, #53 ) ;
#7460=VERTEX_POINT ( 'NONE', #181 ) ;
#7464=CARTESIAN_POINT ( 'NONE',  ( -32.46576781417928714, 41.59008834022678514, -13.00000000000000178 ) ) ;
#7465=CARTESIAN_POINT ( 'NONE',  ( -33.48561063518626923, 47.21331623427104063, -10.50000000000000000 ) ) ;
#7466=DIRECTION ( 'NONE',  ( -1.000000000000000000, 8.705157806719979026E-14, 0.000000000000000000 ) ) ;
#7467=CARTESIAN_POINT ( 'NONE',  ( 55.00000000000000000, -6.735557395310442615E-15, -13.00000000000000178 ) ) ;
#7470=ORIENTED_EDGE ( 'NONE', *, *, #3100, .F. ) ;
#7471=ORIENTED_EDGE ( 'NONE', *, *, #7202, .T. ) ;
#7474=EDGE_CURVE ( 'NONE', #5656, #12871, #14010, .T. ) ;
#7476=ORIENTED_EDGE ( 'NONE', *, *, #12618, .F. ) ;
#7477=EDGE_CURVE ( 'NONE', #8423, #2406, #2661, .T. ) ;
#7479=DIRECTION ( 'NONE',  ( -0.000000000000000000, -0.000000000000000000, 1.000000000000000000 ) ) ;
#7480=EDGE_LOOP ( 'NONE', ( #168, #7792, #2190, #873 ) ) ;
#7481=DIRECTION ( 'NONE',  ( 1.000000000000000000, 0.000000000000000000, 0.000000000000000000 ) ) ;
#7482=ADVANCED_FACE ( 'NONE', ( #1328 ), #7074, .T. ) ;
#7484=CARTESIAN_POINT ( 'NONE',  ( 45.89934640057532533, -26.49999999999987566, -13.00000000000000178 ) ) ;
#7487=CARTESIAN_POINT ( 'NONE',  ( -97.00000000000000000, 1.015776140243522349E-12, -10.50000000000000000 ) ) ;
#7488=EDGE_CURVE ( 'NONE', #13059, #9534, #3456, .T. ) ;
#7489=EDGE_CURVE ( 'NONE', #5951, #14678, #12404, .T. ) ;
#7490=ORIENTED_EDGE ( 'NONE', *, *, #9493, .F. ) ;
#7492=CARTESIAN_POINT ( 'NONE',  ( 53.26842454702428142, 11.55014193876197126, 8.000000000000000000 ) ) ;
#7493=VECTOR ( 'NONE', #11701, 1000.000000000000000 ) ;
#7494=VECTOR ( 'NONE', #2590, 1000.000000000000000 ) ;
#7495=CARTESIAN_POINT ( 'NONE',  ( -37.12029293941441210, -89.61631465359452875, -8.000000000000000000 ) ) ;
#7496=ADVANCED_FACE ( 'NONE', ( #3681 ), #8302, .F. ) ;
#7497=CARTESIAN_POINT ( 'NONE',  ( 0.000000000000000000, 0.000000000000000000, -10.50000000000000000 ) ) ;
#7498=DIRECTION ( 'NONE',  ( -0.000000000000000000, -0.000000000000000000, -1.000000000000000000 ) ) ;
#7499=DIRECTION ( 'NONE',  ( -1.000000000000000000, 0.000000000000000000, 0.000000000000000000 ) ) ;
#7500=AXIS2_PLACEMENT_3D ( 'NONE', #13239, #5035, #2834 ) ;
#7501=DIRECTION ( 'NONE',  ( 0.000000000000000000, 0.000000000000000000, 1.000000000000000000 ) ) ;
#7502=VERTEX_POINT ( 'NONE', #11809 ) ;
#7503=AXIS2_PLACEMENT_3D ( 'NONE', #13710, #6476, #12568 ) ;
#7504=AXIS2_PLACEMENT_3D ( 'NONE', #3209, #3067, #6685 ) ;
#7506=DIRECTION ( 'NONE',  ( 0.000000000000000000, 0.000000000000000000, 1.000000000000000000 ) ) ;
#7507=FACE_OUTER_BOUND ( 'NONE', #12063, .T. ) ;
#7508=DIRECTION ( 'NONE',  ( 1.000000000000000000, 0.000000000000000000, 0.000000000000000000 ) ) ;
#7511=CIRCLE ( 'NONE', #9458, 3.000000000000002665 ) ;
#7512=DIRECTION ( 'NONE',  ( 1.000000000000000000, 0.000000000000000000, 0.000000000000000000 ) ) ;
#7513=VERTEX_POINT ( 'NONE', #1471 ) ;
#7514=CARTESIAN_POINT ( 'NONE',  ( 39.30189486418243661, 33.47282819776626894, -13.00000000000000178 ) ) ;
#7515=AXIS2_PLACEMENT_3D ( 'NONE', #2815, #7433, #1673 ) ;
#7516=VERTEX_POINT ( 'NONE', #8668 ) ;
#7518=CARTESIAN_POINT ( 'NONE',  ( 0.000000000000000000, 0.000000000000000000, 13.00000000000000178 ) ) ;
#7519=FACE_OUTER_BOUND ( 'NONE', #4114, .T. ) ;
#7521=DIRECTION ( 'NONE',  ( 0.000000000000000000, 0.000000000000000000, -1.000000000000000000 ) ) ;
#7523=VECTOR ( 'NONE', #8192, 1000.000000000000000 ) ;
#7525=CIRCLE ( 'NONE', #510, 0.5000000000000022204 ) ;
#7526=ORIENTED_EDGE ( 'NONE', *, *, #6547, .T. ) ;
#7527=CARTESIAN_POINT ( 'NONE',  ( 24.98583958711424202, -30.74264578624780597, -28.00000000000000000 ) ) ;
#7529=CARTESIAN_POINT ( 'NONE',  ( 0.000000000000000000, 0.000000000000000000, 10.50000000000000000 ) ) ;
#7530=VECTOR ( 'NONE', #11922, 1000.000000000000000 ) ;
#7531=DIRECTION ( 'NONE',  ( -0.000000000000000000, -0.000000000000000000, -1.000000000000000000 ) ) ;
#7532=EDGE_CURVE ( 'NONE', #5235, #1639, #3162, .T. ) ;
#7534=EDGE_CURVE ( 'NONE', #3488, #1441, #2420, .T. ) ;
#7536=EDGE_CURVE ( 'NONE', #11040, #11081, #3906, .T. ) ;
#7538=DIRECTION ( 'NONE',  ( 0.000000000000000000, 0.000000000000000000, -1.000000000000000000 ) ) ;
#7540=CIRCLE ( 'NONE', #30, 3.000000000000002665 ) ;
#7541=CARTESIAN_POINT ( 'NONE',  ( 39.61975340586557337, 91.27544013909754028, -13.00000000000000178 ) ) ;
#7542=FACE_OUTER_BOUND ( 'NONE', #14700, .T. ) ;
#7543=ORIENTED_EDGE ( 'NONE', *, *, #10150, .F. ) ;
#7545=AXIS2_PLACEMENT_3D ( 'NONE', #14994, #9502, #4585 ) ;
#7546=CYLINDRICAL_SURFACE ( 'NONE', #828, 63.00000000000000000 ) ;
#7547=ORIENTED_EDGE ( 'NONE', *, *, #9820, .T. ) ;
#7548=EDGE_CURVE ( 'NONE', #14306, #13178, #484, .T. ) ;
#7549=ORIENTED_EDGE ( 'NONE', *, *, #12075, .T. ) ;
#7551=DIRECTION ( 'NONE',  ( 0.000000000000000000, 0.000000000000000000, 1.000000000000000000 ) ) ;
#7553=AXIS2_PLACEMENT_3D ( 'NONE', #13995, #2366, #12780 ) ;
#7554=EDGE_CURVE ( 'NONE', #13671, #9453, #5579, .T. ) ;
#7555=PLANE ( 'NONE',  #10991 ) ;
#7556=EDGE_LOOP ( 'NONE', ( #11587, #10867, #12655, #2183 ) ) ;
#7557=CIRCLE ( 'NONE', #1036, 100.0000000000000000 ) ;
#7558=ORIENTED_EDGE ( 'NONE', *, *, #4433, .T. ) ;
#7560=EDGE_CURVE ( 'NONE', #7767, #8421, #9243, .T. ) ;
#7561=ORIENTED_EDGE ( 'NONE', *, *, #3289, .F. ) ;
#7562=CARTESIAN_POINT ( 'NONE',  ( -22.33583958711380646, -30.74264578624812927, -25.50000000000000355 ) ) ;
#7563=CIRCLE ( 'NONE', #1275, 100.0000000000000000 ) ;
#7564=DIRECTION ( 'NONE',  ( 1.000000000000000000, 0.000000000000000000, -0.000000000000000000 ) ) ;
#7565=( NAMED_UNIT ( * ) SI_UNIT ( $, .STERADIAN. ) SOLID_ANGLE_UNIT ( ) );
#7566=ORIENTED_EDGE ( 'NONE', *, *, #9353, .T. ) ;
#7568=DIRECTION ( 'NONE',  ( 1.000000000000000000, 0.000000000000000000, 0.000000000000000000 ) ) ;
#7569=AXIS2_PLACEMENT_3D ( 'NONE', #9723, #251, #2837 ) ;
#7572=ORIENTED_EDGE ( 'NONE', *, *, #14960, .T. ) ;
#7573=CIRCLE ( 'NONE', #2742, 59.50000000000000000 ) ;
#7577=LINE ( 'NONE', #5392, #7266 ) ;
#7578=EDGE_CURVE ( 'NONE', #6497, #13693, #2702, .T. ) ;
#7580=EDGE_CURVE ( 'NONE', #3803, #11690, #13134, .T. ) ;
#7581=DIRECTION ( 'NONE',  ( 1.000000000000000000, 0.000000000000000000, -0.000000000000000000 ) ) ;
#7582=DIRECTION ( 'NONE',  ( 0.000000000000000000, 0.000000000000000000, 1.000000000000000000 ) ) ;
#7583=DIRECTION ( 'NONE',  ( 0.000000000000000000, 0.000000000000000000, 1.000000000000000000 ) ) ;
#7585=EDGE_CURVE ( 'NONE', #3464, #5876, #8512, .T. ) ;
#7586=AXIS2_PLACEMENT_3D ( 'NONE', #12382, #9384, #1977 ) ;
#7588=DIRECTION ( 'NONE',  ( 0.000000000000000000, 0.000000000000000000, -1.000000000000000000 ) ) ;
#7592=DIRECTION ( 'NONE',  ( 0.000000000000000000, 0.000000000000000000, 1.000000000000000000 ) ) ;
#7593=CIRCLE ( 'NONE', #3968, 52.50000000000000711 ) ;
#7594=ORIENTED_EDGE ( 'NONE', *, *, #11866, .T. ) ;
#7597=DIRECTION ( 'NONE',  ( -0.000000000000000000, -0.000000000000000000, 1.000000000000000000 ) ) ;
#7601=EDGE_CURVE ( 'NONE', #11178, #6334, #2914, .T. ) ;
#7604=PLANE ( 'NONE',  #6788 ) ;
#7605=CARTESIAN_POINT ( 'NONE',  ( -97.00000000000000000, 1.015776140243522349E-12, 8.000000000000000000 ) ) ;
#7607=CIRCLE ( 'NONE', #10766, 59.50000000000000000 ) ;
#7608=DIRECTION ( 'NONE',  ( -1.000000000000000000, 0.000000000000000000, 0.000000000000000000 ) ) ;
#7609=CARTESIAN_POINT ( 'NONE',  ( 49.11971303961677648, 15.88467684210564990, -8.000000000000000000 ) ) ;
#7611=VERTEX_POINT ( 'NONE', #13090 ) ;
#7612=CARTESIAN_POINT ( 'NONE',  ( 89.61631465359491244, 37.12029293941346708, 10.49999999999999822 ) ) ;
#7616=CIRCLE ( 'NONE', #14908, 60.50000000000000000 ) ;
#7618=ORIENTED_EDGE ( 'NONE', *, *, #13919, .F. ) ;
#7619=DIRECTION ( 'NONE',  ( -0.000000000000000000, -0.000000000000000000, -1.000000000000000000 ) ) ;
#7620=ORIENTED_EDGE ( 'NONE', *, *, #12764, .T. ) ;
#7621=CARTESIAN_POINT ( 'NONE',  ( 0.000000000000000000, 0.000000000000000000, -8.000000000000000000 ) ) ;
#7624=AXIS2_PLACEMENT_3D ( 'NONE', #10195, #7479, #14842 ) ;
#7626=DIRECTION ( 'NONE',  ( -1.000000000000000000, 0.000000000000000000, 0.000000000000000000 ) ) ;
#7631=AXIS2_PLACEMENT_3D ( 'NONE', #12395, #14684, #4508 ) ;
#7632=ORIENTED_EDGE ( 'NONE', *, *, #7255, .F. ) ;
#7633=ORIENTED_EDGE ( 'NONE', *, *, #8552, .T. ) ;
#7634=EDGE_CURVE ( 'NONE', #11672, #1517, #1550, .T. ) ;
#7635=FACE_OUTER_BOUND ( 'NONE', #9224, .T. ) ;
#7637=EDGE_CURVE ( 'NONE', #1115, #11359, #2679, .T. ) ;
#7640=VECTOR ( 'NONE', #12092, 1000.000000000000000 ) ;
#7642=AXIS2_PLACEMENT_3D ( 'NONE', #7309, #11966, #481 ) ;
#7643=AXIS2_PLACEMENT_3D ( 'NONE', #5610, #2122, #8800 ) ;
#7644=ORIENTED_EDGE ( 'NONE', *, *, #10927, .F. ) ;
#7646=DIRECTION ( 'NONE',  ( -0.000000000000000000, -0.000000000000000000, -1.000000000000000000 ) ) ;
#7648=EDGE_CURVE ( 'NONE', #1076, #9534, #7267, .T. ) ;
#7649=LINE ( 'NONE', #3249, #14966 ) ;
#7650=AXIS2_PLACEMENT_3D ( 'NONE', #6322, #13410, #9833 ) ;
#7652=FACE_BOUND ( 'NONE', #12935, .T. ) ;
#7654=ORIENTED_EDGE ( 'NONE', *, *, #9057, .T. ) ;
#7655=ADVANCED_FACE ( 'NONE', ( #1911 ), #12551, .T. ) ;
#7656=EDGE_CURVE ( 'NONE', #12197, #8810, #14563, .T. ) ;
#7657=CARTESIAN_POINT ( 'NONE',  ( -65.64523757230321621, -68.01302780753330524, -13.00000000000000178 ) ) ;
#7658=ORIENTED_EDGE ( 'NONE', *, *, #3011, .F. ) ;
#7661=AXIS2_PLACEMENT_3D ( 'NONE', #8452, #3610, #11965 ) ;
#7662=DIRECTION ( 'NONE',  ( 0.000000000000000000, 0.000000000000000000, -1.000000000000000000 ) ) ;
#7663=CARTESIAN_POINT ( 'NONE',  ( 0.000000000000000000, 0.000000000000000000, -8.000000000000000000 ) ) ;
#7665=PLANE ( 'NONE',  #14527 ) ;
#7666=ORIENTED_EDGE ( 'NONE', *, *, #13061, .T. ) ;
#7667=AXIS2_PLACEMENT_3D ( 'NONE', #5563, #3521, #4516 ) ;
#7668=CARTESIAN_POINT ( 'NONE',  ( 0.000000000000000000, 0.000000000000000000, -10.50000000000000000 ) ) ;
#7670=EDGE_CURVE ( 'NONE', #12050, #7980, #13839, .T. ) ;
#7672=EDGE_CURVE ( 'NONE', #7167, #13653, #13340, .T. ) ;
#7673=ADVANCED_FACE ( 'NONE', ( #14524 ), #788, .F. ) ;
#7676=ADVANCED_FACE ( 'NONE', ( #4125 ), #4289, .T. ) ;
#7677=ORIENTED_EDGE ( 'NONE', *, *, #1188, .T. ) ;
#7678=VECTOR ( 'NONE', #1614, 1000.000000000000000 ) ;
#7679=CARTESIAN_POINT ( 'NONE',  ( 68.58935777509523746, 68.58935777509499587, -13.00000000000000178 ) ) ;
#7681=ORIENTED_EDGE ( 'NONE', *, *, #8905, .F. ) ;
#7682=DIRECTION ( 'NONE',  ( 0.000000000000000000, 0.000000000000000000, 1.000000000000000000 ) ) ;
#7684=CARTESIAN_POINT ( 'NONE',  ( 52.72775723226780542, -7.383907457637739036, -13.00000000000000178 ) ) ;
#7685=ADVANCED_FACE ( 'NONE', ( #13530 ), #13384, .F. ) ;
#7686=DIRECTION ( 'NONE',  ( -0.000000000000000000, -0.000000000000000000, -1.000000000000000000 ) ) ;
#7687=DIRECTION ( 'NONE',  ( -1.000000000000000000, 0.000000000000000000, 0.000000000000000000 ) ) ;
#7689=PLANE ( 'NONE',  #6199 ) ;
#7691=ADVANCED_FACE ( 'NONE', ( #3134 ), #10184, .T. ) ;
#7692=EDGE_CURVE ( 'NONE', #9024, #8856, #12398, .T. ) ;
#7693=DIRECTION ( 'NONE',  ( 0.000000000000000000, 0.000000000000000000, 1.000000000000000000 ) ) ;
#7694=ORIENTED_EDGE ( 'NONE', *, *, #8614, .T. ) ;
#7696=ORIENTED_EDGE ( 'NONE', *, *, #14556, .T. ) ;
#7697=FACE_OUTER_BOUND ( 'NONE', #1790, .T. ) ;
#7700=DIRECTION ( 'NONE',  ( -0.000000000000000000, -0.000000000000000000, 1.000000000000000000 ) ) ;
#7705=LINE ( 'NONE', #734, #11553 ) ;
#7709=ORIENTED_EDGE ( 'NONE', *, *, #7112, .T. ) ;
#7711=DIRECTION ( 'NONE',  ( 0.000000000000000000, 0.000000000000000000, 1.000000000000000000 ) ) ;
#7712=DIRECTION ( 'NONE',  ( -0.000000000000000000, -0.000000000000000000, 1.000000000000000000 ) ) ;
#7714=CARTESIAN_POINT ( 'NONE',  ( -68.01302780753309207, 65.64523757230344359, 8.000000000000000000 ) ) ;
#7716=CARTESIAN_POINT ( 'NONE',  ( 37.12029293941315444, -89.61631465359504034, -13.00000000000000178 ) ) ;
#7720=VERTEX_POINT ( 'NONE', #12257 ) ;
#7724=EDGE_CURVE ( 'NONE', #13551, #14933, #9426, .T. ) ;
#7725=ADVANCED_FACE ( 'NONE', ( #869 ), #5491, .T. ) ;
#7727=AXIS2_PLACEMENT_3D ( 'NONE', #2663, #4951, #9780 ) ;
#7730=CARTESIAN_POINT ( 'NONE',  ( 96.58511096861892042, 0.2790467552928839190, 10.49999999999999822 ) ) ;
#7731=EDGE_CURVE ( 'NONE', #2566, #6431, #5560, .T. ) ;
#7733=ORIENTED_EDGE ( 'NONE', *, *, #9718, .T. ) ;
#7735=DIRECTION ( 'NONE',  ( 0.000000000000000000, 0.000000000000000000, 1.000000000000000000 ) ) ;
#7737=AXIS2_PLACEMENT_3D ( 'NONE', #14265, #10916, #8266 ) ;
#7739=EDGE_LOOP ( 'NONE', ( #10108, #1943, #13311, #8867, #1532, #2112, #2841 ) ) ;
#7741=ORIENTED_EDGE ( 'NONE', *, *, #12480, .T. ) ;
#7743=ORIENTED_EDGE ( 'NONE', *, *, #13925, .T. ) ;
#7747=DIRECTION ( 'NONE',  ( -0.000000000000000000, -0.000000000000000000, 1.000000000000000000 ) ) ;
#7748=AXIS2_PLACEMENT_3D ( 'NONE', #10206, #14850, #3372 ) ;
#7752=DIRECTION ( 'NONE',  ( 1.000000000000000000, 0.000000000000000000, 0.000000000000000000 ) ) ;
#7753=EDGE_CURVE ( 'NONE', #11882, #2381, #3288, .T. ) ;
#7755=DIRECTION ( 'NONE',  ( 0.000000000000000000, 0.000000000000000000, 1.000000000000000000 ) ) ;
#7756=EDGE_LOOP ( 'NONE', ( #14126, #8694, #14496, #2013, #2709 ) ) ;
#7758=ORIENTED_EDGE ( 'NONE', *, *, #7417, .F. ) ;
#7762=CYLINDRICAL_SURFACE ( 'NONE', #1768, 63.00000000000000000 ) ;
#7763=AXIS2_PLACEMENT_3D ( 'NONE', #2105, #13286, #14945 ) ;
#7764=ORIENTED_EDGE ( 'NONE', *, *, #6657, .F. ) ;
#7765=CARTESIAN_POINT ( 'NONE',  ( 9.706953719245472456, 57.06275842387054098, -13.00000000000000178 ) ) ;
#7767=VERTEX_POINT ( 'NONE', #11414 ) ;
#7768=DIRECTION ( 'NONE',  ( 0.000000000000000000, 0.000000000000000000, 1.000000000000000000 ) ) ;
#7770=CARTESIAN_POINT ( 'NONE',  ( 37.12029293941379393, 89.61631465359479876, 10.49999999999999822 ) ) ;
#7771=CARTESIAN_POINT ( 'NONE',  ( 12.86891638962116247, -56.43380494354001087, -8.000000000000000000 ) ) ;
#7772=CIRCLE ( 'NONE', #13117, 3.000000000000002665 ) ;
#7775=FACE_OUTER_BOUND ( 'NONE', #375, .T. ) ;
#7776=ADVANCED_FACE ( 'NONE', ( #5928 ), #7055, .F. ) ;
#7777=DIRECTION ( 'NONE',  ( 0.000000000000000000, 0.000000000000000000, 1.000000000000000000 ) ) ;
#7780=AXIS2_PLACEMENT_3D ( 'NONE', #7401, #10823, #3845 ) ;
#7782=EDGE_LOOP ( 'NONE', ( #3181, #10859, #8472, #2808, #1256, #9013, #10232 ) ) ;
#7783=VECTOR ( 'NONE', #4323, 1000.000000000000000 ) ;
#7784=CARTESIAN_POINT ( 'NONE',  ( -100.0000000000000000, 0.000000000000000000, 13.00000000000000178 ) ) ;
#7786=DIRECTION ( 'NONE',  ( -1.000000000000000000, 0.000000000000000000, 0.000000000000000000 ) ) ;
#7787=EDGE_LOOP ( 'NONE', ( #6257, #3937, #3765, #4402, #14995 ) ) ;
#7788=ADVANCED_FACE ( 'NONE', ( #6915 ), #10565, .T. ) ;
#7789=CIRCLE ( 'NONE', #1251, 3.000000000000002665 ) ;
#7790=ORIENTED_EDGE ( 'NONE', *, *, #4764, .F. ) ;
#7791=AXIS2_PLACEMENT_3D ( 'NONE', #2455, #8221, #6013 ) ;
#7792=ORIENTED_EDGE ( 'NONE', *, *, #3721, .T. ) ;
#7794=EDGE_CURVE ( 'NONE', #8824, #13003, #12352, .T. ) ;
#7795=CARTESIAN_POINT ( 'NONE',  ( 37.12029293941315444, -89.61631465359504034, -8.000000000000000000 ) ) ;
#7796=DIRECTION ( 'NONE',  ( -1.000000000000000000, 0.000000000000000000, 0.000000000000000000 ) ) ;
#7797=ORIENTED_EDGE ( 'NONE', *, *, #15003, .T. ) ;
#7798=FACE_BOUND ( 'NONE', #4292, .T. ) ;
#7801=ORIENTED_EDGE ( 'NONE', *, *, #4865, .T. ) ;
#7802=EDGE_LOOP ( 'NONE', ( #14444, #8583, #6027, #8749 ) ) ;
#7804=DIRECTION ( 'NONE',  ( 1.000000000000000000, 0.000000000000000000, 0.000000000000000000 ) ) ;
#7805=DIRECTION ( 'NONE',  ( 1.000000000000000000, 0.000000000000000000, 0.000000000000000000 ) ) ;
#7806=CARTESIAN_POINT ( 'NONE',  ( 0.000000000000000000, 0.000000000000000000, -8.000000000000000000 ) ) ;
#7807=AXIS2_PLACEMENT_3D ( 'NONE', #8448, #1470, #2685 ) ;
#7808=DIRECTION ( 'NONE',  ( 0.000000000000000000, 0.000000000000000000, 1.000000000000000000 ) ) ;
#7810=CARTESIAN_POINT ( 'NONE',  ( -45.89934640057513349, 26.50000000000019540, 8.000000000000000000 ) ) ;
#7813=CIRCLE ( 'NONE', #5630, 3.000000000000002665 ) ;
#7816=CYLINDRICAL_SURFACE ( 'NONE', #14815, 3.000000000000002665 ) ;
#7818=ORIENTED_EDGE ( 'NONE', *, *, #7023, .F. ) ;
#7822=ORIENTED_EDGE ( 'NONE', *, *, #172, .F. ) ;
#7823=ADVANCED_BREP_SHAPE_REPRESENTATION ( '', ( #4169, #5108 ), #6780 ) ;
#7824=FACE_OUTER_BOUND ( 'NONE', #3856, .T. ) ;
#7825=CIRCLE ( 'NONE', #11235, 0.5000000000000004441 ) ;
#7829=DIRECTION ( 'NONE',  ( -1.000000000000000000, 0.000000000000000000, 0.000000000000000000 ) ) ;
#7831=ADVANCED_FACE ( 'NONE', ( #12623 ), #5709, .T. ) ;
#7837=VECTOR ( 'NONE', #361, 1000.000000000000000 ) ;
#7838=CARTESIAN_POINT ( 'NONE',  ( 49.00442420935993226, -30.80502811811213704, -10.50000000000000000 ) ) ;
#7840=ORIENTED_EDGE ( 'NONE', *, *, #14012, .T. ) ;
#7841=VECTOR ( 'NONE', #2148, 1000.000000000000000 ) ;
#7843=ORIENTED_EDGE ( 'NONE', *, *, #10812, .T. ) ;
#7845=CARTESIAN_POINT ( 'NONE',  ( 0.000000000000000000, 0.000000000000000000, -8.000000000000000000 ) ) ;
#7846=ORIENTED_EDGE ( 'NONE', *, *, #880, .F. ) ;
#7848=DIRECTION ( 'NONE',  ( -0.000000000000000000, -0.000000000000000000, -1.000000000000000000 ) ) ;
#7850=EDGE_LOOP ( 'NONE', ( #4192, #14484, #2612, #13911 ) ) ;
#7853=DIRECTION ( 'NONE',  ( -1.000000000000000000, 0.000000000000000000, 0.000000000000000000 ) ) ;
#7854=CARTESIAN_POINT ( 'NONE',  ( 9.706953719245472456, 57.06275842387054098, 10.49999999999999822 ) ) ;
#7855=AXIS2_PLACEMENT_3D ( 'NONE', #11537, #9299, #6717 ) ;
#7856=DIRECTION ( 'NONE',  ( 0.000000000000000000, 0.000000000000000000, -1.000000000000000000 ) ) ;
#7857=EDGE_LOOP ( 'NONE', ( #3408, #13954, #5438, #4607 ) ) ;
#7858=EDGE_CURVE ( 'NONE', #5275, #6515, #4651, .T. ) ;
#7860=EDGE_LOOP ( 'NONE', ( #8541, #14477, #901, #3872, #414, #8624, #13741, #13585 ) ) ;
#7861=CIRCLE ( 'NONE', #7127, 3.000000000000002665 ) ;
#7862=EDGE_LOOP ( 'NONE', ( #12689, #848, #2289, #4720 ) ) ;
#7863=AXIS2_PLACEMENT_3D ( 'NONE', #4477, #5890, #3329 ) ;
#7867=CARTESIAN_POINT ( 'NONE',  ( 42.04772703543530099, 32.26435573746242369, -8.000000000000000000 ) ) ;
#7868=DIRECTION ( 'NONE',  ( 0.000000000000000000, 0.000000000000000000, 1.000000000000000000 ) ) ;
#7870=DIRECTION ( 'NONE',  ( 1.000000000000000000, 0.000000000000000000, 0.000000000000000000 ) ) ;
#7872=ORIENTED_EDGE ( 'NONE', *, *, #9032, .F. ) ;
#7873=CARTESIAN_POINT ( 'NONE',  ( 46.33974596215558961, -6.205269775947987555E-15, -28.00000000000000000 ) ) ;
#7876=VERTEX_POINT ( 'NONE', #8060 ) ;
#7877=CARTESIAN_POINT ( 'NONE',  ( 0.000000000000000000, 0.000000000000000000, -8.000000000000000000 ) ) ;
#7878=AXIS2_PLACEMENT_3D ( 'NONE', #4345, #8049, #1156 ) ;
#7879=AXIS2_PLACEMENT_3D ( 'NONE', #7621, #6544, #9979 ) ;
#7881=AXIS2_PLACEMENT_3D ( 'NONE', #9957, #14606, #13460 ) ;
#7882=EDGE_CURVE ( 'NONE', #6432, #4604, #12698, .T. ) ;
#7883=EDGE_LOOP ( 'NONE', ( #1505, #6473, #13195, #10433, #3328 ) ) ;
#7884=DIRECTION ( 'NONE',  ( 0.000000000000000000, 0.000000000000000000, 1.000000000000000000 ) ) ;
#7887=DIRECTION ( 'NONE',  ( -0.000000000000000000, -0.000000000000000000, 1.000000000000000000 ) ) ;
#7889=DIRECTION ( 'NONE',  ( 0.000000000000000000, 0.000000000000000000, 1.000000000000000000 ) ) ;
#7891=DIRECTION ( 'NONE',  ( 1.000000000000000000, 0.000000000000000000, -0.000000000000000000 ) ) ;
#7892=ORIENTED_EDGE ( 'NONE', *, *, #7474, .F. ) ;
#7893=DIRECTION ( 'NONE',  ( -1.000000000000000000, 0.000000000000000000, 0.000000000000000000 ) ) ;
#7895=CIRCLE ( 'NONE', #10807, 3.000000000000002665 ) ;
#7896=CARTESIAN_POINT ( 'NONE',  ( -11.55014193876141526, 53.26842454702440222, -8.000000000000000000 ) ) ;
#7897=DIRECTION ( 'NONE',  ( -0.000000000000000000, -0.000000000000000000, -1.000000000000000000 ) ) ;
#7898=AXIS2_PLACEMENT_3D ( 'NONE', #3793, #57, #10606 ) ;
#7899=ORIENTED_EDGE ( 'NONE', *, *, #11022, .T. ) ;
#7901=ORIENTED_EDGE ( 'NONE', *, *, #3663, .F. ) ;
#7902=CYLINDRICAL_SURFACE ( 'NONE', #5449, 56.99999999999999289 ) ;
#7904=CARTESIAN_POINT ( 'NONE',  ( -36.14014761921588104, 11.74264578624790190, -28.00000000000000000 ) ) ;
#7906=ADVANCED_FACE ( 'NONE', ( #7208 ), #14278, .T. ) ;
#7909=CARTESIAN_POINT ( 'NONE',  ( 91.27544013909738396, -39.61975340586589311, -13.00000000000000178 ) ) ;
#7912=VERTEX_POINT ( 'NONE', #14352 ) ;
#7913=CARTESIAN_POINT ( 'NONE',  ( 0.000000000000000000, 0.000000000000000000, -10.50000000000000000 ) ) ;
#7914=DIRECTION ( 'NONE',  ( 0.000000000000000000, 0.000000000000000000, 1.000000000000000000 ) ) ;
#7916=AXIS2_PLACEMENT_3D ( 'NONE', #13371, #10023, #13515 ) ;
#7917=PRODUCT ( 'brake disk', 'brake disk', '', ( #4306 ) ) ;
#7918=DIRECTION ( 'NONE',  ( 0.000000000000000000, 0.000000000000000000, -1.000000000000000000 ) ) ;
#7919=VERTEX_POINT ( 'NONE', #7282 ) ;
#7921=VERTEX_POINT ( 'NONE', #6217 ) ;
#7922=EDGE_CURVE ( 'NONE', #11359, #1631, #9658, .T. ) ;
#7923=CARTESIAN_POINT ( 'NONE',  ( 33.29654390035847911, -41.94820822869180432, -10.50000000000000000 ) ) ;
#7926=EDGE_CURVE ( 'NONE', #10396, #9550, #14133, .T. ) ;
#7929=VERTEX_POINT ( 'NONE', #6069 ) ;
#7931=ORIENTED_EDGE ( 'NONE', *, *, #1813, .F. ) ;
#7932=DIRECTION ( 'NONE',  ( 0.000000000000000000, 0.000000000000000000, 1.000000000000000000 ) ) ;
#7933=LINE ( 'NONE', #13634, #6380 ) ;
#7934=CYLINDRICAL_SURFACE ( 'NONE', #5149, 59.50000000000000000 ) ;
#7935=ORIENTED_EDGE ( 'NONE', *, *, #5175, .T. ) ;
#7937=ORIENTED_EDGE ( 'NONE', *, *, #2480, .F. ) ;
#7938=CIRCLE ( 'NONE', #11102, 50.00000000000000000 ) ;
#7941=CYLINDRICAL_SURFACE ( 'NONE', #12691, 50.00000000000000000 ) ;
#7944=ADVANCED_FACE ( 'NONE', ( #13226 ), #5027, .T. ) ;
#7947=DIRECTION ( 'NONE',  ( 0.000000000000000000, 0.000000000000000000, 1.000000000000000000 ) ) ;
#7948=CIRCLE ( 'NONE', #6486, 3.000000000000002665 ) ;
#7950=ORIENTED_EDGE ( 'NONE', *, *, #14014, .F. ) ;
#7952=DIRECTION ( 'NONE',  ( 0.000000000000000000, 0.000000000000000000, -1.000000000000000000 ) ) ;
#7954=LINE ( 'NONE', #14883, #2936 ) ;
#7955=CARTESIAN_POINT ( 'NONE',  ( -13.71740939043329277, 51.19406879332069593, -8.000000000000000000 ) ) ;
#7956=PLANE ( 'NONE',  #7145 ) ;
#7958=EDGE_CURVE ( 'NONE', #2090, #14329, #13076, .T. ) ;
#7960=EDGE_CURVE ( 'NONE', #4919, #4753, #965, .T. ) ;
#7962=LINE ( 'NONE', #12604, #6074 ) ;
#7964=DIRECTION ( 'NONE',  ( 0.000000000000000000, 0.000000000000000000, -1.000000000000000000 ) ) ;
#7967=DIRECTION ( 'NONE',  ( 0.000000000000000000, 0.000000000000000000, 1.000000000000000000 ) ) ;
#7969=AXIS2_PLACEMENT_3D ( 'NONE', #5994, #10713, #13147 ) ;
#7971=ORIENTED_EDGE ( 'NONE', *, *, #12768, .F. ) ;
#7973=CARTESIAN_POINT ( 'NONE',  ( 71.58935777509475429, -68.58935777509547904, -8.000000000000000000 ) ) ;
#7974=DIRECTION ( 'NONE',  ( 1.000000000000000000, 0.000000000000000000, 0.000000000000000000 ) ) ;
#7975=DIRECTION ( 'NONE',  ( 1.000000000000000000, 0.000000000000000000, -0.000000000000000000 ) ) ;
#7978=AXIS2_PLACEMENT_3D ( 'NONE', #6670, #11324, #924 ) ;
#7979=CARTESIAN_POINT ( 'NONE',  ( -6.451868917687557214, -52.36539807335606156, 10.49999999999999822 ) ) ;
#7980=VERTEX_POINT ( 'NONE', #10858 ) ;
#7983=CARTESIAN_POINT ( 'NONE',  ( -56.43380494354004639, -12.86891638962099549, -13.00000000000000178 ) ) ;
#7985=AXIS2_PLACEMENT_3D ( 'NONE', #14417, #14341, #6207 ) ;
#7986=DIRECTION ( 'NONE',  ( 1.000000000000000000, 0.000000000000000000, 0.000000000000000000 ) ) ;
#7987=EDGE_LOOP ( 'NONE', ( #10714, #2438, #5129, #8586, #12253 ) ) ;
#7990=ORIENTED_EDGE ( 'NONE', *, *, #3710, .T. ) ;
#7991=AXIS2_PLACEMENT_3D ( 'NONE', #5086, #2512, #12083 ) ;
#7993=DIRECTION ( 'NONE',  ( 0.000000000000000000, 0.000000000000000000, 1.000000000000000000 ) ) ;
#7994=CARTESIAN_POINT ( 'NONE',  ( -56.43380494354004639, -12.86891638962099549, 8.000000000000000000 ) ) ;
#7995=DIRECTION ( 'NONE',  ( 1.000000000000000000, 0.000000000000000000, 0.000000000000000000 ) ) ;
#7996=ORIENTED_EDGE ( 'NONE', *, *, #62, .F. ) ;
#7997=ORIENTED_EDGE ( 'NONE', *, *, #14663, .F. ) ;
#7998=VERTEX_POINT ( 'NONE', #13070 ) ;
#7999=ORIENTED_EDGE ( 'NONE', *, *, #4087, .F. ) ;
#8000=AXIS2_PLACEMENT_3D ( 'NONE', #708, #8743, #8896 ) ;
#8003=CIRCLE ( 'NONE', #9941, 56.99999999999999289 ) ;
#8005=AXIS2_PLACEMENT_3D ( 'NONE', #4560, #4709, #10395 ) ;
#8008=EDGE_CURVE ( 'NONE', #6463, #13160, #11389, .T. ) ;
#8009=ADVANCED_FACE ( 'NONE', ( #6143 ), #10630, .T. ) ;
#8010=ORIENTED_EDGE ( 'NONE', *, *, #12667, .F. ) ;
#8011=ORIENTED_EDGE ( 'NONE', *, *, #180, .F. ) ;
#8014=AXIS2_PLACEMENT_3D ( 'NONE', #1821, #6436, #11087 ) ;
#8015=DIRECTION ( 'NONE',  ( -0.000000000000000000, -0.000000000000000000, -1.000000000000000000 ) ) ;
#8016=EDGE_CURVE ( 'NONE', #1144, #10864, #8940, .T. ) ;
#8019=CIRCLE ( 'NONE', #13855, 53.55662432702593634 ) ;
#8023=DIRECTION ( 'NONE',  ( 0.000000000000000000, 0.000000000000000000, 1.000000000000000000 ) ) ;
#8025=EDGE_CURVE ( 'NONE', #4530, #9553, #12834, .T. ) ;
#8026=DIRECTION ( 'NONE',  ( 0.000000000000000000, 0.000000000000000000, -1.000000000000000000 ) ) ;
#8028=CIRCLE ( 'NONE', #1017, 0.5000000000000004441 ) ;
#8029=ADVANCED_FACE ( 'NONE', ( #621 ), #7665, .F. ) ;
#8030=VERTEX_POINT ( 'NONE', #11012 ) ;
#8031=AXIS2_PLACEMENT_3D ( 'NONE', #3778, #3470, #10374 ) ;
#8032=VERTEX_POINT ( 'NONE', #691 ) ;
#8033=CARTESIAN_POINT ( 'NONE',  ( -45.89934640057513349, 26.50000000000019540, 8.000000000000000000 ) ) ;
#8034=ORIENTED_EDGE ( 'NONE', *, *, #853, .F. ) ;
#8035=ORIENTED_EDGE ( 'NONE', *, *, #4462, .T. ) ;
#8037=CARTESIAN_POINT ( 'NONE',  ( 9.706953719245472456, 57.06275842387054098, -10.50000000000000000 ) ) ;
#8038=CIRCLE ( 'NONE', #1501, 53.55662432702593634 ) ;
#8041=ORIENTED_EDGE ( 'NONE', *, *, #8804, .F. ) ;
#8043=VECTOR ( 'NONE', #6703, 1000.000000000000000 ) ;
#8044=EDGE_LOOP ( 'NONE', ( #14776, #7566, #14413, #3387 ) ) ;
#8046=DIRECTION ( 'NONE',  ( 1.000000000000000000, 0.000000000000000000, -0.000000000000000000 ) ) ;
#8047=AXIS2_PLACEMENT_3D ( 'NONE', #2225, #6839, #1233 ) ;
#8048=ORIENTED_EDGE ( 'NONE', *, *, #13743, .T. ) ;
#8049=DIRECTION ( 'NONE',  ( -0.000000000000000000, -0.000000000000000000, -1.000000000000000000 ) ) ;
#8050=ORIENTED_EDGE ( 'NONE', *, *, #13125, .F. ) ;
#8052=CARTESIAN_POINT ( 'NONE',  ( -13.21740939043329099, 51.19406879332069593, 10.49999999999999822 ) ) ;
#8055=DIRECTION ( 'NONE',  ( 0.000000000000000000, 0.000000000000000000, 1.000000000000000000 ) ) ;
#8056=EDGE_CURVE ( 'NONE', #8030, #6492, #5307, .T. ) ;
#8057=PLANE ( 'NONE',  #10301 ) ;
#8060=CARTESIAN_POINT ( 'NONE',  ( 45.88839665196118744, -26.99988008862642630, -10.50000000000000000 ) ) ;
#8062=EDGE_CURVE ( 'NONE', #12788, #9888, #12377, .T. ) ;
#8063=DIRECTION ( 'NONE',  ( 0.000000000000000000, 0.000000000000000000, -1.000000000000000000 ) ) ;
#8064=EDGE_LOOP ( 'NONE', ( #2339, #959, #4671, #7822 ) ) ;
#8066=CYLINDRICAL_SURFACE ( 'NONE', #5018, 0.5000000000000004441 ) ;
#8067=CYLINDRICAL_SURFACE ( 'NONE', #12958, 3.000000000000004441 ) ;
#8068=DIRECTION ( 'NONE',  ( 0.000000000000000000, 0.000000000000000000, 1.000000000000000000 ) ) ;
#8069=DIRECTION ( 'NONE',  ( 0.000000000000000000, 0.000000000000000000, 1.000000000000000000 ) ) ;
#8070=EDGE_CURVE ( 'NONE', #9479, #7296, #2644, .T. ) ;
#8071=ORIENTED_EDGE ( 'NONE', *, *, #13833, .F. ) ;
#8072=DIRECTION ( 'NONE',  ( -1.000000000000000000, 0.000000000000000000, 0.000000000000000000 ) ) ;
#8073=VERTEX_POINT ( 'NONE', #1971 ) ;
#8076=LINE ( 'NONE', #3534, #13400 ) ;
#8077=CARTESIAN_POINT ( 'NONE',  ( 38.26834323650905390, 92.38795325112863566, 8.000000000000000000 ) ) ;
#8078=CARTESIAN_POINT ( 'NONE',  ( 12.86891638962116247, -56.43380494354001087, -8.000000000000000000 ) ) ;
#8079=ORIENTED_EDGE ( 'NONE', *, *, #2398, .F. ) ;
#8080=VECTOR ( 'NONE', #8328, 1000.000000000000000 ) ;
#8081=DIRECTION ( 'NONE',  ( 0.000000000000000000, 0.000000000000000000, 1.000000000000000000 ) ) ;
#8082=DIRECTION ( 'NONE',  ( 0.000000000000000000, 0.000000000000000000, 1.000000000000000000 ) ) ;
#8084=ORIENTED_EDGE ( 'NONE', *, *, #7958, .F. ) ;
#8085=VECTOR ( 'NONE', #4973, 1000.000000000000000 ) ;
#8086=ORIENTED_EDGE ( 'NONE', *, *, #3201, .F. ) ;
#8087=ORIENTED_EDGE ( 'NONE', *, *, #3838, .T. ) ;
#8089=CARTESIAN_POINT ( 'NONE',  ( 6.917888187663118416, 52.54657765281190507, 8.000000000000000000 ) ) ;
#8092=DIRECTION ( 'NONE',  ( -1.000000000000000000, 0.000000000000000000, 0.000000000000000000 ) ) ;
#8093=CIRCLE ( 'NONE', #3990, 0.5000000000000073275 ) ;
#8094=AXIS2_PLACEMENT_3D ( 'NONE', #10364, #4673, #12865 ) ;
#8095=CIRCLE ( 'NONE', #4023, 0.5000000000000043299 ) ;
#8096=EDGE_CURVE ( 'NONE', #6738, #11326, #12123, .T. ) ;
#8097=CIRCLE ( 'NONE', #8820, 2.649999999999985700 ) ;
#8098=CYLINDRICAL_SURFACE ( 'NONE', #2211, 100.0000000000000000 ) ;
#8100=SHAPE_REPRESENTATION ( 'brake disk', ( #5108 ), #6780 ) ;
#8101=DIRECTION ( 'NONE',  ( -1.000000000000000000, 0.000000000000000000, 0.000000000000000000 ) ) ;
#8102=CARTESIAN_POINT ( 'NONE',  ( 57.06275842387049835, -9.706953719245678514, 10.49999999999999822 ) ) ;
#8104=ORIENTED_EDGE ( 'NONE', *, *, #2820, .F. ) ;
#8105=ORIENTED_EDGE ( 'NONE', *, *, #5634, .T. ) ;
#8106=DIRECTION ( 'NONE',  ( 0.000000000000000000, 0.000000000000000000, -1.000000000000000000 ) ) ;
#8107=CIRCLE ( 'NONE', #1569, 63.00000000000000000 ) ;
#8111=CARTESIAN_POINT ( 'NONE',  ( 26.49999999999971578, 45.89934640057541060, -10.50000000000000000 ) ) ;
#8113=DIRECTION ( 'NONE',  ( 0.000000000000000000, 0.000000000000000000, 1.000000000000000000 ) ) ;
#8117=AXIS2_PLACEMENT_3D ( 'NONE', #3220, #8550, #1727 ) ;
#8118=CARTESIAN_POINT ( 'NONE',  ( 99.48933418828643482, -1.674280531759671620, -13.00000000000000178 ) ) ;
#8119=ORIENTED_EDGE ( 'NONE', *, *, #5535, .T. ) ;
#8120=CIRCLE ( 'NONE', #10058, 59.50000000000000000 ) ;
#8122=CARTESIAN_POINT ( 'NONE',  ( 53.20607447915237742, -6.117650515114167575, -10.50000000000000000 ) ) ;
#8123=VECTOR ( 'NONE', #9407, 1000.000000000000000 ) ;
#8124=CARTESIAN_POINT ( 'NONE',  ( 30.80502811811196295, 49.00442420936003174, -13.00000000000000178 ) ) ;
#8126=DIRECTION ( 'NONE',  ( 1.000000000000000000, 0.000000000000000000, 0.000000000000000000 ) ) ;
#8128=CIRCLE ( 'NONE', #2314, 0.5000000000000073275 ) ;
#8130=ORIENTED_EDGE ( 'NONE', *, *, #8485, .F. ) ;
#8135=FACE_OUTER_BOUND ( 'NONE', #7006, .T. ) ;
#8136=DIRECTION ( 'NONE',  ( 1.000000000000000000, 0.000000000000000000, 0.000000000000000000 ) ) ;
#8138=VECTOR ( 'NONE', #7013, 1000.000000000000000 ) ;
#8139=DIRECTION ( 'NONE',  ( 0.000000000000000000, 0.000000000000000000, 1.000000000000000000 ) ) ;
#8140=AXIS2_PLACEMENT_3D ( 'NONE', #5466, #7952, #7804 ) ;
#8141=ORIENTED_EDGE ( 'NONE', *, *, #12138, .T. ) ;
#8142=EDGE_CURVE ( 'NONE', #3633, #14620, #2902, .T. ) ;
#8144=LINE ( 'NONE', #2369, #3963 ) ;
#8145=EDGE_CURVE ( 'NONE', #12042, #9441, #3192, .T. ) ;
#8146=CARTESIAN_POINT ( 'NONE',  ( 89.61631465359491244, 37.12029293941346708, -10.50000000000000000 ) ) ;
#8147=PLANE ( 'NONE',  #6399 ) ;
#8149=AXIS2_PLACEMENT_3D ( 'NONE', #11595, #6860, #3236 ) ;
#8150=EDGE_CURVE ( 'NONE', #5144, #14931, #9919, .T. ) ;
#8151=DIRECTION ( 'NONE',  ( 1.000000000000000000, 0.000000000000000000, 0.000000000000000000 ) ) ;
#8152=VERTEX_POINT ( 'NONE', #9937 ) ;
#8153=CARTESIAN_POINT ( 'NONE',  ( -52.54657765281192638, 6.917888187662934563, -13.00000000000000178 ) ) ;
#8154=DIRECTION ( 'NONE',  ( 0.000000000000000000, 0.000000000000000000, 1.000000000000000000 ) ) ;
#8155=DIRECTION ( 'NONE',  ( 1.000000000000000000, 0.000000000000000000, 0.000000000000000000 ) ) ;
#8156=CARTESIAN_POINT ( 'NONE',  ( -9.706953719245875689, -57.06275842387046993, -8.000000000000000000 ) ) ;
#8157=EDGE_CURVE ( 'NONE', #1607, #900, #11877, .T. ) ;
#8159=EDGE_CURVE ( 'NONE', #11131, #7351, #3635, .T. ) ;
#8160=AXIS2_PLACEMENT_3D ( 'NONE', #14837, #9637, #9569 ) ;
#8161=CARTESIAN_POINT ( 'NONE',  ( 46.24878538001313188, -27.00670028307179749, -10.50000000000000000 ) ) ;
#8162=CARTESIAN_POINT ( 'NONE',  ( 0.000000000000000000, 0.000000000000000000, -28.00000000000000000 ) ) ;
#8163=DIRECTION ( 'NONE',  ( 0.000000000000000000, 0.000000000000000000, 1.000000000000000000 ) ) ;
#8164=VERTEX_POINT ( 'NONE', #1213 ) ;
#8165=ORIENTED_EDGE ( 'NONE', *, *, #4343, .F. ) ;
#8166=EDGE_CURVE ( 'NONE', #9519, #11532, #9178, .T. ) ;
#8167=ORIENTED_EDGE ( 'NONE', *, *, #2260, .T. ) ;
#8168=DIRECTION ( 'NONE',  ( 1.000000000000000000, 0.000000000000000000, 0.000000000000000000 ) ) ;
#8169=LINE ( 'NONE', #11604, #1729 ) ;
#8170=CARTESIAN_POINT ( 'NONE',  ( 69.20695371924547601, 57.06275842387054098, -10.50000000000000000 ) ) ;
#8171=DIRECTION ( 'NONE',  ( 1.000000000000000000, 0.000000000000000000, 0.000000000000000000 ) ) ;
#8173=CARTESIAN_POINT ( 'NONE',  ( 39.30189486418243661, 33.47282819776626894, 8.000000000000000000 ) ) ;
#8177=FACE_OUTER_BOUND ( 'NONE', #10535, .T. ) ;
#8178=FACE_OUTER_BOUND ( 'NONE', #3791, .T. ) ;
#8179=EDGE_LOOP ( 'NONE', ( #14529, #13325, #11155, #2718, #5463 ) ) ;
#8180=VERTEX_POINT ( 'NONE', #5833 ) ;
#8181=DIRECTION ( 'NONE',  ( 0.000000000000000000, 0.000000000000000000, 1.000000000000000000 ) ) ;
#8183=ORIENTED_EDGE ( 'NONE', *, *, #9893, .F. ) ;
#8184=DIRECTION ( 'NONE',  ( 1.000000000000000000, 0.000000000000000000, 0.000000000000000000 ) ) ;
#8185=CARTESIAN_POINT ( 'NONE',  ( 0.000000000000000000, 0.000000000000000000, 8.000000000000000000 ) ) ;
#8186=DIRECTION ( 'NONE',  ( 1.000000000000000000, 0.000000000000000000, 0.000000000000000000 ) ) ;
#8187=CARTESIAN_POINT ( 'NONE',  ( -52.04657765281192638, 6.917888187662934563, 10.49999999999999822 ) ) ;
#8190=LINE ( 'NONE', #68, #719 ) ;
#8191=ORIENTED_EDGE ( 'NONE', *, *, #6799, .T. ) ;
#8192=DIRECTION ( 'NONE',  ( -0.000000000000000000, -0.000000000000000000, -1.000000000000000000 ) ) ;
#8193=ADVANCED_FACE ( 'NONE', ( #11393 ), #12683, .T. ) ;
#8194=FACE_OUTER_BOUND ( 'NONE', #14280, .T. ) ;
#8195=EDGE_CURVE ( 'NONE', #3842, #8710, #8190, .T. ) ;
#8196=VERTEX_POINT ( 'NONE', #5906 ) ;
#8199=EDGE_LOOP ( 'NONE', ( #1028, #10584, #8720, #8578 ) ) ;
#8201=CARTESIAN_POINT ( 'NONE',  ( -42.04772703543551415, -32.26435573746212526, -10.50000000000000000 ) ) ;
#8203=CARTESIAN_POINT ( 'NONE',  ( 0.000000000000000000, 0.000000000000000000, -8.000000000000000000 ) ) ;
#8205=AXIS2_PLACEMENT_3D ( 'NONE', #4499, #5839, #6821 ) ;
#8209=ORIENTED_EDGE ( 'NONE', *, *, #7536, .F. ) ;
#8212=CARTESIAN_POINT ( 'NONE',  ( 0.000000000000000000, 0.000000000000000000, -10.50000000000000000 ) ) ;
#8213=DIRECTION ( 'NONE',  ( 0.000000000000000000, 0.000000000000000000, -1.000000000000000000 ) ) ;
#8214=VERTEX_POINT ( 'NONE', #14888 ) ;
#8215=DIRECTION ( 'NONE',  ( -0.000000000000000000, -0.000000000000000000, 1.000000000000000000 ) ) ;
#8216=ORIENTED_EDGE ( 'NONE', *, *, #10102, .T. ) ;
#8218=DIRECTION ( 'NONE',  ( 0.000000000000000000, 0.000000000000000000, 1.000000000000000000 ) ) ;
#8219=FACE_OUTER_BOUND ( 'NONE', #6621, .T. ) ;
#8221=DIRECTION ( 'NONE',  ( 0.000000000000000000, 0.000000000000000000, 1.000000000000000000 ) ) ;
#8222=FACE_OUTER_BOUND ( 'NONE', #3674, .T. ) ;
#8225=ORIENTED_EDGE ( 'NONE', *, *, #5748, .F. ) ;
#8226=DIRECTION ( 'NONE',  ( 0.000000000000000000, 0.000000000000000000, 1.000000000000000000 ) ) ;
#8228=DIRECTION ( 'NONE',  ( 0.000000000000000000, 0.000000000000000000, -1.000000000000000000 ) ) ;
#8229=ORIENTED_EDGE ( 'NONE', *, *, #5827, .F. ) ;
#8230=CIRCLE ( 'NONE', #10168, 3.000000000000002665 ) ;
#8231=ORIENTED_EDGE ( 'NONE', *, *, #12994, .T. ) ;
#8235=DIRECTION ( 'NONE',  ( 1.000000000000000000, 0.000000000000000000, 0.000000000000000000 ) ) ;
#8236=CARTESIAN_POINT ( 'NONE',  ( -68.58935777509570642, -68.58935777509452691, 8.000000000000000000 ) ) ;
#8237=DIRECTION ( 'NONE',  ( 0.000000000000000000, 0.000000000000000000, -1.000000000000000000 ) ) ;
#8239=AXIS2_PLACEMENT_3D ( 'NONE', #10582, #10358, #4668 ) ;
#8240=LINE ( 'NONE', #124, #2811 ) ;
#8242=ORIENTED_EDGE ( 'NONE', *, *, #5517, .T. ) ;
#8244=ORIENTED_EDGE ( 'NONE', *, *, #12023, .F. ) ;
#8245=AXIS2_PLACEMENT_3D ( 'NONE', #3882, #2740, #9562 ) ;
#8246=EDGE_CURVE ( 'NONE', #6195, #5327, #14791, .T. ) ;
#8247=CARTESIAN_POINT ( 'NONE',  ( 50.00000000000000000, -6.123233995736766085E-15, -8.000000000000000000 ) ) ;
#8248=CARTESIAN_POINT ( 'NONE',  ( 14.07862063237891981, -50.84834283436993729, -10.50000000000000000 ) ) ;
#8249=CYLINDRICAL_SURFACE ( 'NONE', #3972, 59.50000000000000711 ) ;
#8250=VERTEX_POINT ( 'NONE', #11478 ) ;
#8251=CIRCLE ( 'NONE', #13837, 63.00000000000000000 ) ;
#8252=VERTEX_POINT ( 'NONE', #13982 ) ;
#8253=CARTESIAN_POINT ( 'NONE',  ( -52.54657765281192638, 6.917888187662934563, -10.50000000000000000 ) ) ;
#8254=AXIS2_PLACEMENT_3D ( 'NONE', #1449, #2511, #13223 ) ;
#8255=VERTEX_POINT ( 'NONE', #3573 ) ;
#8256=ADVANCED_FACE ( 'NONE', ( #5688 ), #10325, .F. ) ;
#8257=CIRCLE ( 'NONE', #2683, 52.50000000000000711 ) ;
#8260=CARTESIAN_POINT ( 'NONE',  ( -44.79355920668832880, -31.05588327715819474, 8.000000000000000000 ) ) ;
#8261=PRESENTATION_STYLE_ASSIGNMENT (( #3942 ) ) ;
#8262=VECTOR ( 'NONE', #14970, 1000.000000000000000 ) ;
#8265=VECTOR ( 'NONE', #13899, 1000.000000000000000 ) ;
#8266=DIRECTION ( 'NONE',  ( 1.000000000000000000, 0.000000000000000000, 0.000000000000000000 ) ) ;
#8268=AXIS2_PLACEMENT_3D ( 'NONE', #3247, #906, #1749 ) ;
#8270=VECTOR ( 'NONE', #10915, 1000.000000000000000 ) ;
#8271=ORIENTED_EDGE ( 'NONE', *, *, #11094, .T. ) ;
#8273=AXIS2_PLACEMENT_3D ( 'NONE', #5746, #10228, #2262 ) ;
#8275=ORIENTED_EDGE ( 'NONE', *, *, #4089, .F. ) ;
#8277=AXIS2_PLACEMENT_3D ( 'NONE', #12634, #10050, #5427 ) ;
#8278=DIRECTION ( 'NONE',  ( 1.000000000000000000, 0.000000000000000000, -0.000000000000000000 ) ) ;
#8280=CARTESIAN_POINT ( 'NONE',  ( -33.48561063518626923, 47.21331623427104063, -10.50000000000000000 ) ) ;
#8283=ORIENTED_EDGE ( 'NONE', *, *, #1979, .F. ) ;
#8284=EDGE_CURVE ( 'NONE', #14147, #571, #1454, .T. ) ;
#8285=DIRECTION ( 'NONE',  ( 1.000000000000000000, 0.000000000000000000, 0.000000000000000000 ) ) ;
#8286=EDGE_CURVE ( 'NONE', #8164, #11873, #4636, .T. ) ;
#8287=AXIS2_PLACEMENT_3D ( 'NONE', #2143, #3214, #794 ) ;
#8288=ORIENTED_EDGE ( 'NONE', *, *, #9078, .F. ) ;
#8289=PLANE ( 'NONE',  #5731 ) ;
#8291=CIRCLE ( 'NONE', #12180, 3.000000000000002665 ) ;
#8292=DIRECTION ( 'NONE',  ( 1.000000000000000000, 0.000000000000000000, 0.000000000000000000 ) ) ;
#8297=AXIS2_PLACEMENT_3D ( 'NONE', #1802, #13555, #3166 ) ;
#8299=EDGE_CURVE ( 'NONE', #11315, #5870, #8230, .T. ) ;
#8300=DIRECTION ( 'NONE',  ( 0.000000000000000000, 0.000000000000000000, 1.000000000000000000 ) ) ;
#8301=CARTESIAN_POINT ( 'NONE',  ( -68.58935777509570642, -68.58935777509452691, -13.00000000000000178 ) ) ;
#8302=CYLINDRICAL_SURFACE ( 'NONE', #9679, 0.5000000000000043299 ) ;
#8303=CIRCLE ( 'NONE', #54, 63.00000000000000000 ) ;
#8304=DIRECTION ( 'NONE',  ( 0.000000000000000000, 0.000000000000000000, 1.000000000000000000 ) ) ;
#8305=EDGE_CURVE ( 'NONE', #8402, #1144, #14043, .T. ) ;
#8306=ORIENTED_EDGE ( 'NONE', *, *, #14856, .F. ) ;
#8307=FACE_OUTER_BOUND ( 'NONE', #10477, .T. ) ;
#8309=AXIS2_PLACEMENT_3D ( 'NONE', #2304, #11585, #5780 ) ;
#8310=DIRECTION ( 'NONE',  ( -0.000000000000000000, -0.000000000000000000, 1.000000000000000000 ) ) ;
#8311=EDGE_LOOP ( 'NONE', ( #12766, #4529, #10960, #740 ) ) ;
#8314=ORIENTED_EDGE ( 'NONE', *, *, #1390, .F. ) ;
#8317=CARTESIAN_POINT ( 'NONE',  ( 37.12029293941379393, 89.61631465359479876, -8.000000000000000000 ) ) ;
#8320=ORIENTED_EDGE ( 'NONE', *, *, #14291, .F. ) ;
#8321=EDGE_LOOP ( 'NONE', ( #4623, #1062, #8050, #6413, #13188, #3601 ) ) ;
#8323=CARTESIAN_POINT ( 'NONE',  ( 3.000000000000004885, -97.00000000000000000, -8.000000000000000000 ) ) ;
#8325=EDGE_CURVE ( 'NONE', #11061, #8180, #5613, .T. ) ;
#8326=CIRCLE ( 'NONE', #12215, 3.000000000000002665 ) ;
#8327=EDGE_CURVE ( 'NONE', #1613, #12145, #14551, .T. ) ;
#8328=DIRECTION ( 'NONE',  ( 0.000000000000000000, 0.000000000000000000, 1.000000000000000000 ) ) ;
#8329=ORIENTED_EDGE ( 'NONE', *, *, #7554, .F. ) ;
#8331=LINE ( 'NONE', #7183, #11795 ) ;
#8334=VECTOR ( 'NONE', #10480, 1000.000000000000000 ) ;
#8335=CARTESIAN_POINT ( 'NONE',  ( 37.53686968382241673, 89.89283556784525331, -10.50000000000000000 ) ) ;
#8337=DIRECTION ( 'NONE',  ( -0.000000000000000000, -0.000000000000000000, 1.000000000000000000 ) ) ;
#8338=CIRCLE ( 'NONE', #11007, 53.55662432702593634 ) ;
#8340=DIRECTION ( 'NONE',  ( 1.000000000000000000, 0.000000000000000000, 0.000000000000000000 ) ) ;
#8341=ORIENTED_EDGE ( 'NONE', *, *, #13933, .T. ) ;
#8342=DIRECTION ( 'NONE',  ( 1.000000000000000000, 0.000000000000000000, 0.000000000000000000 ) ) ;
#8343=CYLINDRICAL_SURFACE ( 'NONE', #8712, 0.5000000000000043299 ) ;
#8345=CARTESIAN_POINT ( 'NONE',  ( 100.0000000000000000, -3.430248998885766286E-13, 8.000000000000000000 ) ) ;
#8346=EDGE_CURVE ( 'NONE', #6889, #2988, #522, .T. ) ;
#8347=ADVANCED_FACE ( 'NONE', ( #3867 ), #4851, .T. ) ;
#8348=VECTOR ( 'NONE', #13191, 1000.000000000000000 ) ;
#8350=AXIS2_PLACEMENT_3D ( 'NONE', #14410, #10686, #2489 ) ;
#8351=ORIENTED_EDGE ( 'NONE', *, *, #1652, .F. ) ;
#8353=CARTESIAN_POINT ( 'NONE',  ( -12.86891638962156215, 56.43380494353993271, 10.49999999999999822 ) ) ;
#8354=ORIENTED_EDGE ( 'NONE', *, *, #5567, .F. ) ;
#8356=AXIS2_PLACEMENT_3D ( 'NONE', #5938, #10352, #2308 ) ;
#8359=CARTESIAN_POINT ( 'NONE',  ( 19.68583958711425552, -30.74264578624780597, -28.00000000000000000 ) ) ;
#8360=AXIS2_PLACEMENT_3D ( 'NONE', #4145, #5571, #11351 ) ;
#8361=AXIS2_PLACEMENT_3D ( 'NONE', #13361, #10930, #12013 ) ;
#8363=ORIENTED_EDGE ( 'NONE', *, *, #7692, .F. ) ;
#8367=CARTESIAN_POINT ( 'NONE',  ( 38.26834323650903968, 92.38795325112864987, -8.000000000000000000 ) ) ;
#8368=AXIS2_PLACEMENT_3D ( 'NONE', #11951, #241, #6156 ) ;
#8369=CARTESIAN_POINT ( 'NONE',  ( 57.06275842387049835, -9.706953719245678514, 8.000000000000000000 ) ) ;
#8370=AXIS2_PLACEMENT_3D ( 'NONE', #12455, #3190, #992 ) ;
#8371=CARTESIAN_POINT ( 'NONE',  ( -42.50536573064432133, -32.06294366074479996, -10.50000000000000000 ) ) ;
#8373=EDGE_CURVE ( 'NONE', #14780, #8393, #2655, .T. ) ;
#8374=CARTESIAN_POINT ( 'NONE',  ( -42.04772703543551415, -32.26435573746212526, 8.000000000000000000 ) ) ;
#8375=ORIENTED_EDGE ( 'NONE', *, *, #5136, .F. ) ;
#8376=ORIENTED_EDGE ( 'NONE', *, *, #2845, .T. ) ;
#8377=CARTESIAN_POINT ( 'NONE',  ( -23.49999999999971223, -45.89934640057541060, 8.000000000000000000 ) ) ;
#8378=CYLINDRICAL_SURFACE ( 'NONE', #7807, 59.50000000000000000 ) ;
#8383=VERTEX_POINT ( 'NONE', #14196 ) ;
#8384=PLANE ( 'NONE',  #895 ) ;
#8385=DIRECTION ( 'NONE',  ( 1.000000000000000000, 0.000000000000000000, 0.000000000000000000 ) ) ;
#8386=CARTESIAN_POINT ( 'NONE',  ( -36.14014761921588104, 11.74264578624790190, -25.50000000000000355 ) ) ;
#8388=EDGE_CURVE ( 'NONE', #2149, #12781, #6765, .T. ) ;
#8391=ADVANCED_FACE ( 'NONE', ( #14415 ), #8343, .F. ) ;
#8393=VERTEX_POINT ( 'NONE', #6205 ) ;
#8394=DIRECTION ( 'NONE',  ( 0.000000000000000000, 0.000000000000000000, 1.000000000000000000 ) ) ;
#8395=FACE_OUTER_BOUND ( 'NONE', #2186, .T. ) ;
#8402=VERTEX_POINT ( 'NONE', #9472 ) ;
#8403=ORIENTED_EDGE ( 'NONE', *, *, #5268, .T. ) ;
#8405=DIRECTION ( 'NONE',  ( 0.000000000000000000, 0.000000000000000000, 1.000000000000000000 ) ) ;
#8406=CARTESIAN_POINT ( 'NONE',  ( -47.21331623427138879, -33.48561063518577896, -13.00000000000000178 ) ) ;
#8407=DIRECTION ( 'NONE',  ( -1.000000000000000000, 0.000000000000000000, 0.000000000000000000 ) ) ;
#8408=ORIENTED_EDGE ( 'NONE', *, *, #4130, .F. ) ;
#8409=EDGE_LOOP ( 'NONE', ( #9819, #258, #6332, #6035 ) ) ;
#8410=DIRECTION ( 'NONE',  ( -1.000000000000000000, 0.000000000000000000, 0.000000000000000000 ) ) ;
#8411=CIRCLE ( 'NONE', #13022, 0.5000000000000004441 ) ;
#8412=VERTEX_POINT ( 'NONE', #214 ) ;
#8413=CARTESIAN_POINT ( 'NONE',  ( -68.58935777509427112, 68.58935777509594800, -8.000000000000000000 ) ) ;
#8414=EDGE_CURVE ( 'NONE', #11296, #5532, #235, .T. ) ;
#8415=DIRECTION ( 'NONE',  ( 1.000000000000000000, 0.000000000000000000, 0.000000000000000000 ) ) ;
#8416=LINE ( 'NONE', #7111, #11904 ) ;
#8417=VERTEX_POINT ( 'NONE', #7192 ) ;
#8419=CARTESIAN_POINT ( 'NONE',  ( 68.58935777509475429, -68.58935777509547904, -10.50000000000000000 ) ) ;
#8421=VERTEX_POINT ( 'NONE', #12905 ) ;
#8423=VERTEX_POINT ( 'NONE', #10618 ) ;
#8428=AXIS2_PLACEMENT_3D ( 'NONE', #5677, #13809, #6362 ) ;
#8429=EDGE_CURVE ( 'NONE', #469, #14514, #2947, .T. ) ;
#8431=CYLINDRICAL_SURFACE ( 'NONE', #8735, 0.5000000000000004441 ) ;
#8432=DIRECTION ( 'NONE',  ( 1.000000000000000000, 0.000000000000000000, 0.000000000000000000 ) ) ;
#8434=ORIENTED_EDGE ( 'NONE', *, *, #14365, .F. ) ;
#8435=CARTESIAN_POINT ( 'NONE',  ( 0.000000000000000000, 0.000000000000000000, 8.000000000000000000 ) ) ;
#8436=ORIENTED_EDGE ( 'NONE', *, *, #14810, .T. ) ;
#8437=EDGE_CURVE ( 'NONE', #7919, #9694, #7540, .T. ) ;
#8438=CARTESIAN_POINT ( 'NONE',  ( -52.54657765281192638, 6.917888187662934563, -8.000000000000000000 ) ) ;
#8440=DIRECTION ( 'NONE',  ( -1.000000000000000000, 0.000000000000000000, 0.000000000000000000 ) ) ;
#8444=DIRECTION ( 'NONE',  ( -1.000000000000000000, 0.000000000000000000, 0.000000000000000000 ) ) ;
#8445=ORIENTED_EDGE ( 'NONE', *, *, #10347, .T. ) ;
#8446=EDGE_CURVE ( 'NONE', #13092, #11131, #11447, .T. ) ;
#8448=CARTESIAN_POINT ( 'NONE',  ( 57.06275842387049835, -9.706953719245678514, -13.00000000000000178 ) ) ;
#8449=DIRECTION ( 'NONE',  ( 1.000000000000000000, -7.105427357601001859E-15, 0.000000000000000000 ) ) ;
#8450=CARTESIAN_POINT ( 'NONE',  ( 27.00670028307162340, 46.24878538001323136, -10.50000000000000000 ) ) ;
#8452=CARTESIAN_POINT ( 'NONE',  ( 6.917888187663118416, 52.54657765281190507, 10.49999999999999822 ) ) ;
#8453=CARTESIAN_POINT ( 'NONE',  ( -51.19406879332065330, -13.71740939043347041, -10.50000000000000000 ) ) ;
#8454=CARTESIAN_POINT ( 'NONE',  ( 49.00442420935993226, -30.80502811811213704, -10.50000000000000000 ) ) ;
#8455=ORIENTED_EDGE ( 'NONE', *, *, #3255, .F. ) ;
#8456=CARTESIAN_POINT ( 'NONE',  ( 47.21331623427115431, 33.48561063518610581, -13.00000000000000178 ) ) ;
#8457=AXIS2_PLACEMENT_3D ( 'NONE', #8966, #13604, #13688 ) ;
#8458=ORIENTED_EDGE ( 'NONE', *, *, #12206, .F. ) ;
#8459=CARTESIAN_POINT ( 'NONE',  ( 36.52608637591580987, -92.55687898036916295, -8.000000000000000000 ) ) ;
#8460=DIRECTION ( 'NONE',  ( 0.000000000000000000, 0.000000000000000000, 1.000000000000000000 ) ) ;
#8463=EDGE_CURVE ( 'NONE', #3549, #7242, #9480, .T. ) ;
#8464=VERTEX_POINT ( 'NONE', #9922 ) ;
#8466=DIRECTION ( 'NONE',  ( 0.000000000000000000, 0.000000000000000000, -1.000000000000000000 ) ) ;
#8468=CARTESIAN_POINT ( 'NONE',  ( -32.26435573746199736, 42.04772703543562073, -8.000000000000000000 ) ) ;
#8469=EDGE_CURVE ( 'NONE', #13798, #5235, #13373, .T. ) ;
#8470=DIRECTION ( 'NONE',  ( 1.000000000000000000, 0.000000000000000000, 0.000000000000000000 ) ) ;
#8471=VERTEX_POINT ( 'NONE', #14572 ) ;
#8472=ORIENTED_EDGE ( 'NONE', *, *, #817, .F. ) ;
#8475=DIRECTION ( 'NONE',  ( -1.000000000000000000, 0.000000000000000000, 0.000000000000000000 ) ) ;
#8476=ORIENTED_EDGE ( 'NONE', *, *, #11876, .F. ) ;
#8477=CIRCLE ( 'NONE', #7985, 56.99999999999999289 ) ;
#8478=DIRECTION ( 'NONE',  ( 0.000000000000000000, 0.000000000000000000, -1.000000000000000000 ) ) ;
#8479=DIRECTION ( 'NONE',  ( 0.000000000000000000, 0.000000000000000000, -1.000000000000000000 ) ) ;
#8480=CYLINDRICAL_SURFACE ( 'NONE', #12381, 59.50000000000000000 ) ;
#8481=ORIENTED_EDGE ( 'NONE', *, *, #6088, .F. ) ;
#8484=ORIENTED_EDGE ( 'NONE', *, *, #8522, .T. ) ;
#8485=EDGE_CURVE ( 'NONE', #9901, #6334, #13131, .T. ) ;
#8486=CARTESIAN_POINT ( 'NONE',  ( 0.000000000000000000, 0.000000000000000000, -10.50000000000000000 ) ) ;
#8487=AXIS2_PLACEMENT_3D ( 'NONE', #11337, #12392, #4281 ) ;
#8488=VERTEX_POINT ( 'NONE', #4176 ) ;
#8489=AXIS2_PLACEMENT_3D ( 'NONE', #13840, #14906, #7053 ) ;
#8490=AXIS2_PLACEMENT_3D ( 'NONE', #9326, #13978, #3571 ) ;
#8492=DIRECTION ( 'NONE',  ( 1.000000000000000000, 0.000000000000000000, 0.000000000000000000 ) ) ;
#8493=CARTESIAN_POINT ( 'NONE',  ( -52.36539807335606156, 6.451868917687758831, -10.50000000000000000 ) ) ;
#8494=DIRECTION ( 'NONE',  ( -1.000000000000000000, 0.000000000000000000, 0.000000000000000000 ) ) ;
#8496=AXIS2_PLACEMENT_3D ( 'NONE', #5306, #7662, #6583 ) ;
#8498=CARTESIAN_POINT ( 'NONE',  ( -31.76435573746199381, 42.04772703543562073, -13.00000000000000178 ) ) ;
#8499=CARTESIAN_POINT ( 'NONE',  ( -37.12029293941250074, 89.61631465359532456, 10.49999999999999822 ) ) ;
#8500=AXIS2_PLACEMENT_3D ( 'NONE', #11979, #13106, #2703 ) ;
#8503=ORIENTED_EDGE ( 'NONE', *, *, #2354, .F. ) ;
#8504=DIRECTION ( 'NONE',  ( -0.000000000000000000, -0.000000000000000000, 1.000000000000000000 ) ) ;
#8505=ORIENTED_EDGE ( 'NONE', *, *, #12371, .F. ) ;
#8508=EDGE_CURVE ( 'NONE', #9888, #5327, #6813, .T. ) ;
#8509=AXIS2_PLACEMENT_3D ( 'NONE', #13347, #11230, #8787 ) ;
#8510=EDGE_CURVE ( 'NONE', #1401, #4053, #10692, .T. ) ;
#8511=CARTESIAN_POINT ( 'NONE',  ( 0.000000000000000000, 0.000000000000000000, -10.50000000000000000 ) ) ;
#8512=CIRCLE ( 'NONE', #5845, 3.000000000000002665 ) ;
#8513=FACE_OUTER_BOUND ( 'NONE', #11215, .T. ) ;
#8517=DIRECTION ( 'NONE',  ( 1.000000000000000000, 0.000000000000000000, 0.000000000000000000 ) ) ;
#8520=FACE_OUTER_BOUND ( 'NONE', #2604, .T. ) ;
#8521=CARTESIAN_POINT ( 'NONE',  ( 56.43380494353997534, 12.86891638962136319, 10.49999999999999822 ) ) ;
#8522=EDGE_CURVE ( 'NONE', #7016, #11742, #4161, .T. ) ;
#8524=DIRECTION ( 'NONE',  ( 0.000000000000000000, 0.000000000000000000, -1.000000000000000000 ) ) ;
#8526=DIRECTION ( 'NONE',  ( 0.000000000000000000, 0.000000000000000000, 1.000000000000000000 ) ) ;
#8528=AXIS2_PLACEMENT_3D ( 'NONE', #7465, #8337, #208 ) ;
#8529=DIRECTION ( 'NONE',  ( 1.000000000000000000, 0.000000000000000000, 0.000000000000000000 ) ) ;
#8530=LINE ( 'NONE', #13173, #9797 ) ;
#8532=CARTESIAN_POINT ( 'NONE',  ( -13.71740939043329277, 51.19406879332069593, -10.50000000000000000 ) ) ;
#8535=ORIENTED_EDGE ( 'NONE', *, *, #6372, .F. ) ;
#8537=VERTEX_POINT ( 'NONE', #6652 ) ;
#8539=CARTESIAN_POINT ( 'NONE',  ( 0.000000000000000000, 0.000000000000000000, -8.000000000000000000 ) ) ;
#8540=CARTESIAN_POINT ( 'NONE',  ( 89.61631465359491244, 37.12029293941346708, -13.00000000000000178 ) ) ;
#8541=ORIENTED_EDGE ( 'NONE', *, *, #7548, .T. ) ;
#8542=VECTOR ( 'NONE', #7390, 1000.000000000000000 ) ;
#8543=LINE ( 'NONE', #4921, #8348 ) ;
#8546=DIRECTION ( 'NONE',  ( 0.000000000000000000, 0.000000000000000000, 1.000000000000000000 ) ) ;
#8547=ORIENTED_EDGE ( 'NONE', *, *, #9029, .T. ) ;
#8548=CIRCLE ( 'NONE', #4945, 53.55662432702593634 ) ;
#8549=ORIENTED_EDGE ( 'NONE', *, *, #13626, .F. ) ;
#8550=DIRECTION ( 'NONE',  ( 0.000000000000000000, 0.000000000000000000, 1.000000000000000000 ) ) ;
#8551=VERTEX_POINT ( 'NONE', #10148 ) ;
#8552=EDGE_CURVE ( 'NONE', #11984, #6973, #4020, .T. ) ;
#8554=DIRECTION ( 'NONE',  ( -1.000000000000000000, 0.000000000000000000, 0.000000000000000000 ) ) ;
#8555=( NAMED_UNIT ( * ) PLANE_ANGLE_UNIT ( ) SI_UNIT ( $, .RADIAN. ) );
#8556=AXIS2_PLACEMENT_3D ( 'NONE', #13166, #1472, #2761 ) ;
#8558=CARTESIAN_POINT ( 'NONE',  ( 2.449293598294700991E-16, -97.00000000000000000, -13.00000000000000178 ) ) ;
#8559=ORIENTED_EDGE ( 'NONE', *, *, #10369, .F. ) ;
#8560=PLANE ( 'NONE',  #4883 ) ;
#8561=CIRCLE ( 'NONE', #7586, 60.50000000000000000 ) ;
#8562=VERTEX_POINT ( 'NONE', #1738 ) ;
#8563=EDGE_LOOP ( 'NONE', ( #12211, #4054 ) ) ;
#8565=CIRCLE ( 'NONE', #1786, 0.5000000000000073275 ) ;
#8566=EDGE_CURVE ( 'NONE', #198, #11105, #5368, .T. ) ;
#8567=EDGE_CURVE ( 'NONE', #13490, #12729, #9966, .T. ) ;
#8568=DIRECTION ( 'NONE',  ( 0.000000000000000000, 0.000000000000000000, -1.000000000000000000 ) ) ;
#8569=DIRECTION ( 'NONE',  ( 1.000000000000000000, 0.000000000000000000, 0.000000000000000000 ) ) ;
#8570=LINE ( 'NONE', #8498, #11900 ) ;
#8572=CARTESIAN_POINT ( 'NONE',  ( -38.79014761921587962, 11.74264578624790190, -28.00000000000000000 ) ) ;
#8573=ORIENTED_EDGE ( 'NONE', *, *, #8195, .F. ) ;
#8575=AXIS2_PLACEMENT_3D ( 'NONE', #596, #8479, #11921 ) ;
#8578=ORIENTED_EDGE ( 'NONE', *, *, #4179, .F. ) ;
#8579=LINE ( 'NONE', #14671, #7678 ) ;
#8580=DIRECTION ( 'NONE',  ( 1.000000000000000000, -1.778456000581264310E-15, 0.000000000000000000 ) ) ;
#8583=ORIENTED_EDGE ( 'NONE', *, *, #817, .T. ) ;
#8586=ORIENTED_EDGE ( 'NONE', *, *, #3367, .T. ) ;
#8587=AXIS2_PLACEMENT_3D ( 'NONE', #9382, #6954, #14030 ) ;
#8588=DIRECTION ( 'NONE',  ( 0.000000000000000000, 0.000000000000000000, 1.000000000000000000 ) ) ;
#8589=VERTEX_POINT ( 'NONE', #9087 ) ;
#8592=DIRECTION ( 'NONE',  ( 0.000000000000000000, 0.000000000000000000, 1.000000000000000000 ) ) ;
#8593=EDGE_CURVE ( 'NONE', #9550, #8921, #286, .T. ) ;
#8595=FACE_OUTER_BOUND ( 'NONE', #11446, .T. ) ;
#8596=AXIS2_PLACEMENT_3D ( 'NONE', #10334, #14974, #4568 ) ;
#8597=EDGE_CURVE ( 'NONE', #14537, #13133, #14336, .T. ) ;
#8600=DIRECTION ( 'NONE',  ( 1.000000000000000000, 0.000000000000000000, -0.000000000000000000 ) ) ;
#8602=CIRCLE ( 'NONE', #5937, 0.5000000000000004441 ) ;
#8603=CARTESIAN_POINT ( 'NONE',  ( 0.000000000000000000, 0.000000000000000000, -10.50000000000000000 ) ) ;
#8605=ORIENTED_EDGE ( 'NONE', *, *, #5903, .F. ) ;
#8607=CIRCLE ( 'NONE', #6666, 0.5000000000000022204 ) ;
#8608=ORIENTED_EDGE ( 'NONE', *, *, #6673, .T. ) ;
#8610=CYLINDRICAL_SURFACE ( 'NONE', #3205, 60.50000000000000000 ) ;
#8611=AXIS2_PLACEMENT_3D ( 'NONE', #7663, #3114, #5308 ) ;
#8612=ADVANCED_FACE ( 'NONE', ( #14950 ), #974, .F. ) ;
#8613=DIRECTION ( 'NONE',  ( -0.000000000000000000, -0.000000000000000000, 1.000000000000000000 ) ) ;
#8614=EDGE_CURVE ( 'NONE', #11081, #6408, #7789, .T. ) ;
#8615=DIRECTION ( 'NONE',  ( -0.000000000000000000, -0.000000000000000000, 1.000000000000000000 ) ) ;
#8618=ORIENTED_EDGE ( 'NONE', *, *, #11746, .T. ) ;
#8620=CIRCLE ( 'NONE', #13734, 0.5000000000000004441 ) ;
#8621=CARTESIAN_POINT ( 'NONE',  ( -26.49999999999971578, -45.89934640057541060, -13.00000000000000178 ) ) ;
#8624=ORIENTED_EDGE ( 'NONE', *, *, #4087, .T. ) ;
#8626=EDGE_LOOP ( 'NONE', ( #9400, #9863, #6580, #11628, #5065 ) ) ;
#8627=CARTESIAN_POINT ( 'NONE',  ( -45.46633369868291652, 26.25000000000019895, -10.50000000000000000 ) ) ;
#8628=VERTEX_POINT ( 'NONE', #7017 ) ;
#8629=VECTOR ( 'NONE', #797, 1000.000000000000000 ) ;
#8633=ORIENTED_EDGE ( 'NONE', *, *, #5049, .T. ) ;
#8635=DIRECTION ( 'NONE',  ( 1.000000000000000000, 0.000000000000000000, 0.000000000000000000 ) ) ;
#8636=ORIENTED_EDGE ( 'NONE', *, *, #3072, .T. ) ;
#8638=CIRCLE ( 'NONE', #7667, 59.50000000000000000 ) ;
#8640=ORIENTED_EDGE ( 'NONE', *, *, #8346, .T. ) ;
#8647=CARTESIAN_POINT ( 'NONE',  ( -89.61631465359441506, 37.12029293941468211, 8.000000000000000000 ) ) ;
#8649=EDGE_CURVE ( 'NONE', #1696, #9753, #3189, .T. ) ;
#8650=LINE ( 'NONE', #14507, #9227 ) ;
#8651=LINE ( 'NONE', #2886, #5290 ) ;
#8653=ADVANCED_FACE ( 'NONE', ( #6796 ), #6722, .T. ) ;
#8654=ADVANCED_FACE ( 'NONE', ( #13886 ), #8098, .T. ) ;
#8655=DIRECTION ( 'NONE',  ( 0.000000000000000000, 0.000000000000000000, 1.000000000000000000 ) ) ;
#8656=FACE_OUTER_BOUND ( 'NONE', #982, .T. ) ;
#8659=ORIENTED_EDGE ( 'NONE', *, *, #8927, .T. ) ;
#8661=ORIENTED_EDGE ( 'NONE', *, *, #12606, .F. ) ;
#8664=VERTEX_POINT ( 'NONE', #12585 ) ;
#8666=CARTESIAN_POINT ( 'NONE',  ( -42.89934640057513349, 26.50000000000019540, -8.000000000000000000 ) ) ;
#8668=CARTESIAN_POINT ( 'NONE',  ( -52.50000000000000711, 0.000000000000000000, -10.50000000000000000 ) ) ;
#8669=LINE ( 'NONE', #558, #1801 ) ;
#8670=CARTESIAN_POINT ( 'NONE',  ( -45.89934640057513349, 26.50000000000019540, -10.50000000000000000 ) ) ;
#8671=CIRCLE ( 'NONE', #9396, 0.5000000000000004441 ) ;
#8672=ORIENTED_EDGE ( 'NONE', *, *, #7474, .T. ) ;
#8674=CARTESIAN_POINT ( 'NONE',  ( 9.917888187663120192, 52.54657765281190507, -8.000000000000000000 ) ) ;
#8675=CARTESIAN_POINT ( 'NONE',  ( 96.58511096861892042, 0.2790467552928839190, -13.00000000000000178 ) ) ;
#8677=CARTESIAN_POINT ( 'NONE',  ( -57.06275842387042729, 9.706953719246069312, 8.000000000000000000 ) ) ;
#8678=EDGE_LOOP ( 'NONE', ( #1655, #6953, #7696, #14175 ) ) ;
#8680=VERTEX_POINT ( 'NONE', #8173 ) ;
#8681=DIRECTION ( 'NONE',  ( 1.000000000000000000, 0.000000000000000000, 0.000000000000000000 ) ) ;
#8682=CARTESIAN_POINT ( 'NONE',  ( -52.04657765281192638, 6.917888187662934563, -13.00000000000000178 ) ) ;
#8684=CARTESIAN_POINT ( 'NONE',  ( 47.21331623427115431, 33.48561063518610581, 8.000000000000000000 ) ) ;
#8687=VERTEX_POINT ( 'NONE', #1056 ) ;
#8689=DIRECTION ( 'NONE',  ( 0.000000000000000000, 0.000000000000000000, -1.000000000000000000 ) ) ;
#8690=CARTESIAN_POINT ( 'NONE',  ( -12.86891638962156215, 56.43380494353993271, -8.000000000000000000 ) ) ;
#8691=ORIENTED_EDGE ( 'NONE', *, *, #6748, .F. ) ;
#8692=EDGE_CURVE ( 'NONE', #2935, #14, #521, .T. ) ;
#8693=ADVANCED_FACE ( 'NONE', ( #5674 ), #9160, .F. ) ;
#8694=ORIENTED_EDGE ( 'NONE', *, *, #3523, .T. ) ;
#8695=ORIENTED_EDGE ( 'NONE', *, *, #2351, .F. ) ;
#8696=EDGE_CURVE ( 'NONE', #3819, #3199, #12639, .T. ) ;
#8701=ORIENTED_EDGE ( 'NONE', *, *, #11727, .T. ) ;
#8702=DIRECTION ( 'NONE',  ( 0.000000000000000000, 0.000000000000000000, 1.000000000000000000 ) ) ;
#8703=DIRECTION ( 'NONE',  ( 0.000000000000000000, 0.000000000000000000, -1.000000000000000000 ) ) ;
#8704=VERTEX_POINT ( 'NONE', #11681 ) ;
#8706=ORIENTED_EDGE ( 'NONE', *, *, #12561, .T. ) ;
#8708=AXIS2_PLACEMENT_3D ( 'NONE', #13378, #2066, #10176 ) ;
#8709=EDGE_CURVE ( 'NONE', #5953, #11449, #2454, .T. ) ;
#8710=VERTEX_POINT ( 'NONE', #4060 ) ;
#8711=DIRECTION ( 'NONE',  ( -1.000000000000000000, 0.000000000000000000, 0.000000000000000000 ) ) ;
#8712=AXIS2_PLACEMENT_3D ( 'NONE', #8558, #10771, #13055 ) ;
#8714=CYLINDRICAL_SURFACE ( 'NONE', #270, 3.000000000000002665 ) ;
#8716=FACE_OUTER_BOUND ( 'NONE', #14368, .T. ) ;
#8717=CARTESIAN_POINT ( 'NONE',  ( 29.51438936481373077, 47.21331623427104063, 8.000000000000000000 ) ) ;
#8718=AXIS2_PLACEMENT_3D ( 'NONE', #9628, #11854, #10852 ) ;
#8720=ORIENTED_EDGE ( 'NONE', *, *, #5240, .T. ) ;
#8721=AXIS2_PLACEMENT_3D ( 'NONE', #4122, #11186, #12173 ) ;
#8722=CARTESIAN_POINT ( 'NONE',  ( -68.58935777509570642, -68.58935777509452691, -13.00000000000000178 ) ) ;
#8723=CYLINDRICAL_SURFACE ( 'NONE', #13045, 56.99999999999999289 ) ;
#8724=CIRCLE ( 'NONE', #8490, 50.00000000000000000 ) ;
#8725=DIRECTION ( 'NONE',  ( 1.000000000000000000, 0.000000000000000000, 0.000000000000000000 ) ) ;
#8727=ORIENTED_EDGE ( 'NONE', *, *, #14004, .F. ) ;
#8730=ORIENTED_EDGE ( 'NONE', *, *, #12705, .T. ) ;
#8732=PLANE ( 'NONE',  #6633 ) ;
#8734=CARTESIAN_POINT ( 'NONE',  ( -41.65105036528990468, -31.95997502295777792, -10.50000000000000000 ) ) ;
#8735=AXIS2_PLACEMENT_3D ( 'NONE', #2739, #14057, #11941 ) ;
#8736=ORIENTED_EDGE ( 'NONE', *, *, #9810, .F. ) ;
#8737=CIRCLE ( 'NONE', #14580, 20.00000000000000000 ) ;
#8739=CARTESIAN_POINT ( 'NONE',  ( -89.61631465359441506, 37.12029293941468211, 10.49999999999999822 ) ) ;
#8741=LINE ( 'NONE', #12325, #6343 ) ;
#8742=EDGE_CURVE ( 'NONE', #1839, #14718, #8028, .T. ) ;
#8743=DIRECTION ( 'NONE',  ( 0.000000000000000000, 0.000000000000000000, 1.000000000000000000 ) ) ;
#8747=DIRECTION ( 'NONE',  ( 1.000000000000000000, 0.000000000000000000, 0.000000000000000000 ) ) ;
#8748=AXIS2_PLACEMENT_3D ( 'NONE', #4324, #10083, #3178 ) ;
#8749=ORIENTED_EDGE ( 'NONE', *, *, #1813, .T. ) ;
#8751=CIRCLE ( 'NONE', #5371, 60.50000000000000000 ) ;
#8752=CARTESIAN_POINT ( 'NONE',  ( -37.12029293941250074, 89.61631465359532456, -8.000000000000000000 ) ) ;
#8753=AXIS2_PLACEMENT_3D ( 'NONE', #8374, #6990, #14005 ) ;
#8755=ORIENTED_EDGE ( 'NONE', *, *, #7534, .T. ) ;
#8756=PRODUCT_DEFINITION_SHAPE ( 'NONE', 'NONE',  #898 ) ;
#8757=ORIENTED_EDGE ( 'NONE', *, *, #8429, .F. ) ;
#8759=ORIENTED_EDGE ( 'NONE', *, *, #2629, .F. ) ;
#8760=AXIS2_PLACEMENT_3D ( 'NONE', #13804, #1272, #1194 ) ;
#8761=DIRECTION ( 'NONE',  ( 1.000000000000000000, 0.000000000000000000, 0.000000000000000000 ) ) ;
#8762=EDGE_CURVE ( 'NONE', #8810, #2149, #1486, .T. ) ;
#8764=EDGE_CURVE ( 'NONE', #406, #3450, #12890, .T. ) ;
#8765=ORIENTED_EDGE ( 'NONE', *, *, #2686, .T. ) ;
#8767=AXIS2_PLACEMENT_3D ( 'NONE', #5506, #955, #2999 ) ;
#8770=ORIENTED_EDGE ( 'NONE', *, *, #7118, .T. ) ;
#8773=DIRECTION ( 'NONE',  ( 0.000000000000000000, 0.000000000000000000, 1.000000000000000000 ) ) ;
#8774=CIRCLE ( 'NONE', #1262, 63.00000000000000000 ) ;
#8775=DIRECTION ( 'NONE',  ( -0.000000000000000000, -0.000000000000000000, 1.000000000000000000 ) ) ;
#8777=CIRCLE ( 'NONE', #12430, 60.50000000000000000 ) ;
#8779=EDGE_LOOP ( 'NONE', ( #11501, #893, #13071, #13632 ) ) ;
#8780=LINE ( 'NONE', #12290, #1807 ) ;
#8782=DIRECTION ( 'NONE',  ( 1.000000000000000000, 0.000000000000000000, 0.000000000000000000 ) ) ;
#8783=DIRECTION ( 'NONE',  ( 0.000000000000000000, 0.000000000000000000, -1.000000000000000000 ) ) ;
#8784=ADVANCED_FACE ( 'NONE', ( #413 ), #1695, .F. ) ;
#8785=ORIENTED_EDGE ( 'NONE', *, *, #4824, .F. ) ;
#8786=FACE_OUTER_BOUND ( 'NONE', #5521, .T. ) ;
#8787=DIRECTION ( 'NONE',  ( 1.000000000000000000, 0.000000000000000000, 0.000000000000000000 ) ) ;
#8788=EDGE_CURVE ( 'NONE', #1485, #8869, #5609, .T. ) ;
#8789=EDGE_LOOP ( 'NONE', ( #13450, #11251, #9742, #4774 ) ) ;
#8790=DIRECTION ( 'NONE',  ( -0.000000000000000000, -0.000000000000000000, 1.000000000000000000 ) ) ;
#8792=CIRCLE ( 'NONE', #72, 60.50000000000000000 ) ;
#8796=CARTESIAN_POINT ( 'NONE',  ( 0.000000000000000000, 0.000000000000000000, -8.000000000000000000 ) ) ;
#8797=AXIS2_PLACEMENT_3D ( 'NONE', #9916, #12292, #8782 ) ;
#8798=PRODUCT_DEFINITION_CONTEXT ( 'detailed design', #5439, 'design' ) ;
#8800=DIRECTION ( 'NONE',  ( 1.000000000000000000, 0.000000000000000000, 0.000000000000000000 ) ) ;
#8802=ADVANCED_FACE ( 'NONE', ( #8595 ), #14375, .F. ) ;
#8803=CARTESIAN_POINT ( 'NONE',  ( -2.449293598294708880E-16, 38.00000000000000000, -28.00000000000000000 ) ) ;
#8804=EDGE_CURVE ( 'NONE', #4396, #6265, #14346, .T. ) ;
#8806=FACE_BOUND ( 'NONE', #3806, .T. ) ;
#8810=VERTEX_POINT ( 'NONE', #12103 ) ;
#8813=CARTESIAN_POINT ( 'NONE',  ( -38.26834323650773229, 92.38795325112918988, 8.000000000000000000 ) ) ;
#8814=ORIENTED_EDGE ( 'NONE', *, *, #9624, .F. ) ;
#8816=CYLINDRICAL_SURFACE ( 'NONE', #7881, 3.000000000000002665 ) ;
#8820=AXIS2_PLACEMENT_3D ( 'NONE', #9430, #7226, #3682 ) ;
#8821=DIRECTION ( 'NONE',  ( 1.000000000000000000, 0.000000000000000000, 0.000000000000000000 ) ) ;
#8822=CARTESIAN_POINT ( 'NONE',  ( 47.21331623427115431, 33.48561063518610581, 8.000000000000000000 ) ) ;
#8824=VERTEX_POINT ( 'NONE', #6385 ) ;
#8826=DIRECTION ( 'NONE',  ( 1.000000000000000000, 0.000000000000000000, 0.000000000000000000 ) ) ;
#8830=ORIENTED_EDGE ( 'NONE', *, *, #12301, .T. ) ;
#8831=ORIENTED_EDGE ( 'NONE', *, *, #2407, .T. ) ;
#8833=ORIENTED_EDGE ( 'NONE', *, *, #5240, .F. ) ;
#8834=FACE_OUTER_BOUND ( 'NONE', #2581, .T. ) ;
#8837=CIRCLE ( 'NONE', #3762, 60.50000000000000000 ) ;
#8838=CARTESIAN_POINT ( 'NONE',  ( -52.50000000000000711, 0.000000000000000000, -13.00000000000000178 ) ) ;
#8841=ORIENTED_EDGE ( 'NONE', *, *, #1657, .T. ) ;
#8842=AXIS2_PLACEMENT_3D ( 'NONE', #11975, #8394, #8681 ) ;
#8843=VECTOR ( 'NONE', #12182, 1000.000000000000000 ) ;
#8844=AXIS2_PLACEMENT_3D ( 'NONE', #6750, #11409, #9119 ) ;
#8845=ORIENTED_EDGE ( 'NONE', *, *, #1979, .T. ) ;
#8848=ADVANCED_FACE ( 'NONE', ( #6235 ), #12178, .F. ) ;
#8849=FACE_OUTER_BOUND ( 'NONE', #5291, .T. ) ;
#8851=EDGE_CURVE ( 'NONE', #5997, #5159, #4903, .T. ) ;
#8853=AXIS2_PLACEMENT_3D ( 'NONE', #10172, #5841, #8954 ) ;
#8854=ORIENTED_EDGE ( 'NONE', *, *, #5225, .T. ) ;
#8855=AXIS2_PLACEMENT_3D ( 'NONE', #7032, #9175, #13902 ) ;
#8856=VERTEX_POINT ( 'NONE', #711 ) ;
#8857=EDGE_CURVE ( 'NONE', #12316, #6659, #10467, .T. ) ;
#8860=LINE ( 'NONE', #825, #1291 ) ;
#8861=DIRECTION ( 'NONE',  ( -1.000000000000000000, 0.000000000000000000, 0.000000000000000000 ) ) ;
#8863=ORIENTED_EDGE ( 'NONE', *, *, #1243, .F. ) ;
#8864=CIRCLE ( 'NONE', #4018, 60.50000000000000000 ) ;
#8865=DIRECTION ( 'NONE',  ( 1.000000000000000000, 0.000000000000000000, 0.000000000000000000 ) ) ;
#8867=ORIENTED_EDGE ( 'NONE', *, *, #602, .T. ) ;
#8868=DIRECTION ( 'NONE',  ( 0.000000000000000000, 0.000000000000000000, 1.000000000000000000 ) ) ;
#8869=VERTEX_POINT ( 'NONE', #3293 ) ;
#8870=ORIENTED_EDGE ( 'NONE', *, *, #9127, .T. ) ;
#8871=CARTESIAN_POINT ( 'NONE',  ( 56.43380494353997534, 12.86891638962136319, -10.50000000000000000 ) ) ;
#8872=CIRCLE ( 'NONE', #11803, 3.000000000000002665 ) ;
#8873=EDGE_CURVE ( 'NONE', #9553, #8704, #3198, .T. ) ;
#8874=CARTESIAN_POINT ( 'NONE',  ( 0.000000000000000000, 0.000000000000000000, -10.50000000000000000 ) ) ;
#8876=CARTESIAN_POINT ( 'NONE',  ( 0.000000000000000000, 0.000000000000000000, -8.000000000000000000 ) ) ;
#8877=DIRECTION ( 'NONE',  ( -0.000000000000000000, -0.000000000000000000, 1.000000000000000000 ) ) ;
#8878=ORIENTED_EDGE ( 'NONE', *, *, #6824, .T. ) ;
#8879=CIRCLE ( 'NONE', #9601, 52.50000000000000711 ) ;
#8880=CARTESIAN_POINT ( 'NONE',  ( 31.95997502295791648, -41.65105036528979099, -10.50000000000000000 ) ) ;
#8881=CYLINDRICAL_SURFACE ( 'NONE', #5974, 3.000000000000002665 ) ;
#8882=DIRECTION ( 'NONE',  ( 1.000000000000000000, 0.000000000000000000, 0.000000000000000000 ) ) ;
#8883=ORIENTED_EDGE ( 'NONE', *, *, #3646, .F. ) ;
#8884=CARTESIAN_POINT ( 'NONE',  ( 100.0000000000000000, -1.224646799147353217E-14, -13.00000000000000178 ) ) ;
#8885=VERTEX_POINT ( 'NONE', #7979 ) ;
#8886=EDGE_CURVE ( 'NONE', #13653, #967, #11697, .T. ) ;
#8889=ORIENTED_EDGE ( 'NONE', *, *, #2435, .F. ) ;
#8890=CARTESIAN_POINT ( 'NONE',  ( 0.000000000000000000, 0.000000000000000000, 8.000000000000000000 ) ) ;
#8892=ORIENTED_EDGE ( 'NONE', *, *, #13575, .F. ) ;
#8896=DIRECTION ( 'NONE',  ( 1.000000000000000000, 0.000000000000000000, 0.000000000000000000 ) ) ;
#8897=DIRECTION ( 'NONE',  ( -1.000000000000000000, 0.000000000000000000, 0.000000000000000000 ) ) ;
#8899=DIRECTION ( 'NONE',  ( 0.000000000000000000, 0.000000000000000000, 1.000000000000000000 ) ) ;
#8900=ORIENTED_EDGE ( 'NONE', *, *, #1067, .T. ) ;
#8903=DIRECTION ( 'NONE',  ( -1.000000000000000000, 0.000000000000000000, 0.000000000000000000 ) ) ;
#8904=DIRECTION ( 'NONE',  ( -0.000000000000000000, -0.000000000000000000, 1.000000000000000000 ) ) ;
#8905=EDGE_CURVE ( 'NONE', #7460, #7720, #4175, .T. ) ;
#8906=VERTEX_POINT ( 'NONE', #13607 ) ;
#8909=CARTESIAN_POINT ( 'NONE',  ( -51.53979475227126983, -13.35619814848815601, -13.00000000000000178 ) ) ;
#8910=DIRECTION ( 'NONE',  ( -0.000000000000000000, -0.000000000000000000, -1.000000000000000000 ) ) ;
#8911=CLOSED_SHELL ( 'NONE', ( #8784, #6331, #11842, #1417, #7685, #644, #3141, #14766, #9532, #976, #14562, #6153, #7304, #5467, #13502, #6731, #8391, #7673, #5431, #13335, #14924, #3940, #3775, #10387, #7788, #9309, #11110, #6429, #6439, #5774, #14928, #13483, #1339, #14750, #4637, #7691, #14020, #6351, #14473, #6238, #9445, #5755, #13079, #598, #7482, #5241, #9891, #13605, #10880, #7655, #9169, #6909, #4782, #3337, #14426, #4310, #5456, #4721, #9831, #3435, #4974, #10288, #12791, #14067, #11824, #10241, #410, #10303, #5655, #12204, #14176, #2213, #14941, #11788, #8029, #14981, #3855, #6002, #4683, #789, #4633, #13979, #9903, #4536, #14372, #4071, #11497, #3642, #4371, #1050, #3898, #2317, #6468, #10911, #11936, #11000, #8654, #4954, #11405, #3059, #9580, #11590, #2069, #10853, #4907, #9168, #4905, #7725, #12939, #1889, #1998, #13002, #3148, #7676, #13218, #10295, #4283, #3860, #3664, #1359, #6733, #12688, #7906, #13072, #9308, #2638, #11137, #4313, #791, #5606, #365, #1769, #6557, #5921, #3116, #11086, #8612, #9225, #12329, #7288, #1708, #6829, #6194, #10882, #724, #2735, #7094, #10170, #129, #2355, #3809, #2525, #13522, #9576, #4273, #8009, #11610, #718, #14897, #5294, #12425, #9250, #209, #8653, #6518, #8193, #13783, #1457, #3144, #14327, #11797, #2280, #8347, #2719, #8693, #2388, #6246, #1561, #4930, #4861, #11642, #1337, #10175, #14110, #7944, #9492, #11403, #11114, #7219, #14463, #741, #10888, #4859, #9267, #5048, #4591, #9940, #11570, #3876, #10939, #3802, #4238, #2299, #14658, #10744, #13844, #9671, #7831, #2218, #9494, #7496, #6000, #4220, #13503, #14047, #11499, #4816, #10984, #13810, #6435, #6061, #9913, #4195, #447, #2310, #6969, #1484, #1193, #2944, #2087, #8848, #1853, #10557, #5551, #834, #9369, #14179, #10634, #322, #3607, #4409, #11833, #7776, #12751, #3566, #13436, #6152, #13888, #1540, #1648, #12387, #10513, #12578, #2477, #10532, #920, #3424, #6749, #10650, #5919, #14996, #1254, #186, #12598, #10097, #14100, #10470, #8256, #14381, #5515, #13529, #2164, #7314, #548, #13881, #13171, #14983, #11084, #1152, #9319, #9075, #8802, #6330 ) ) ;
#8913=LINE ( 'NONE', #12195, #66 ) ;
#8914=ORIENTED_EDGE ( 'NONE', *, *, #1431, .F. ) ;
#8916=ORIENTED_EDGE ( 'NONE', *, *, #13694, .F. ) ;
#8917=CARTESIAN_POINT ( 'NONE',  ( -36.70371619500578220, -89.33979373934407420, -10.50000000000000000 ) ) ;
#8918=CARTESIAN_POINT ( 'NONE',  ( 72.70695371924547601, 57.06275842387054098, 8.000000000000000000 ) ) ;
#8919=DIRECTION ( 'NONE',  ( 1.000000000000000000, 0.000000000000000000, 0.000000000000000000 ) ) ;
#8920=EDGE_LOOP ( 'NONE', ( #8034, #7594, #6727, #9967, #3418, #10592 ) ) ;
#8921=VERTEX_POINT ( 'NONE', #9044 ) ;
#8922=VERTEX_POINT ( 'NONE', #13465 ) ;
#8924=FACE_OUTER_BOUND ( 'NONE', #4788, .T. ) ;
#8925=EDGE_CURVE ( 'NONE', #2119, #6659, #8970, .T. ) ;
#8926=DIRECTION ( 'NONE',  ( 0.000000000000000000, 0.000000000000000000, 1.000000000000000000 ) ) ;
#8927=EDGE_CURVE ( 'NONE', #6973, #2752, #3442, .T. ) ;
#8928=ORIENTED_EDGE ( 'NONE', *, *, #10192, .T. ) ;
#8929=DIRECTION ( 'NONE',  ( -0.000000000000000000, -0.000000000000000000, 1.000000000000000000 ) ) ;
#8931=ORIENTED_EDGE ( 'NONE', *, *, #8485, .T. ) ;
#8933=ORIENTED_EDGE ( 'NONE', *, *, #4269, .T. ) ;
#8935=ORIENTED_EDGE ( 'NONE', *, *, #12727, .T. ) ;
#8939=CARTESIAN_POINT ( 'NONE',  ( 53.63365512954693770, -9.714003807513686084, -13.00000000000000178 ) ) ;
#8940=CIRCLE ( 'NONE', #2167, 3.000000000000002665 ) ;
#8942=DIRECTION ( 'NONE',  ( 1.000000000000000000, 0.000000000000000000, 0.000000000000000000 ) ) ;
#8943=DIRECTION ( 'NONE',  ( -1.000000000000000000, 0.000000000000000000, 0.000000000000000000 ) ) ;
#8944=EDGE_CURVE ( 'NONE', #11984, #12052, #5619, .T. ) ;
#8947=VERTEX_POINT ( 'NONE', #10116 ) ;
#8949=FACE_OUTER_BOUND ( 'NONE', #1907, .T. ) ;
#8951=AXIS2_PLACEMENT_3D ( 'NONE', #7810, #5247, #14664 ) ;
#8954=DIRECTION ( 'NONE',  ( 1.000000000000000000, 0.000000000000000000, 0.000000000000000000 ) ) ;
#8956=CARTESIAN_POINT ( 'NONE',  ( 0.000000000000000000, 0.000000000000000000, -13.00000000000000178 ) ) ;
#8957=ORIENTED_EDGE ( 'NONE', *, *, #7554, .T. ) ;
#8961=AXIS2_PLACEMENT_3D ( 'NONE', #3979, #7225, #9725 ) ;
#8963=DIRECTION ( 'NONE',  ( 0.000000000000000000, 0.000000000000000000, 1.000000000000000000 ) ) ;
#8965=AXIS2_PLACEMENT_3D ( 'NONE', #5109, #9722, #13162 ) ;
#8966=CARTESIAN_POINT ( 'NONE',  ( 13.71740939043365337, -51.19406879332061067, 10.49999999999999822 ) ) ;
#8967=VECTOR ( 'NONE', #5395, 1000.000000000000000 ) ;
#8969=EDGE_CURVE ( 'NONE', #8073, #5446, #9724, .T. ) ;
#8970=LINE ( 'NONE', #4291, #13140 ) ;
#8973=EDGE_CURVE ( 'NONE', #14518, #7413, #8774, .T. ) ;
#8974=DIRECTION ( 'NONE',  ( 0.000000000000000000, 0.000000000000000000, 1.000000000000000000 ) ) ;
#8975=CARTESIAN_POINT ( 'NONE',  ( 52.54657765281197612, -6.917888187662545540, 8.000000000000000000 ) ) ;
#8976=EDGE_CURVE ( 'NONE', #7044, #12589, #9008, .T. ) ;
#8977=DIRECTION ( 'NONE',  ( 1.000000000000000000, 0.000000000000000000, 0.000000000000000000 ) ) ;
#8978=CIRCLE ( 'NONE', #2431, 53.55662432702593634 ) ;
#8979=DIRECTION ( 'NONE',  ( 0.000000000000000000, 0.000000000000000000, -1.000000000000000000 ) ) ;
#8980=EDGE_LOOP ( 'NONE', ( #9751, #6624, #2423, #11664 ) ) ;
#8982=DIRECTION ( 'NONE',  ( 0.000000000000000000, 0.000000000000000000, -1.000000000000000000 ) ) ;
#8984=DIRECTION ( 'NONE',  ( 1.000000000000000000, 0.000000000000000000, 0.000000000000000000 ) ) ;
#8985=FACE_OUTER_BOUND ( 'NONE', #41, .T. ) ;
#8986=AXIS2_PLACEMENT_3D ( 'NONE', #3716, #10608, #4015 ) ;
#8988=DIRECTION ( 'NONE',  ( 0.000000000000000000, 0.000000000000000000, 1.000000000000000000 ) ) ;
#8991=CIRCLE ( 'NONE', #10933, 3.000000000000002665 ) ;
#8993=VERTEX_POINT ( 'NONE', #1097 ) ;
#8996=DIRECTION ( 'NONE',  ( -1.000000000000000000, 0.000000000000000000, 0.000000000000000000 ) ) ;
#9000=AXIS2_PLACEMENT_3D ( 'NONE', #4547, #9306, #6952 ) ;
#9002=ORIENTED_EDGE ( 'NONE', *, *, #10427, .F. ) ;
#9004=DIRECTION ( 'NONE',  ( 0.000000000000000000, 0.000000000000000000, 1.000000000000000000 ) ) ;
#9005=FACE_OUTER_BOUND ( 'NONE', #12210, .T. ) ;
#9006=CARTESIAN_POINT ( 'NONE',  ( 0.000000000000000000, 0.000000000000000000, -13.00000000000000178 ) ) ;
#9008=CIRCLE ( 'NONE', #40, 0.5000000000000038858 ) ;
#9009=DIRECTION ( 'NONE',  ( 0.000000000000000000, 0.000000000000000000, -1.000000000000000000 ) ) ;
#9010=ORIENTED_EDGE ( 'NONE', *, *, #12875, .F. ) ;
#9012=CIRCLE ( 'NONE', #8528, 60.49999999999999289 ) ;
#9013=ORIENTED_EDGE ( 'NONE', *, *, #5082, .F. ) ;
#9014=EDGE_LOOP ( 'NONE', ( #9649, #1261, #5311, #9996, #3169 ) ) ;
#9015=DIRECTION ( 'NONE',  ( 1.000000000000000000, 0.000000000000000000, 0.000000000000000000 ) ) ;
#9017=VECTOR ( 'NONE', #38, 1000.000000000000000 ) ;
#9018=CARTESIAN_POINT ( 'NONE',  ( 32.26435573746228158, -42.04772703543541468, -13.00000000000000178 ) ) ;
#9019=CARTESIAN_POINT ( 'NONE',  ( 26.99988008862626643, 45.88839665196127271, 10.49999999999999822 ) ) ;
#9021=LINE ( 'NONE', #11161, #4989 ) ;
#9023=DIRECTION ( 'NONE',  ( -0.000000000000000000, -0.000000000000000000, 1.000000000000000000 ) ) ;
#9024=VERTEX_POINT ( 'NONE', #7057 ) ;
#9025=DIRECTION ( 'NONE',  ( 1.000000000000000000, 0.000000000000000000, 0.000000000000000000 ) ) ;
#9029=EDGE_CURVE ( 'NONE', #11449, #10669, #3690, .T. ) ;
#9030=ORIENTED_EDGE ( 'NONE', *, *, #507, .F. ) ;
#9032=EDGE_CURVE ( 'NONE', #13122, #7998, #11717, .T. ) ;
#9033=EDGE_CURVE ( 'NONE', #5812, #13295, #2957, .T. ) ;
#9035=FACE_OUTER_BOUND ( 'NONE', #6763, .T. ) ;
#9036=EDGE_CURVE ( 'NONE', #9073, #11672, #1031, .T. ) ;
#9037=DIRECTION ( 'NONE',  ( 0.000000000000000000, 0.000000000000000000, -1.000000000000000000 ) ) ;
#9038=AXIS2_PLACEMENT_3D ( 'NONE', #3346, #7964, #1358 ) ;
#9040=DIRECTION ( 'NONE',  ( -1.000000000000000000, 0.000000000000000000, 0.000000000000000000 ) ) ;
#9041=PLANE ( 'NONE',  #14616 ) ;
#9042=DIRECTION ( 'NONE',  ( 0.000000000000000000, 0.000000000000000000, 1.000000000000000000 ) ) ;
#9044=CARTESIAN_POINT ( 'NONE',  ( -33.49014761921589667, 11.74264578624790190, -28.00000000000000000 ) ) ;
#9046=ORIENTED_EDGE ( 'NONE', *, *, #4079, .T. ) ;
#9049=VECTOR ( 'NONE', #668, 1000.000000000000000 ) ;
#9050=DIRECTION ( 'NONE',  ( 1.000000000000000000, 0.000000000000000000, 0.000000000000000000 ) ) ;
#9051=DIRECTION ( 'NONE',  ( 0.000000000000000000, 0.000000000000000000, 1.000000000000000000 ) ) ;
#9052=VERTEX_POINT ( 'NONE', #2516 ) ;
#9053=CIRCLE ( 'NONE', #11511, 3.000000000000002665 ) ;
#9054=FACE_OUTER_BOUND ( 'NONE', #9077, .T. ) ;
#9056=ORIENTED_EDGE ( 'NONE', *, *, #5096, .F. ) ;
#9057=EDGE_CURVE ( 'NONE', #1886, #7929, #11933, .T. ) ;
#9059=CARTESIAN_POINT ( 'NONE',  ( -13.71740939043329277, 51.19406879332069593, 10.49999999999999822 ) ) ;
#9060=EDGE_CURVE ( 'NONE', #6775, #12166, #8038, .T. ) ;
#9061=DIRECTION ( 'NONE',  ( 1.000000000000000000, 0.000000000000000000, 0.000000000000000000 ) ) ;
#9063=VERTEX_POINT ( 'NONE', #9274 ) ;
#9065=AXIS2_PLACEMENT_3D ( 'NONE', #875, #1020, #1918 ) ;
#9067=VECTOR ( 'NONE', #10625, 1000.000000000000000 ) ;
#9068=DIRECTION ( 'NONE',  ( 1.000000000000000000, 0.000000000000000000, 0.000000000000000000 ) ) ;
#9073=VERTEX_POINT ( 'NONE', #7138 ) ;
#9075=ADVANCED_FACE ( 'NONE', ( #14985 ), #4735, .F. ) ;
#9077=EDGE_LOOP ( 'NONE', ( #10802, #1718, #5042, #3705 ) ) ;
#9078=EDGE_CURVE ( 'NONE', #5604, #1589, #5383, .T. ) ;
#9080=DIRECTION ( 'NONE',  ( 0.000000000000000000, 0.000000000000000000, -1.000000000000000000 ) ) ;
#9081=AXIS2_PLACEMENT_3D ( 'NONE', #13526, #5487, #3130 ) ;
#9083=DIRECTION ( 'NONE',  ( -0.000000000000000000, -0.000000000000000000, -1.000000000000000000 ) ) ;
#9086=ORIENTED_EDGE ( 'NONE', *, *, #2629, .T. ) ;
#9087=CARTESIAN_POINT ( 'NONE',  ( 68.49330278050122445, -68.09867107463004743, 10.49999999999999822 ) ) ;
#9088=EDGE_LOOP ( 'NONE', ( #10837, #10149, #3530, #9707, #7797, #13110, #13641 ) ) ;
#9089=ORIENTED_EDGE ( 'NONE', *, *, #8150, .T. ) ;
#9090=EDGE_CURVE ( 'NONE', #1620, #5654, #4665, .T. ) ;
#9091=DIRECTION ( 'NONE',  ( 0.000000000000000000, 0.000000000000000000, 1.000000000000000000 ) ) ;
#9092=DIRECTION ( 'NONE',  ( 1.000000000000000000, 0.000000000000000000, 0.000000000000000000 ) ) ;
#9093=AXIS2_PLACEMENT_3D ( 'NONE', #9261, #6679, #5766 ) ;
#9094=CIRCLE ( 'NONE', #12986, 3.000000000000002665 ) ;
#9096=AXIS2_PLACEMENT_3D ( 'NONE', #11622, #1211, #12759 ) ;
#9099=ORIENTED_EDGE ( 'NONE', *, *, #2217, .F. ) ;
#9100=ORIENTED_EDGE ( 'NONE', *, *, #6929, .F. ) ;
#9101=CIRCLE ( 'NONE', #7650, 52.50000000000000711 ) ;
#9102=DIRECTION ( 'NONE',  ( 1.000000000000000000, 0.000000000000000000, 0.000000000000000000 ) ) ;
#9103=DIRECTION ( 'NONE',  ( 1.000000000000000000, 0.000000000000000000, 0.000000000000000000 ) ) ;
#9105=DIRECTION ( 'NONE',  ( 0.000000000000000000, 0.000000000000000000, -1.000000000000000000 ) ) ;
#9106=FACE_OUTER_BOUND ( 'NONE', #6228, .T. ) ;
#9108=ORIENTED_EDGE ( 'NONE', *, *, #7325, .T. ) ;
#9109=CARTESIAN_POINT ( 'NONE',  ( 46.63108361037843252, 56.43380494353993271, -13.00000000000000178 ) ) ;
#9110=VERTEX_POINT ( 'NONE', #3742 ) ;
#9111=AXIS2_PLACEMENT_3D ( 'NONE', #12863, #9433, #9511 ) ;
#9113=DIRECTION ( 'NONE',  ( 1.000000000000000000, 0.000000000000000000, 0.000000000000000000 ) ) ;
#9115=LINE ( 'NONE', #3349, #1822 ) ;
#9118=CARTESIAN_POINT ( 'NONE',  ( 0.2790467552932288098, 97.41488903138106537, 10.49999999999999822 ) ) ;
#9119=DIRECTION ( 'NONE',  ( 1.000000000000000000, 0.000000000000000000, 0.000000000000000000 ) ) ;
#9120=DIRECTION ( 'NONE',  ( 0.000000000000000000, 0.000000000000000000, -1.000000000000000000 ) ) ;
#9123=EDGE_CURVE ( 'NONE', #1207, #7348, #14323, .T. ) ;
#9124=CARTESIAN_POINT ( 'NONE',  ( 90.10640870805727332, 37.02125851216391794, -13.00000000000000178 ) ) ;
#9126=EDGE_CURVE ( 'NONE', #1282, #2937, #7772, .T. ) ;
#9127=EDGE_CURVE ( 'NONE', #11326, #212, #2722, .T. ) ;
#9130=CARTESIAN_POINT ( 'NONE',  ( -68.58935777509570642, -68.58935777509452691, -13.00000000000000178 ) ) ;
#9131=DIRECTION ( 'NONE',  ( 0.000000000000000000, 0.000000000000000000, 1.000000000000000000 ) ) ;
#9132=DIRECTION ( 'NONE',  ( 1.000000000000000000, 0.000000000000000000, 0.000000000000000000 ) ) ;
#9134=PLANE ( 'NONE',  #14397 ) ;
#9137=ORIENTED_EDGE ( 'NONE', *, *, #9029, .F. ) ;
#9138=EDGE_CURVE ( 'NONE', #6594, #9373, #1960, .T. ) ;
#9139=CYLINDRICAL_SURFACE ( 'NONE', #1939, 63.00000000000000000 ) ;
#9141=DIRECTION ( 'NONE',  ( -1.000000000000000000, 0.000000000000000000, 0.000000000000000000 ) ) ;
#9144=EDGE_CURVE ( 'NONE', #9553, #2051, #256, .T. ) ;
#9145=EDGE_LOOP ( 'NONE', ( #3029, #12447, #14622, #4252, #9781 ) ) ;
#9146=ORIENTED_EDGE ( 'NONE', *, *, #12247, .T. ) ;
#9147=ORIENTED_EDGE ( 'NONE', *, *, #11364, .F. ) ;
#9150=LINE ( 'NONE', #3544, #9017 ) ;
#9152=VERTEX_POINT ( 'NONE', #2744 ) ;
#9153=ORIENTED_EDGE ( 'NONE', *, *, #2949, .T. ) ;
#9154=CARTESIAN_POINT ( 'NONE',  ( -12.86891638962156215, 56.43380494353993271, -8.000000000000000000 ) ) ;
#9155=CYLINDRICAL_SURFACE ( 'NONE', #14589, 0.5000000000000004441 ) ;
#9156=CARTESIAN_POINT ( 'NONE',  ( -13.71740939043329277, 51.19406879332069593, -10.50000000000000000 ) ) ;
#9158=DIRECTION ( 'NONE',  ( 1.000000000000000000, 0.000000000000000000, 0.000000000000000000 ) ) ;
#9160=PLANE ( 'NONE',  #11923 ) ;
#9161=ORIENTED_EDGE ( 'NONE', *, *, #5815, .F. ) ;
#9162=DIRECTION ( 'NONE',  ( 0.000000000000000000, 0.000000000000000000, 1.000000000000000000 ) ) ;
#9163=ORIENTED_EDGE ( 'NONE', *, *, #11280, .T. ) ;
#9164=EDGE_CURVE ( 'NONE', #10988, #11670, #7438, .T. ) ;
#9167=ORIENTED_EDGE ( 'NONE', *, *, #5724, .F. ) ;
#9168=ADVANCED_FACE ( 'NONE', ( #1455 ), #14354, .T. ) ;
#9169=ADVANCED_FACE ( 'NONE', ( #317 ), #6285, .F. ) ;
#9170=ORIENTED_EDGE ( 'NONE', *, *, #6043, .T. ) ;
#9172=FACE_OUTER_BOUND ( 'NONE', #10700, .T. ) ;
#9174=DIRECTION ( 'NONE',  ( -0.000000000000000000, -0.000000000000000000, -1.000000000000000000 ) ) ;
#9175=DIRECTION ( 'NONE',  ( -0.000000000000000000, -0.000000000000000000, 1.000000000000000000 ) ) ;
#9178=LINE ( 'NONE', #8118, #5318 ) ;
#9182=DIRECTION ( 'NONE',  ( 0.000000000000000000, 0.000000000000000000, 1.000000000000000000 ) ) ;
#9183=ORIENTED_EDGE ( 'NONE', *, *, #13997, .T. ) ;
#9184=FACE_OUTER_BOUND ( 'NONE', #12887, .T. ) ;
#9185=VECTOR ( 'NONE', #10096, 1000.000000000000000 ) ;
#9189=CARTESIAN_POINT ( 'NONE',  ( 42.04772703543530099, 32.26435573746242369, -8.000000000000000000 ) ) ;
#9195=ORIENTED_EDGE ( 'NONE', *, *, #12989, .F. ) ;
#9196=DIRECTION ( 'NONE',  ( -0.000000000000000000, -0.000000000000000000, 1.000000000000000000 ) ) ;
#9197=DIRECTION ( 'NONE',  ( 1.000000000000000000, 0.000000000000000000, 0.000000000000000000 ) ) ;
#9198=CARTESIAN_POINT ( 'NONE',  ( 89.61631465359468507, -37.12029293941410657, -13.00000000000000178 ) ) ;
#9199=ORIENTED_EDGE ( 'NONE', *, *, #8056, .T. ) ;
#9203=CIRCLE ( 'NONE', #11157, 100.0000000000000000 ) ;
#9205=CARTESIAN_POINT ( 'NONE',  ( -1.674280531759324342, -99.48933418828643482, 8.000000000000000000 ) ) ;
#9206=CIRCLE ( 'NONE', #8721, 56.99999999999999289 ) ;
#9207=EDGE_CURVE ( 'NONE', #14795, #10139, #8650, .T. ) ;
#9210=FACE_OUTER_BOUND ( 'NONE', #140, .T. ) ;
#9211=DIRECTION ( 'NONE',  ( 0.000000000000000000, 0.000000000000000000, 1.000000000000000000 ) ) ;
#9212=DIRECTION ( 'NONE',  ( 1.000000000000000000, 0.000000000000000000, 0.000000000000000000 ) ) ;
#9214=ORIENTED_EDGE ( 'NONE', *, *, #14952, .T. ) ;
#9215=ORIENTED_EDGE ( 'NONE', *, *, #595, .F. ) ;
#9218=CIRCLE ( 'NONE', #11167, 3.000000000000002665 ) ;
#9219=CARTESIAN_POINT ( 'NONE',  ( -33.48561063518626923, 47.21331623427104063, -8.000000000000000000 ) ) ;
#9222=DIRECTION ( 'NONE',  ( -1.000000000000000000, 0.000000000000000000, 0.000000000000000000 ) ) ;
#9223=ORIENTED_EDGE ( 'NONE', *, *, #416, .T. ) ;
#9224=EDGE_LOOP ( 'NONE', ( #1653, #6729, #7102, #11182 ) ) ;
#9225=ADVANCED_FACE ( 'NONE', ( #8949 ), #13587, .T. ) ;
#9227=VECTOR ( 'NONE', #997, 1000.000000000000000 ) ;
#9228=ORIENTED_EDGE ( 'NONE', *, *, #1585, .F. ) ;
#9229=AXIS2_PLACEMENT_3D ( 'NONE', #11768, #2801, #9680 ) ;
#9230=DIRECTION ( 'NONE',  ( -1.000000000000000000, 0.000000000000000000, 0.000000000000000000 ) ) ;
#9231=AXIS2_PLACEMENT_3D ( 'NONE', #8236, #6024, #13882 ) ;
#9234=DIRECTION ( 'NONE',  ( 1.000000000000000000, 8.881784197001252323E-16, 0.000000000000000000 ) ) ;
#9235=CYLINDRICAL_SURFACE ( 'NONE', #4029, 3.000000000000002665 ) ;
#9236=CARTESIAN_POINT ( 'NONE',  ( 56.43380494353997534, 12.86891638962136319, -10.50000000000000000 ) ) ;
#9238=ORIENTED_EDGE ( 'NONE', *, *, #11571, .F. ) ;
#9240=DIRECTION ( 'NONE',  ( 0.000000000000000000, 0.000000000000000000, 1.000000000000000000 ) ) ;
#9243=CIRCLE ( 'NONE', #3922, 2.649999999999992806 ) ;
#9244=CIRCLE ( 'NONE', #770, 0.5000000000000038858 ) ;
#9247=ORIENTED_EDGE ( 'NONE', *, *, #172, .T. ) ;
#9248=DIRECTION ( 'NONE',  ( 0.000000000000000000, 0.000000000000000000, 1.000000000000000000 ) ) ;
#9249=DIRECTION ( 'NONE',  ( 0.000000000000000000, 0.000000000000000000, -1.000000000000000000 ) ) ;
#9250=ADVANCED_FACE ( 'NONE', ( #5398, #8806 ), #5616, .T. ) ;
#9251=CARTESIAN_POINT ( 'NONE',  ( 70.71067811865489716, 70.71067811865461294, -8.000000000000000000 ) ) ;
#9252=FACE_OUTER_BOUND ( 'NONE', #449, .T. ) ;
#9253=CARTESIAN_POINT ( 'NONE',  ( 0.5000000000000045519, -97.00000000000000000, -13.00000000000000178 ) ) ;
#9255=ORIENTED_EDGE ( 'NONE', *, *, #9727, .T. ) ;
#9257=EDGE_CURVE ( 'NONE', #12166, #4396, #787, .T. ) ;
#9258=CARTESIAN_POINT ( 'NONE',  ( 69.20695371924547601, 57.06275842387054098, 10.49999999999999822 ) ) ;
#9259=AXIS2_PLACEMENT_3D ( 'NONE', #11247, #1828, #11395 ) ;
#9260=ORIENTED_EDGE ( 'NONE', *, *, #10328, .T. ) ;
#9261=CARTESIAN_POINT ( 'NONE',  ( 89.61631465359491244, 37.12029293941346708, -8.000000000000000000 ) ) ;
#9262=DIRECTION ( 'NONE',  ( -0.000000000000000000, -0.000000000000000000, -1.000000000000000000 ) ) ;
#9264=ORIENTED_EDGE ( 'NONE', *, *, #4734, .T. ) ;
#9267=ADVANCED_FACE ( 'NONE', ( #14742 ), #2967, .T. ) ;
#9273=CIRCLE ( 'NONE', #1519, 0.5000000000000022204 ) ;
#9274=CARTESIAN_POINT ( 'NONE',  ( -45.39934640057513349, 26.50000000000019540, 10.49999999999999822 ) ) ;
#9275=ORIENTED_EDGE ( 'NONE', *, *, #5340, .T. ) ;
#9276=VECTOR ( 'NONE', #12174, 1000.000000000000000 ) ;
#9277=DIRECTION ( 'NONE',  ( 0.000000000000000000, 0.000000000000000000, 1.000000000000000000 ) ) ;
#9279=CARTESIAN_POINT ( 'NONE',  ( 0.000000000000000000, 0.000000000000000000, 8.000000000000000000 ) ) ;
#9280=CARTESIAN_POINT ( 'NONE',  ( -52.54657765281192638, 6.917888187662934563, 10.49999999999999822 ) ) ;
#9282=ORIENTED_EDGE ( 'NONE', *, *, #7417, .T. ) ;
#9283=DIRECTION ( 'NONE',  ( 0.000000000000000000, 0.000000000000000000, 1.000000000000000000 ) ) ;
#9284=EDGE_LOOP ( 'NONE', ( #11139, #13656, #4098, #4317, #14592, #6588, #4548, #5961, #2309, #13887 ) ) ;
#9286=CIRCLE ( 'NONE', #4935, 52.50000000000000711 ) ;
#9289=VERTEX_POINT ( 'NONE', #12312 ) ;
#9290=AXIS2_PLACEMENT_3D ( 'NONE', #6484, #14714, #4314 ) ;
#9292=CARTESIAN_POINT ( 'NONE',  ( -45.89934640057513349, 26.50000000000019540, -8.000000000000000000 ) ) ;
#9293=FACE_OUTER_BOUND ( 'NONE', #8044, .T. ) ;
#9294=CARTESIAN_POINT ( 'NONE',  ( -30.80502811811232888, -49.00442420935981147, -13.00000000000000178 ) ) ;
#9295=ORIENTED_EDGE ( 'NONE', *, *, #14991, .F. ) ;
#9296=AXIS2_PLACEMENT_3D ( 'NONE', #6771, #2155, #7995 ) ;
#9297=VERTEX_POINT ( 'NONE', #8880 ) ;
#9298=VERTEX_POINT ( 'NONE', #1898 ) ;
#9299=DIRECTION ( 'NONE',  ( 0.000000000000000000, 0.000000000000000000, -1.000000000000000000 ) ) ;
#9306=DIRECTION ( 'NONE',  ( 0.000000000000000000, 0.000000000000000000, 1.000000000000000000 ) ) ;
#9308=ADVANCED_FACE ( 'NONE', ( #13670 ), #12460, .F. ) ;
#9309=ADVANCED_FACE ( 'NONE', ( #4340 ), #6510, .F. ) ;
#9310=VERTEX_POINT ( 'NONE', #14814 ) ;
#9313=DIRECTION ( 'NONE',  ( 0.000000000000000000, 0.000000000000000000, 1.000000000000000000 ) ) ;
#9314=EDGE_CURVE ( 'NONE', #1107, #10590, #10926, .T. ) ;
#9315=ORIENTED_EDGE ( 'NONE', *, *, #12933, .F. ) ;
#9316=ORIENTED_EDGE ( 'NONE', *, *, #1067, .F. ) ;
#9317=DIRECTION ( 'NONE',  ( 0.000000000000000000, 0.000000000000000000, 1.000000000000000000 ) ) ;
#9318=CIRCLE ( 'NONE', #6391, 3.000000000000002665 ) ;
#9319=ADVANCED_FACE ( 'NONE', ( #926 ), #5314, .F. ) ;
#9323=DIRECTION ( 'NONE',  ( 0.000000000000000000, 0.000000000000000000, -1.000000000000000000 ) ) ;
#9326=CARTESIAN_POINT ( 'NONE',  ( 0.000000000000000000, 0.000000000000000000, 8.000000000000000000 ) ) ;
#9328=DIRECTION ( 'NONE',  ( 0.000000000000000000, 0.000000000000000000, 1.000000000000000000 ) ) ;
#9329=ORIENTED_EDGE ( 'NONE', *, *, #1435, .T. ) ;
#9330=AXIS2_PLACEMENT_3D ( 'NONE', #10889, #2921, #1788 ) ;
#9334=PLANE ( 'NONE',  #14764 ) ;
#9337=CARTESIAN_POINT ( 'NONE',  ( 30.80502811811196295, 49.00442420936003174, -10.50000000000000000 ) ) ;
#9339=CIRCLE ( 'NONE', #8855, 50.00000000000000000 ) ;
#9340=CARTESIAN_POINT ( 'NONE',  ( -12.86891638962156215, 56.43380494353993271, -13.00000000000000178 ) ) ;
#9341=CARTESIAN_POINT ( 'NONE',  ( -94.51066581171356518, -1.674280531758327140, -8.000000000000000000 ) ) ;
#9342=CARTESIAN_POINT ( 'NONE',  ( 0.000000000000000000, 0.000000000000000000, -8.000000000000000000 ) ) ;
#9346=CIRCLE ( 'NONE', #11052, 53.55662432702593634 ) ;
#9348=CIRCLE ( 'NONE', #5952, 3.000000000000002665 ) ;
#9349=ORIENTED_EDGE ( 'NONE', *, *, #7794, .F. ) ;
#9352=EDGE_CURVE ( 'NONE', #5870, #6495, #5831, .T. ) ;
#9353=EDGE_CURVE ( 'NONE', #4977, #8921, #1215, .T. ) ;
#9354=CARTESIAN_POINT ( 'NONE',  ( -39.30189486418265687, -33.47282819776598473, 8.000000000000000000 ) ) ;
#9356=ORIENTED_EDGE ( 'NONE', *, *, #1299, .T. ) ;
#9357=AXIS2_PLACEMENT_3D ( 'NONE', #2765, #7387, #9651 ) ;
#9359=ORIENTED_EDGE ( 'NONE', *, *, #2351, .T. ) ;
#9361=DIRECTION ( 'NONE',  ( 1.000000000000000000, 0.000000000000000000, 0.000000000000000000 ) ) ;
#9362=EDGE_CURVE ( 'NONE', #10605, #7502, #14584, .T. ) ;
#9364=CYLINDRICAL_SURFACE ( 'NONE', #9296, 60.50000000000000000 ) ;
#9365=ORIENTED_EDGE ( 'NONE', *, *, #9820, .F. ) ;
#9367=DIRECTION ( 'NONE',  ( 1.000000000000000000, 0.000000000000000000, 0.000000000000000000 ) ) ;
#9369=ADVANCED_FACE ( 'NONE', ( #3499 ), #10475, .F. ) ;
#9370=DIRECTION ( 'NONE',  ( -1.000000000000000000, 0.000000000000000000, 0.000000000000000000 ) ) ;
#9371=ORIENTED_EDGE ( 'NONE', *, *, #12727, .F. ) ;
#9372=ORIENTED_EDGE ( 'NONE', *, *, #11745, .F. ) ;
#9373=VERTEX_POINT ( 'NONE', #8122 ) ;
#9374=DIRECTION ( 'NONE',  ( 1.000000000000000000, 0.000000000000000000, 0.000000000000000000 ) ) ;
#9379=CARTESIAN_POINT ( 'NONE',  ( 97.00000000000000000, -3.384287605079545030E-13, 10.49999999999999822 ) ) ;
#9382=CARTESIAN_POINT ( 'NONE',  ( -45.89934640057513349, 26.50000000000019540, 10.49999999999999822 ) ) ;
#9384=DIRECTION ( 'NONE',  ( 0.000000000000000000, 0.000000000000000000, -1.000000000000000000 ) ) ;
#9385=ORIENTED_EDGE ( 'NONE', *, *, #3311, .F. ) ;
#9386=VERTEX_POINT ( 'NONE', #2283 ) ;
#9387=CARTESIAN_POINT ( 'NONE',  ( -37.71449950290985953, 86.67575032682117353, 8.000000000000000000 ) ) ;
#9391=FACE_OUTER_BOUND ( 'NONE', #14732, .T. ) ;
#9392=EDGE_CURVE ( 'NONE', #900, #1607, #9469, .T. ) ;
#9394=VERTEX_POINT ( 'NONE', #11562 ) ;
#9396=AXIS2_PLACEMENT_3D ( 'NONE', #2633, #14031, #1356 ) ;
#9397=CARTESIAN_POINT ( 'NONE',  ( 0.000000000000000000, 0.000000000000000000, 8.000000000000000000 ) ) ;
#9398=ORIENTED_EDGE ( 'NONE', *, *, #12481, .T. ) ;
#9400=ORIENTED_EDGE ( 'NONE', *, *, #5634, .F. ) ;
#9401=CARTESIAN_POINT ( 'NONE',  ( -53.20607447915234189, 6.117650515114558374, -10.50000000000000000 ) ) ;
#9402=ORIENTED_EDGE ( 'NONE', *, *, #6565, .T. ) ;
#9403=CARTESIAN_POINT ( 'NONE',  ( -68.58935777509427112, 68.58935777509594800, -13.00000000000000178 ) ) ;
#9405=EDGE_CURVE ( 'NONE', #8537, #12171, #2208, .T. ) ;
#9406=DIRECTION ( 'NONE',  ( -1.000000000000000000, 0.000000000000000000, 0.000000000000000000 ) ) ;
#9407=DIRECTION ( 'NONE',  ( 0.000000000000000000, 0.000000000000000000, 1.000000000000000000 ) ) ;
#9410=AXIS2_PLACEMENT_3D ( 'NONE', #9006, #12515, #8861 ) ;
#9413=DIRECTION ( 'NONE',  ( 0.000000000000000000, 0.000000000000000000, 1.000000000000000000 ) ) ;
#9414=ORIENTED_EDGE ( 'NONE', *, *, #4537, .F. ) ;
#9418=CARTESIAN_POINT ( 'NONE',  ( -29.49928053175900899, -45.83364790889059037, 8.000000000000000000 ) ) ;
#9419=ORIENTED_EDGE ( 'NONE', *, *, #10804, .T. ) ;
#9420=DIRECTION ( 'NONE',  ( 1.000000000000000000, 0.000000000000000000, 0.000000000000000000 ) ) ;
#9422=ORIENTED_EDGE ( 'NONE', *, *, #14136, .F. ) ;
#9423=DIRECTION ( 'NONE',  ( -1.000000000000000000, 5.335368001743792930E-15, 0.000000000000000000 ) ) ;
#9424=FACE_OUTER_BOUND ( 'NONE', #8920, .T. ) ;
#9426=CIRCLE ( 'NONE', #4835, 2.649999999999985700 ) ;
#9427=EDGE_CURVE ( 'NONE', #9900, #12050, #1077, .T. ) ;
#9429=EDGE_CURVE ( 'NONE', #5812, #14878, #7962, .T. ) ;
#9430=CARTESIAN_POINT ( 'NONE',  ( 22.33583958711425055, -30.74264578624780597, -28.00000000000000000 ) ) ;
#9431=EDGE_CURVE ( 'NONE', #2014, #10761, #5691, .T. ) ;
#9432=ORIENTED_EDGE ( 'NONE', *, *, #2354, .T. ) ;
#9433=DIRECTION ( 'NONE',  ( 0.000000000000000000, 0.000000000000000000, 1.000000000000000000 ) ) ;
#9434=DIRECTION ( 'NONE',  ( 0.000000000000000000, 0.000000000000000000, 1.000000000000000000 ) ) ;
#9435=DIRECTION ( 'NONE',  ( -1.000000000000000000, 0.000000000000000000, 0.000000000000000000 ) ) ;
#9436=ORIENTED_EDGE ( 'NONE', *, *, #8159, .F. ) ;
#9437=EDGE_CURVE ( 'NONE', #13133, #13337, #6801, .T. ) ;
#9439=CIRCLE ( 'NONE', #12610, 53.55662432702593634 ) ;
#9440=ORIENTED_EDGE ( 'NONE', *, *, #1664, .T. ) ;
#9441=VERTEX_POINT ( 'NONE', #7426 ) ;
#9443=AXIS2_PLACEMENT_3D ( 'NONE', #1545, #7297, #8444 ) ;
#9444=DIRECTION ( 'NONE',  ( -1.000000000000000000, 0.000000000000000000, 0.000000000000000000 ) ) ;
#9445=ADVANCED_FACE ( 'NONE', ( #3869 ), #301, .T. ) ;
#9449=FACE_OUTER_BOUND ( 'NONE', #14682, .T. ) ;
#9450=CIRCLE ( 'NONE', #1703, 0.5000000000000004441 ) ;
#9451=ORIENTED_EDGE ( 'NONE', *, *, #7268, .T. ) ;
#9452=AXIS2_PLACEMENT_3D ( 'NONE', #14192, #12000, #4780 ) ;
#9453=VERTEX_POINT ( 'NONE', #7345 ) ;
#9454=CARTESIAN_POINT ( 'NONE',  ( -97.00000000000000000, 1.015776140243522349E-12, -8.000000000000000000 ) ) ;
#9455=CARTESIAN_POINT ( 'NONE',  ( -68.09867107463028901, -68.49330278050098286, 10.49999999999999822 ) ) ;
#9456=CARTESIAN_POINT ( 'NONE',  ( 37.62029293941316155, -89.61631465359504034, 10.49999999999999822 ) ) ;
#9458=AXIS2_PLACEMENT_3D ( 'NONE', #3510, #6976, #11633 ) ;
#9459=ORIENTED_EDGE ( 'NONE', *, *, #4957, .F. ) ;
#9460=CARTESIAN_POINT ( 'NONE',  ( -45.89934640057513349, 26.50000000000019540, -8.000000000000000000 ) ) ;
#9461=CIRCLE ( 'NONE', #13109, 0.5000000000000038858 ) ;
#9462=ORIENTED_EDGE ( 'NONE', *, *, #13646, .T. ) ;
#9463=CIRCLE ( 'NONE', #2931, 50.00000000000000000 ) ;
#9464=AXIS2_PLACEMENT_3D ( 'NONE', #6047, #7262, #7423 ) ;
#9465=CARTESIAN_POINT ( 'NONE',  ( -42.50536573064432133, -32.06294366074479996, -13.00000000000000178 ) ) ;
#9466=DIRECTION ( 'NONE',  ( 0.000000000000000000, 0.000000000000000000, 1.000000000000000000 ) ) ;
#9469=CIRCLE ( 'NONE', #12638, 2.649999999999987477 ) ;
#9472=CARTESIAN_POINT ( 'NONE',  ( -91.27544013909712817, 39.61975340586647576, -8.000000000000000000 ) ) ;
#9474=CIRCLE ( 'NONE', #4403, 100.0000000000000000 ) ;
#9475=DIRECTION ( 'NONE',  ( -1.000000000000000000, 0.000000000000000000, 0.000000000000000000 ) ) ;
#9478=ORIENTED_EDGE ( 'NONE', *, *, #10150, .T. ) ;
#9479=VERTEX_POINT ( 'NONE', #5075 ) ;
#9480=CIRCLE ( 'NONE', #11688, 0.5000000000000004441 ) ;
#9481=DIRECTION ( 'NONE',  ( -1.000000000000000000, 0.000000000000000000, 0.000000000000000000 ) ) ;
#9484=CARTESIAN_POINT ( 'NONE',  ( -51.79945067148133120, -13.60620885621556475, -10.50000000000000000 ) ) ;
#9486=CARTESIAN_POINT ( 'NONE',  ( -57.06275842387042729, 9.706953719246069312, -10.50000000000000000 ) ) ;
#9488=ORIENTED_EDGE ( 'NONE', *, *, #11323, .F. ) ;
#9491=VERTEX_POINT ( 'NONE', #12005 ) ;
#9492=ADVANCED_FACE ( 'NONE', ( #1440 ), #8560, .F. ) ;
#9493=EDGE_CURVE ( 'NONE', #1639, #2908, #3666, .T. ) ;
#9494=ADVANCED_FACE ( 'NONE', ( #5015 ), #5158, .F. ) ;
#9495=DIRECTION ( 'NONE',  ( 0.000000000000000000, 0.000000000000000000, 1.000000000000000000 ) ) ;
#9496=DIRECTION ( 'NONE',  ( 0.000000000000000000, 0.000000000000000000, -1.000000000000000000 ) ) ;
#9497=CIRCLE ( 'NONE', #8767, 3.000000000000002665 ) ;
#9498=DIRECTION ( 'NONE',  ( 0.000000000000000000, 0.000000000000000000, 1.000000000000000000 ) ) ;
#9499=DIRECTION ( 'NONE',  ( 0.000000000000000000, 0.000000000000000000, 1.000000000000000000 ) ) ;
#9500=ORIENTED_EDGE ( 'NONE', *, *, #11221, .T. ) ;
#9502=DIRECTION ( 'NONE',  ( 0.000000000000000000, 0.000000000000000000, 1.000000000000000000 ) ) ;
#9503=ORIENTED_EDGE ( 'NONE', *, *, #13538, .F. ) ;
#9504=AXIS2_PLACEMENT_3D ( 'NONE', #4082, #6411, #738 ) ;
#9505=DIRECTION ( 'NONE',  ( -1.000000000000000000, 0.000000000000000000, 0.000000000000000000 ) ) ;
#9511=DIRECTION ( 'NONE',  ( 1.000000000000000000, 0.000000000000000000, 0.000000000000000000 ) ) ;
#9512=CARTESIAN_POINT ( 'NONE',  ( -23.49999999999971223, -45.89934640057541060, -13.00000000000000178 ) ) ;
#9513=AXIS2_PLACEMENT_3D ( 'NONE', #947, #11423, #1024 ) ;
#9514=CYLINDRICAL_SURFACE ( 'NONE', #7069, 59.49999999999999289 ) ;
#9519=VERTEX_POINT ( 'NONE', #14267 ) ;
#9520=EDGE_CURVE ( 'NONE', #4822, #10098, #13569, .T. ) ;
#9523=CARTESIAN_POINT ( 'NONE',  ( 29.49928053175900899, 45.83364790889059037, -13.00000000000000178 ) ) ;
#9526=ORIENTED_EDGE ( 'NONE', *, *, #14810, .F. ) ;
#9527=DIRECTION ( 'NONE',  ( -0.000000000000000000, -0.000000000000000000, 1.000000000000000000 ) ) ;
#9528=CARTESIAN_POINT ( 'NONE',  ( 0.000000000000000000, 0.000000000000000000, 8.000000000000000000 ) ) ;
#9529=AXIS2_PLACEMENT_3D ( 'NONE', #3458, #12569, #11437 ) ;
#9531=EDGE_LOOP ( 'NONE', ( #9947, #8458, #6933, #11818, #433 ) ) ;
#9532=ADVANCED_FACE ( 'NONE', ( #9689 ), #2729, .F. ) ;
#9533=EDGE_CURVE ( 'NONE', #3826, #10605, #8477, .T. ) ;
#9534=VERTEX_POINT ( 'NONE', #10846 ) ;
#9538=DIRECTION ( 'NONE',  ( 0.000000000000000000, 0.000000000000000000, -1.000000000000000000 ) ) ;
#9541=CARTESIAN_POINT ( 'NONE',  ( 0.000000000000000000, 0.000000000000000000, 8.000000000000000000 ) ) ;
#9542=( NAMED_UNIT ( * ) SI_UNIT ( $, .STERADIAN. ) SOLID_ANGLE_UNIT ( ) );
#9543=EDGE_CURVE ( 'NONE', #11817, #4331, #3159, .T. ) ;
#9545=DIRECTION ( 'NONE',  ( -1.000000000000000000, 0.000000000000000000, 0.000000000000000000 ) ) ;
#9548=CIRCLE ( 'NONE', #8587, 0.5000000000000004441 ) ;
#9549=VECTOR ( 'NONE', #1121, 1000.000000000000000 ) ;
#9550=VERTEX_POINT ( 'NONE', #14120 ) ;
#9551=CIRCLE ( 'NONE', #3024, 46.33974596215558961 ) ;
#9553=VERTEX_POINT ( 'NONE', #8345 ) ;
#9554=CARTESIAN_POINT ( 'NONE',  ( -12.86891638962156215, 56.43380494353993271, 8.000000000000000000 ) ) ;
#9556=ORIENTED_EDGE ( 'NONE', *, *, #7437, .T. ) ;
#9558=AXIS2_PLACEMENT_3D ( 'NONE', #5500, #11275, #12129 ) ;
#9559=ORIENTED_EDGE ( 'NONE', *, *, #1131, .F. ) ;
#9560=CARTESIAN_POINT ( 'NONE',  ( -50.00000000000000000, 0.000000000000000000, -13.00000000000000178 ) ) ;
#9561=DIRECTION ( 'NONE',  ( -1.000000000000000000, 0.000000000000000000, 0.000000000000000000 ) ) ;
#9562=DIRECTION ( 'NONE',  ( 1.000000000000000000, 0.000000000000000000, 0.000000000000000000 ) ) ;
#9563=AXIS2_PLACEMENT_3D ( 'NONE', #13039, #10675, #503 ) ;
#9564=CIRCLE ( 'NONE', #13701, 60.50000000000000000 ) ;
#9566=EDGE_LOOP ( 'NONE', ( #4301, #8759, #11910, #4182, #9163, #6701, #118, #11625, #7445, #10948, #13357, #5490 ) ) ;
#9569=DIRECTION ( 'NONE',  ( 1.000000000000000000, 0.000000000000000000, 0.000000000000000000 ) ) ;
#9570=CARTESIAN_POINT ( 'NONE',  ( -57.06275842387042729, 9.706953719246069312, 10.49999999999999822 ) ) ;
#9572=CARTESIAN_POINT ( 'NONE',  ( 57.06275842387049835, -9.706953719245678514, 8.000000000000000000 ) ) ;
#9575=ORIENTED_EDGE ( 'NONE', *, *, #14281, .T. ) ;
#9576=ADVANCED_FACE ( 'NONE', ( #13280 ), #2873, .T. ) ;
#9578=ORIENTED_EDGE ( 'NONE', *, *, #10192, .F. ) ;
#9580=ADVANCED_FACE ( 'NONE', ( #11849 ), #6051, .F. ) ;
#9581=FACE_OUTER_BOUND ( 'NONE', #5292, .T. ) ;
#9582=CIRCLE ( 'NONE', #10566, 55.00000000000000000 ) ;
#9583=CIRCLE ( 'NONE', #10808, 63.00000000000000000 ) ;
#9585=CYLINDRICAL_SURFACE ( 'NONE', #10526, 0.5000000000000004441 ) ;
#9586=VERTEX_POINT ( 'NONE', #5301 ) ;
#9587=FACE_OUTER_BOUND ( 'NONE', #1342, .T. ) ;
#9589=DIRECTION ( 'NONE',  ( 0.000000000000000000, 0.000000000000000000, 1.000000000000000000 ) ) ;
#9591=VECTOR ( 'NONE', #12332, 1000.000000000000000 ) ;
#9594=DIRECTION ( 'NONE',  ( 0.000000000000000000, 0.000000000000000000, -1.000000000000000000 ) ) ;
#9595=ORIENTED_EDGE ( 'NONE', *, *, #5791, .F. ) ;
#9597=EDGE_CURVE ( 'NONE', #9719, #8562, #232, .T. ) ;
#9598=LINE ( 'NONE', #1492, #11973 ) ;
#9600=CARTESIAN_POINT ( 'NONE',  ( 23.50071946824041191, 45.96504489226015977, -8.000000000000000000 ) ) ;
#9601=AXIS2_PLACEMENT_3D ( 'NONE', #4214, #13247, #11193 ) ;
#9602=ORIENTED_EDGE ( 'NONE', *, *, #11408, .F. ) ;
#9604=CARTESIAN_POINT ( 'NONE',  ( 89.12622059913255157, 37.21932736666302333, -13.00000000000000178 ) ) ;
#9605=CARTESIAN_POINT ( 'NONE',  ( 52.54657765281197612, -6.917888187662545540, -13.00000000000000178 ) ) ;
#9607=ORIENTED_EDGE ( 'NONE', *, *, #10831, .T. ) ;
#9608=VERTEX_POINT ( 'NONE', #1961 ) ;
#9609=PLANE ( 'NONE',  #9835 ) ;
#9610=ORIENTED_EDGE ( 'NONE', *, *, #8976, .F. ) ;
#9611=DIRECTION ( 'NONE',  ( 0.000000000000000000, 0.000000000000000000, 1.000000000000000000 ) ) ;
#9612=DIRECTION ( 'NONE',  ( -1.000000000000000000, 0.000000000000000000, 0.000000000000000000 ) ) ;
#9613=EDGE_CURVE ( 'NONE', #4454, #10864, #14799, .T. ) ;
#9615=DIRECTION ( 'NONE',  ( 0.000000000000000000, 0.000000000000000000, 1.000000000000000000 ) ) ;
#9619=DIRECTION ( 'NONE',  ( 1.000000000000000000, 0.000000000000000000, 0.000000000000000000 ) ) ;
#9620=EDGE_CURVE ( 'NONE', #10362, #7077, #1216, .T. ) ;
#9621=EDGE_LOOP ( 'NONE', ( #8183, #13301, #9627, #12302, #6009 ) ) ;
#9623=DIRECTION ( 'NONE',  ( -1.000000000000000000, 0.000000000000000000, 0.000000000000000000 ) ) ;
#9624=EDGE_CURVE ( 'NONE', #915, #11561, #4120, .T. ) ;
#9625=ORIENTED_EDGE ( 'NONE', *, *, #12757, .F. ) ;
#9627=ORIENTED_EDGE ( 'NONE', *, *, #13352, .F. ) ;
#9628=CARTESIAN_POINT ( 'NONE',  ( 22.33583958711425055, -30.74264578624780597, -25.50000000000000355 ) ) ;
#9630=FACE_OUTER_BOUND ( 'NONE', #6632, .T. ) ;
#9631=CARTESIAN_POINT ( 'NONE',  ( 37.12029293941379393, 89.61631465359479876, 8.000000000000000000 ) ) ;
#9632=DIRECTION ( 'NONE',  ( -1.000000000000000000, 0.000000000000000000, 0.000000000000000000 ) ) ;
#9634=ORIENTED_EDGE ( 'NONE', *, *, #8593, .F. ) ;
#9637=DIRECTION ( 'NONE',  ( 0.000000000000000000, 0.000000000000000000, 1.000000000000000000 ) ) ;
#9639=CARTESIAN_POINT ( 'NONE',  ( -26.99988008862626643, -45.88839665196127271, 10.49999999999999822 ) ) ;
#9640=DIRECTION ( 'NONE',  ( 1.000000000000000000, 0.000000000000000000, 0.000000000000000000 ) ) ;
#9641=ORIENTED_EDGE ( 'NONE', *, *, #9759, .F. ) ;
#9644=CYLINDRICAL_SURFACE ( 'NONE', #6529, 20.00000000000000000 ) ;
#9645=CARTESIAN_POINT ( 'NONE',  ( 4.121772567811984089, 51.45950017607689375, 8.000000000000000000 ) ) ;
#9649=ORIENTED_EDGE ( 'NONE', *, *, #7922, .T. ) ;
#9650=ORIENTED_EDGE ( 'NONE', *, *, #12098, .F. ) ;
#9651=DIRECTION ( 'NONE',  ( 1.000000000000000000, 0.000000000000000000, 0.000000000000000000 ) ) ;
#9652=CARTESIAN_POINT ( 'NONE',  ( 33.48561063518626923, -47.21331623427104063, -13.00000000000000178 ) ) ;
#9654=EDGE_CURVE ( 'NONE', #12743, #5953, #10085, .T. ) ;
#9656=VERTEX_POINT ( 'NONE', #11150 ) ;
#9658=CIRCLE ( 'NONE', #10157, 60.50000000000000000 ) ;
#9659=ORIENTED_EDGE ( 'NONE', *, *, #10242, .F. ) ;
#9661=DIRECTION ( 'NONE',  ( 0.000000000000000000, 0.000000000000000000, -1.000000000000000000 ) ) ;
#9664=CARTESIAN_POINT ( 'NONE',  ( 96.58511096861892042, 0.2790467552928839190, -10.50000000000000000 ) ) ;
#9666=EDGE_LOOP ( 'NONE', ( #4941, #152, #2774, #1932, #2787 ) ) ;
#9667=LINE ( 'NONE', #9604, #10290 ) ;
#9670=CARTESIAN_POINT ( 'NONE',  ( 42.04772703543530099, 32.26435573746242369, -13.00000000000000178 ) ) ;
#9671=ADVANCED_FACE ( 'NONE', ( #757 ), #14650, .T. ) ;
#9674=ORIENTED_EDGE ( 'NONE', *, *, #593, .F. ) ;
#9675=CARTESIAN_POINT ( 'NONE',  ( -12.86891638962156215, 56.43380494353993271, -10.50000000000000000 ) ) ;
#9676=EDGE_CURVE ( 'NONE', #13408, #8680, #14494, .T. ) ;
#9678=AXIS2_PLACEMENT_3D ( 'NONE', #9798, #5182, #13083 ) ;
#9679=AXIS2_PLACEMENT_3D ( 'NONE', #12942, #2533, #7155 ) ;
#9680=DIRECTION ( 'NONE',  ( -1.000000000000000000, 0.000000000000000000, 0.000000000000000000 ) ) ;
#9681=CIRCLE ( 'NONE', #7504, 3.000000000000004441 ) ;
#9682=AXIS2_PLACEMENT_3D ( 'NONE', #10017, #4190, #8943 ) ;
#9683=DIRECTION ( 'NONE',  ( 0.000000000000000000, 0.000000000000000000, -1.000000000000000000 ) ) ;
#9684=( LENGTH_UNIT ( ) NAMED_UNIT ( * ) SI_UNIT ( .MILLI., .METRE. ) );
#9689=FACE_OUTER_BOUND ( 'NONE', #11541, .T. ) ;
#9690=AXIS2_PLACEMENT_3D ( 'NONE', #7495, #8568, #10780 ) ;
#9693=CONICAL_SURFACE ( 'NONE', #748, 55.00000000000000000, 0.5235987755983000369 ) ;
#9694=VERTEX_POINT ( 'NONE', #6374 ) ;
#9695=DIRECTION ( 'NONE',  ( 0.000000000000000000, 0.000000000000000000, -1.000000000000000000 ) ) ;
#9697=ORIENTED_EDGE ( 'NONE', *, *, #4600, .F. ) ;
#9698=CARTESIAN_POINT ( 'NONE',  ( -32.26435573746199736, 42.04772703543562073, -13.00000000000000178 ) ) ;
#9699=AXIS2_PLACEMENT_3D ( 'NONE', #9784, #8504, #2885 ) ;
#9701=CARTESIAN_POINT ( 'NONE',  ( 52.54657765281197612, -6.917888187662545540, -8.000000000000000000 ) ) ;
#9702=FACE_OUTER_BOUND ( 'NONE', #292, .T. ) ;
#9705=CARTESIAN_POINT ( 'NONE',  ( 13.71740939043365337, -51.19406879332061067, -8.000000000000000000 ) ) ;
#9706=CIRCLE ( 'NONE', #1964, 2.649999999999985700 ) ;
#9707=ORIENTED_EDGE ( 'NONE', *, *, #13235, .F. ) ;
#9709=ORIENTED_EDGE ( 'NONE', *, *, #4455, .F. ) ;
#9710=CARTESIAN_POINT ( 'NONE',  ( 9.706953719245472456, 57.06275842387054098, -10.50000000000000000 ) ) ;
#9711=LINE ( 'NONE', #7214, #6606 ) ;
#9715=AXIS2_PLACEMENT_3D ( 'NONE', #13243, #8592, #1774 ) ;
#9716=EDGE_CURVE ( 'NONE', #5988, #3770, #9875, .T. ) ;
#9718=EDGE_CURVE ( 'NONE', #8383, #9852, #3884, .T. ) ;
#9719=VERTEX_POINT ( 'NONE', #7375 ) ;
#9720=LINE ( 'NONE', #13159, #2171 ) ;
#9721=ORIENTED_EDGE ( 'NONE', *, *, #4818, .F. ) ;
#9722=DIRECTION ( 'NONE',  ( -0.000000000000000000, -0.000000000000000000, -1.000000000000000000 ) ) ;
#9723=CARTESIAN_POINT ( 'NONE',  ( 56.43380494353997534, 12.86891638962136319, -10.50000000000000000 ) ) ;
#9724=CIRCLE ( 'NONE', #775, 0.5000000000000022204 ) ;
#9725=DIRECTION ( 'NONE',  ( 1.000000000000000000, -9.769962616701375978E-15, 0.000000000000000000 ) ) ;
#9727=EDGE_CURVE ( 'NONE', #8393, #8383, #10907, .T. ) ;
#9728=CARTESIAN_POINT ( 'NONE',  ( -33.48561063518626923, 47.21331623427104063, -10.50000000000000000 ) ) ;
#9729=EDGE_LOOP ( 'NONE', ( #9595, #5234, #9975, #2318 ) ) ;
#9730=VECTOR ( 'NONE', #9466, 1000.000000000000000 ) ;
#9732=CARTESIAN_POINT ( 'NONE',  ( -37.12029293941250074, 89.61631465359532456, -13.00000000000000178 ) ) ;
#9734=DIRECTION ( 'NONE',  ( 1.000000000000000000, 0.000000000000000000, 0.000000000000000000 ) ) ;
#9735=AXIS2_PLACEMENT_3D ( 'NONE', #8386, #13250, #10655 ) ;
#9736=ORIENTED_EDGE ( 'NONE', *, *, #12561, .F. ) ;
#9737=DIRECTION ( 'NONE',  ( -1.000000000000000000, 0.000000000000000000, 0.000000000000000000 ) ) ;
#9738=VERTEX_POINT ( 'NONE', #14288 ) ;
#9739=AXIS2_PLACEMENT_3D ( 'NONE', #13016, #333, #4971 ) ;
#9740=DIRECTION ( 'NONE',  ( -1.000000000000000000, 0.000000000000000000, 0.000000000000000000 ) ) ;
#9741=PLANE ( 'NONE',  #6094 ) ;
#9742=ORIENTED_EDGE ( 'NONE', *, *, #12478, .F. ) ;
#9743=CARTESIAN_POINT ( 'NONE',  ( -32.46576781417928714, 41.59008834022678514, -10.50000000000000000 ) ) ;
#9744=DIRECTION ( 'NONE',  ( 1.000000000000000000, 0.000000000000000000, 0.000000000000000000 ) ) ;
#9745=DIRECTION ( 'NONE',  ( -1.000000000000000000, 0.000000000000000000, 0.000000000000000000 ) ) ;
#9746=EDGE_LOOP ( 'NONE', ( #13691, #6135 ) ) ;
#9748=DIRECTION ( 'NONE',  ( -1.000000000000000000, 0.000000000000000000, 0.000000000000000000 ) ) ;
#9749=DIRECTION ( 'NONE',  ( 1.000000000000000000, 0.000000000000000000, 0.000000000000000000 ) ) ;
#9751=ORIENTED_EDGE ( 'NONE', *, *, #4545, .T. ) ;
#9753=VERTEX_POINT ( 'NONE', #13013 ) ;
#9754=CARTESIAN_POINT ( 'NONE',  ( -26.49999999999971578, -45.89934640057541060, -8.000000000000000000 ) ) ;
#9755=ORIENTED_EDGE ( 'NONE', *, *, #8325, .F. ) ;
#9756=AXIS2_PLACEMENT_3D ( 'NONE', #8511, #14285, #8292 ) ;
#9757=DIRECTION ( 'NONE',  ( 1.000000000000000000, 0.000000000000000000, 0.000000000000000000 ) ) ;
#9758=EDGE_CURVE ( 'NONE', #5520, #8464, #7010, .T. ) ;
#9759=EDGE_CURVE ( 'NONE', #2920, #8250, #482, .T. ) ;
#9760=CARTESIAN_POINT ( 'NONE',  ( -43.30127018922181037, 25.00000000000021672, -8.000000000000000000 ) ) ;
#9762=EDGE_CURVE ( 'NONE', #8164, #11760, #3644, .T. ) ;
#9763=AXIS2_PLACEMENT_3D ( 'NONE', #11661, #10207, #12720 ) ;
#9764=DIRECTION ( 'NONE',  ( -1.000000000000000000, 0.000000000000000000, 0.000000000000000000 ) ) ;
#9765=DIRECTION ( 'NONE',  ( 0.000000000000000000, 0.000000000000000000, 1.000000000000000000 ) ) ;
#9767=DIRECTION ( 'NONE',  ( 1.000000000000000000, 0.000000000000000000, 0.000000000000000000 ) ) ;
#9768=AXIS2_PLACEMENT_3D ( 'NONE', #6118, #3708, #8407 ) ;
#9769=ORIENTED_EDGE ( 'NONE', *, *, #6464, .F. ) ;
#9770=VERTEX_POINT ( 'NONE', #1687 ) ;
#9771=CARTESIAN_POINT ( 'NONE',  ( 33.48561063518626923, -47.21331623427104063, -8.000000000000000000 ) ) ;
#9773=EDGE_LOOP ( 'NONE', ( #1151, #5283, #12730, #9282 ) ) ;
#9774=AXIS2_PLACEMENT_3D ( 'NONE', #13307, #12258, #1848 ) ;
#9775=CARTESIAN_POINT ( 'NONE',  ( -31.05588327715806329, 44.79355920668842828, 8.000000000000000000 ) ) ;
#9777=CARTESIAN_POINT ( 'NONE',  ( 0.000000000000000000, 0.000000000000000000, -10.50000000000000000 ) ) ;
#9778=CARTESIAN_POINT ( 'NONE',  ( 6.917888187663118416, 52.54657765281190507, -13.00000000000000178 ) ) ;
#9779=EDGE_CURVE ( 'NONE', #13295, #8252, #9720, .T. ) ;
#9780=DIRECTION ( 'NONE',  ( 1.000000000000000000, 0.000000000000000000, 0.000000000000000000 ) ) ;
#9781=ORIENTED_EDGE ( 'NONE', *, *, #10386, .F. ) ;
#9783=AXIS2_PLACEMENT_3D ( 'NONE', #6490, #9844, #14488 ) ;
#9784=CARTESIAN_POINT ( 'NONE',  ( 30.80502811811196295, 49.00442420936003174, -10.50000000000000000 ) ) ;
#9785=CIRCLE ( 'NONE', #3262, 59.50000000000000000 ) ;
#9786=LINE ( 'NONE', #12445, #4562 ) ;
#9788=CARTESIAN_POINT ( 'NONE',  ( 37.12029293941315444, -89.61631465359504034, 10.49999999999999822 ) ) ;
#9789=DIRECTION ( 'NONE',  ( 0.000000000000000000, 0.000000000000000000, -1.000000000000000000 ) ) ;
#9790=ORIENTED_EDGE ( 'NONE', *, *, #11323, .T. ) ;
#9793=CIRCLE ( 'NONE', #11284, 3.000000000000002665 ) ;
#9794=DIRECTION ( 'NONE',  ( 0.000000000000000000, 0.000000000000000000, 1.000000000000000000 ) ) ;
#9795=ORIENTED_EDGE ( 'NONE', *, *, #10515, .F. ) ;
#9796=VECTOR ( 'NONE', #13030, 1000.000000000000000 ) ;
#9797=VECTOR ( 'NONE', #1480, 1000.000000000000000 ) ;
#9798=CARTESIAN_POINT ( 'NONE',  ( 0.000000000000000000, 0.000000000000000000, 8.000000000000000000 ) ) ;
#9799=CIRCLE ( 'NONE', #9081, 0.5000000000000043299 ) ;
#9800=ORIENTED_EDGE ( 'NONE', *, *, #8709, .T. ) ;
#9802=CYLINDRICAL_SURFACE ( 'NONE', #2421, 3.000000000000002665 ) ;
#9805=DIRECTION ( 'NONE',  ( -1.000000000000000000, 0.000000000000000000, 0.000000000000000000 ) ) ;
#9806=DIRECTION ( 'NONE',  ( -0.000000000000000000, -0.000000000000000000, -1.000000000000000000 ) ) ;
#9807=EDGE_CURVE ( 'NONE', #7876, #669, #14547, .T. ) ;
#9808=VECTOR ( 'NONE', #14443, 1000.000000000000000 ) ;
#9810=EDGE_CURVE ( 'NONE', #8471, #4116, #5328, .T. ) ;
#9811=CIRCLE ( 'NONE', #12501, 63.00000000000000000 ) ;
#9812=CARTESIAN_POINT ( 'NONE',  ( 47.21331623427115431, 33.48561063518610581, -10.50000000000000000 ) ) ;
#9813=CYLINDRICAL_SURFACE ( 'NONE', #850, 56.99999999999999289 ) ;
#9814=VECTOR ( 'NONE', #14886, 1000.000000000000000 ) ;
#9817=ORIENTED_EDGE ( 'NONE', *, *, #3411, .T. ) ;
#9819=ORIENTED_EDGE ( 'NONE', *, *, #5816, .F. ) ;
#9820=EDGE_CURVE ( 'NONE', #1055, #12316, #14447, .T. ) ;
#9822=CIRCLE ( 'NONE', #3789, 0.5000000000000004441 ) ;
#9824=CARTESIAN_POINT ( 'NONE',  ( -52.50000000000000711, 0.000000000000000000, -13.00000000000000178 ) ) ;
#9831=ADVANCED_FACE ( 'NONE', ( #7446 ), #12095, .F. ) ;
#9833=DIRECTION ( 'NONE',  ( -1.000000000000000000, 1.065814103640150279E-14, 0.000000000000000000 ) ) ;
#9834=DIRECTION ( 'NONE',  ( -0.000000000000000000, -0.000000000000000000, 1.000000000000000000 ) ) ;
#9835=AXIS2_PLACEMENT_3D ( 'NONE', #2404, #12750, #3858 ) ;
#9836=DIRECTION ( 'NONE',  ( 0.000000000000000000, 0.000000000000000000, 1.000000000000000000 ) ) ;
#9837=ORIENTED_EDGE ( 'NONE', *, *, #2631, .T. ) ;
#9839=FACE_OUTER_BOUND ( 'NONE', #6259, .T. ) ;
#9841=CIRCLE ( 'NONE', #4521, 3.000000000000002665 ) ;
#9844=DIRECTION ( 'NONE',  ( 0.000000000000000000, 0.000000000000000000, -1.000000000000000000 ) ) ;
#9845=ORIENTED_EDGE ( 'NONE', *, *, #5903, .T. ) ;
#9848=ORIENTED_EDGE ( 'NONE', *, *, #3345, .F. ) ;
#9849=VECTOR ( 'NONE', #5379, 1000.000000000000000 ) ;
#9852=VERTEX_POINT ( 'NONE', #8813 ) ;
#9853=ORIENTED_EDGE ( 'NONE', *, *, #4743, .T. ) ;
#9856=EDGE_CURVE ( 'NONE', #7413, #4919, #13326, .T. ) ;
#9858=CARTESIAN_POINT ( 'NONE',  ( -6.917888187662729393, -52.54657765281195481, 8.000000000000000000 ) ) ;
#9860=DIRECTION ( 'NONE',  ( 0.000000000000000000, 0.000000000000000000, -1.000000000000000000 ) ) ;
#9861=CARTESIAN_POINT ( 'NONE',  ( 92.55687898036906347, 36.52608637591612961, -13.00000000000000178 ) ) ;
#9863=ORIENTED_EDGE ( 'NONE', *, *, #9870, .F. ) ;
#9864=LINE ( 'NONE', #6880, #9873 ) ;
#9865=EDGE_CURVE ( 'NONE', #2732, #132, #2662, .T. ) ;
#9866=DIRECTION ( 'NONE',  ( 1.000000000000000000, 0.000000000000000000, 0.000000000000000000 ) ) ;
#9869=DIRECTION ( 'NONE',  ( 0.000000000000000000, 0.000000000000000000, 1.000000000000000000 ) ) ;
#9870=EDGE_CURVE ( 'NONE', #14678, #7442, #3654, .T. ) ;
#9871=ORIENTED_EDGE ( 'NONE', *, *, #8649, .T. ) ;
#9872=LINE ( 'NONE', #11101, #11261 ) ;
#9873=VECTOR ( 'NONE', #913, 1000.000000000000000 ) ;
#9875=LINE ( 'NONE', #633, #6038 ) ;
#9876=ORIENTED_EDGE ( 'NONE', *, *, #10554, .T. ) ;
#9877=DIRECTION ( 'NONE',  ( 0.000000000000000000, 0.000000000000000000, 1.000000000000000000 ) ) ;
#9878=CARTESIAN_POINT ( 'NONE',  ( 11.55014193876178297, -53.26842454702432406, -8.000000000000000000 ) ) ;
#9880=CARTESIAN_POINT ( 'NONE',  ( -9.706953719245875689, -57.06275842387046993, 10.49999999999999822 ) ) ;
#9882=DIRECTION ( 'NONE',  ( 0.000000000000000000, 0.000000000000000000, -1.000000000000000000 ) ) ;
#9883=AXIS2_PLACEMENT_3D ( 'NONE', #9528, #14178, #3627 ) ;
#9885=DIRECTION ( 'NONE',  ( 1.000000000000000000, 0.000000000000000000, 0.000000000000000000 ) ) ;
#9887=CYLINDRICAL_SURFACE ( 'NONE', #813, 0.5000000000000004441 ) ;
#9888=VERTEX_POINT ( 'NONE', #13681 ) ;
#9889=CARTESIAN_POINT ( 'NONE',  ( 0.000000000000000000, 0.000000000000000000, 8.000000000000000000 ) ) ;
#9890=EDGE_CURVE ( 'NONE', #10669, #2752, #11163, .T. ) ;
#9891=ADVANCED_FACE ( 'NONE', ( #13524 ), #862, .T. ) ;
#9892=VERTEX_POINT ( 'NONE', #8734 ) ;
#9893=EDGE_CURVE ( 'NONE', #1264, #14119, #2427, .T. ) ;
#9897=CARTESIAN_POINT ( 'NONE',  ( -33.48561063518626923, 47.21331623427104063, -10.50000000000000000 ) ) ;
#9900=VERTEX_POINT ( 'NONE', #3129 ) ;
#9901=VERTEX_POINT ( 'NONE', #5325 ) ;
#9902=ORIENTED_EDGE ( 'NONE', *, *, #11333, .F. ) ;
#9903=ADVANCED_FACE ( 'NONE', ( #12547 ), #14603, .F. ) ;
#9905=DIRECTION ( 'NONE',  ( 0.000000000000000000, 0.000000000000000000, -1.000000000000000000 ) ) ;
#9906=CARTESIAN_POINT ( 'NONE',  ( 53.26842454702428142, 11.55014193876197126, -13.00000000000000178 ) ) ;
#9907=ORIENTED_EDGE ( 'NONE', *, *, #8142, .F. ) ;
#9911=EDGE_CURVE ( 'NONE', #2565, #14269, #6522, .T. ) ;
#9913=ADVANCED_FACE ( 'NONE', ( #6747 ), #13456, .F. ) ;
#9914=CARTESIAN_POINT ( 'NONE',  ( -30.80502811811232888, -49.00442420935981147, -13.00000000000000178 ) ) ;
#9916=CARTESIAN_POINT ( 'NONE',  ( 0.000000000000000000, 0.000000000000000000, -8.000000000000000000 ) ) ;
#9918=CARTESIAN_POINT ( 'NONE',  ( -1.674280531759324342, -99.48933418828643482, -8.000000000000000000 ) ) ;
#9919=CIRCLE ( 'NONE', #7978, 52.50000000000000711 ) ;
#9920=ORIENTED_EDGE ( 'NONE', *, *, #3480, .T. ) ;
#9921=DIRECTION ( 'NONE',  ( 0.000000000000000000, 0.000000000000000000, 1.000000000000000000 ) ) ;
#9922=CARTESIAN_POINT ( 'NONE',  ( 86.67575032682076142, 37.71449950291080455, -8.000000000000000000 ) ) ;
#9925=ORIENTED_EDGE ( 'NONE', *, *, #9597, .T. ) ;
#9927=AXIS2_PLACEMENT_3D ( 'NONE', #13428, #6578, #11233 ) ;
#9928=ORIENTED_EDGE ( 'NONE', *, *, #11408, .T. ) ;
#9931=CIRCLE ( 'NONE', #9682, 60.50000000000000000 ) ;
#9932=CARTESIAN_POINT ( 'NONE',  ( 0.000000000000000000, 0.000000000000000000, 8.000000000000000000 ) ) ;
#9933=CARTESIAN_POINT ( 'NONE',  ( 0.000000000000000000, 0.000000000000000000, -8.000000000000000000 ) ) ;
#9934=DIRECTION ( 'NONE',  ( 0.000000000000000000, 0.000000000000000000, 1.000000000000000000 ) ) ;
#9936=AXIS2_PLACEMENT_3D ( 'NONE', #12470, #6600, #12251 ) ;
#9937=CARTESIAN_POINT ( 'NONE',  ( -33.47282819776587814, 39.30189486418276346, 8.000000000000000000 ) ) ;
#9938=ORIENTED_EDGE ( 'NONE', *, *, #10427, .T. ) ;
#9939=AXIS2_PLACEMENT_3D ( 'NONE', #10038, #4432, #1993 ) ;
#9940=ADVANCED_FACE ( 'NONE', ( #7824 ), #4349, .T. ) ;
#9941=AXIS2_PLACEMENT_3D ( 'NONE', #7299, #10805, #6086 ) ;
#9943=VERTEX_POINT ( 'NONE', #14752 ) ;
#9944=MECHANICAL_DESIGN_GEOMETRIC_PRESENTATION_REPRESENTATION('',(#13589),#502);
#9945=DIRECTION ( 'NONE',  ( 0.000000000000000000, 0.000000000000000000, -1.000000000000000000 ) ) ;
#9946=CARTESIAN_POINT ( 'NONE',  ( -97.00000000000000000, 1.015776140243522349E-12, -13.00000000000000178 ) ) ;
#9947=ORIENTED_EDGE ( 'NONE', *, *, #5878, .T. ) ;
#9950=AXIS2_PLACEMENT_3D ( 'NONE', #1286, #3410, #5900 ) ;
#9951=CARTESIAN_POINT ( 'NONE',  ( 0.000000000000000000, 0.000000000000000000, -28.00000000000000000 ) ) ;
#9953=CARTESIAN_POINT ( 'NONE',  ( -51.19406879332065330, -13.71740939043347041, 8.000000000000000000 ) ) ;
#9956=AXIS2_PLACEMENT_3D ( 'NONE', #10997, #3945, #6266 ) ;
#9957=CARTESIAN_POINT ( 'NONE',  ( -51.19406879332065330, -13.71740939043347041, -13.00000000000000178 ) ) ;
#9958=DIRECTION ( 'NONE',  ( 0.000000000000000000, 0.000000000000000000, 1.000000000000000000 ) ) ;
#9960=CARTESIAN_POINT ( 'NONE',  ( -52.54657765281192638, 6.917888187662934563, -13.00000000000000178 ) ) ;
#9961=EDGE_CURVE ( 'NONE', #5756, #7182, #11179, .T. ) ;
#9962=PLANE ( 'NONE',  #9774 ) ;
#9963=EDGE_CURVE ( 'NONE', #12145, #13693, #1009, .T. ) ;
#9966=CIRCLE ( 'NONE', #13861, 3.000000000000002665 ) ;
#9967=ORIENTED_EDGE ( 'NONE', *, *, #10753, .F. ) ;
#9969=AXIS2_PLACEMENT_3D ( 'NONE', #10223, #6870, #10302 ) ;
#9970=CARTESIAN_POINT ( 'NONE',  ( -39.66766701456180755, -30.43807145043597728, 8.000000000000000000 ) ) ;
#9971=CIRCLE ( 'NONE', #2941, 63.00000000000000000 ) ;
#9972=CARTESIAN_POINT ( 'NONE',  ( -2.449293598294708880E-16, 38.00000000000000000, -25.50000000000000355 ) ) ;
#9973=EDGE_CURVE ( 'NONE', #3062, #3301, #11422, .T. ) ;
#9975=ORIENTED_EDGE ( 'NONE', *, *, #13676, .F. ) ;
#9976=APPLICATION_CONTEXT ( 'automotive_design' ) ;
#9977=DIRECTION ( 'NONE',  ( -1.000000000000000000, 4.163336342344304841E-14, 0.000000000000000000 ) ) ;
#9979=DIRECTION ( 'NONE',  ( 1.000000000000000000, 0.000000000000000000, 0.000000000000000000 ) ) ;
#9980=DIRECTION ( 'NONE',  ( -0.000000000000000000, -0.000000000000000000, 1.000000000000000000 ) ) ;
#9981=CIRCLE ( 'NONE', #11970, 0.5000000000000004441 ) ;
#9982=CARTESIAN_POINT ( 'NONE',  ( -9.714003807513870825, -53.63365512954690217, 8.000000000000000000 ) ) ;
#9983=CIRCLE ( 'NONE', #14851, 3.000000000000002665 ) ;
#9984=DIRECTION ( 'NONE',  ( -1.000000000000000000, 0.000000000000000000, 0.000000000000000000 ) ) ;
#9986=EDGE_LOOP ( 'NONE', ( #7164, #13377, #12001, #2874, #11199 ) ) ;
#9987=EDGE_LOOP ( 'NONE', ( #13052, #6540, #7233, #9650, #11228, #3995 ) ) ;
#9989=CARTESIAN_POINT ( 'NONE',  ( -29.49928053175900899, -45.83364790889059037, -8.000000000000000000 ) ) ;
#9990=AXIS2_PLACEMENT_3D ( 'NONE', #11095, #4420, #7893 ) ;
#9994=VERTEX_POINT ( 'NONE', #9118 ) ;
#9996=ORIENTED_EDGE ( 'NONE', *, *, #13575, .T. ) ;
#9999=CARTESIAN_POINT ( 'NONE',  ( 50.13108361037843252, 56.43380494353993271, 8.000000000000000000 ) ) ;
#10001=ORIENTED_EDGE ( 'NONE', *, *, #6890, .F. ) ;
#10004=VERTEX_POINT ( 'NONE', #2426 ) ;
#10008=ORIENTED_EDGE ( 'NONE', *, *, #9392, .F. ) ;
#10009=VECTOR ( 'NONE', #7531, 1000.000000000000000 ) ;
#10010=ORIENTED_EDGE ( 'NONE', *, *, #4678, .T. ) ;
#10012=DIRECTION ( 'NONE',  ( 0.000000000000000000, 0.000000000000000000, 1.000000000000000000 ) ) ;
#10013=EDGE_CURVE ( 'NONE', #10294, #11817, #3653, .T. ) ;
#10016=CARTESIAN_POINT ( 'NONE',  ( 49.00442420935993226, -30.80502811811213704, 10.49999999999999822 ) ) ;
#10017=CARTESIAN_POINT ( 'NONE',  ( -12.86891638962156215, 56.43380494353993271, -10.50000000000000000 ) ) ;
#10018=CARTESIAN_POINT ( 'NONE',  ( 0.000000000000000000, 0.000000000000000000, 8.000000000000000000 ) ) ;
#10019=CONICAL_SURFACE ( 'NONE', #5424, 52.83493649053890806, 0.5235987755983000369 ) ;
#10020=ORIENTED_EDGE ( 'NONE', *, *, #1167, .F. ) ;
#10021=CARTESIAN_POINT ( 'NONE',  ( 0.000000000000000000, 0.000000000000000000, -13.00000000000000178 ) ) ;
#10023=DIRECTION ( 'NONE',  ( 0.000000000000000000, 0.000000000000000000, -1.000000000000000000 ) ) ;
#10025=ORIENTED_EDGE ( 'NONE', *, *, #1834, .F. ) ;
#10026=LINE ( 'NONE', #8884, #9808 ) ;
#10027=LINE ( 'NONE', #10946, #14656 ) ;
#10029=CARTESIAN_POINT ( 'NONE',  ( 51.53979475227119167, 13.35619814848851483, -13.00000000000000178 ) ) ;
#10031=ORIENTED_EDGE ( 'NONE', *, *, #6900, .F. ) ;
#10032=DIRECTION ( 'NONE',  ( 1.000000000000000000, 0.000000000000000000, 0.000000000000000000 ) ) ;
#10033=CARTESIAN_POINT ( 'NONE',  ( 45.89934640057532533, -26.49999999999987566, 8.000000000000000000 ) ) ;
#10034=DIRECTION ( 'NONE',  ( 1.000000000000000000, 0.000000000000000000, 0.000000000000000000 ) ) ;
#10035=CIRCLE ( 'NONE', #2515, 3.000000000000002665 ) ;
#10038=CARTESIAN_POINT ( 'NONE',  ( -33.48561063518626923, 47.21331623427104063, 10.49999999999999822 ) ) ;
#10039=CARTESIAN_POINT ( 'NONE',  ( 47.21331623427115431, 33.48561063518610581, -10.50000000000000000 ) ) ;
#10040=CARTESIAN_POINT ( 'NONE',  ( -89.61631465359519666, -37.12029293941281338, 10.49999999999999822 ) ) ;
#10041=ORIENTED_EDGE ( 'NONE', *, *, #12434, .F. ) ;
#10042=DIRECTION ( 'NONE',  ( -1.000000000000000000, 0.000000000000000000, 0.000000000000000000 ) ) ;
#10043=CARTESIAN_POINT ( 'NONE',  ( -50.84834283437000835, -14.07862063237876704, 10.49999999999999822 ) ) ;
#10044=DIRECTION ( 'NONE',  ( 1.000000000000000000, 0.000000000000000000, 0.000000000000000000 ) ) ;
#10045=CIRCLE ( 'NONE', #110, 59.50000000000000000 ) ;
#10048=EDGE_LOOP ( 'NONE', ( #9556, #7428, #14709, #2745, #12409 ) ) ;
#10049=EDGE_CURVE ( 'NONE', #7502, #12871, #13583, .T. ) ;
#10050=DIRECTION ( 'NONE',  ( 0.000000000000000000, 0.000000000000000000, 1.000000000000000000 ) ) ;
#10051=EDGE_CURVE ( 'NONE', #9770, #8885, #12615, .T. ) ;
#10055=AXIS2_PLACEMENT_3D ( 'NONE', #9754, #13616, #2717 ) ;
#10056=DIRECTION ( 'NONE',  ( 0.000000000000000000, 0.000000000000000000, 1.000000000000000000 ) ) ;
#10057=LINE ( 'NONE', #3086, #1300 ) ;
#10058=AXIS2_PLACEMENT_3D ( 'NONE', #7854, #13794, #13554 ) ;
#10060=ORIENTED_EDGE ( 'NONE', *, *, #4262, .T. ) ;
#10061=VECTOR ( 'NONE', #12495, 1000.000000000000000 ) ;
#10062=AXIS2_PLACEMENT_3D ( 'NONE', #14618, #3297, #4215 ) ;
#10063=EDGE_CURVE ( 'NONE', #13418, #14780, #6, .T. ) ;
#10066=CARTESIAN_POINT ( 'NONE',  ( 0.000000000000000000, 0.000000000000000000, -13.00000000000000178 ) ) ;
#10067=DIRECTION ( 'NONE',  ( 0.000000000000000000, 0.000000000000000000, 1.000000000000000000 ) ) ;
#10068=EDGE_CURVE ( 'NONE', #8464, #10287, #7511, .T. ) ;
#10069=DIRECTION ( 'NONE',  ( -1.000000000000000000, 3.530314442338765862E-15, 0.000000000000000000 ) ) ;
#10071=AXIS2_PLACEMENT_3D ( 'NONE', #1444, #2424, #12912 ) ;
#10072=VERTEX_POINT ( 'NONE', #3585 ) ;
#10073=EDGE_CURVE ( 'NONE', #1517, #13137, #10919, .T. ) ;
#10074=AXIS2_PLACEMENT_3D ( 'NONE', #10468, #12901, #10611 ) ;
#10078=CARTESIAN_POINT ( 'NONE',  ( 0.5000000000000045519, -97.00000000000000000, 10.49999999999999822 ) ) ;
#10081=AXIS2_PLACEMENT_3D ( 'NONE', #528, #9695, #8711 ) ;
#10082=CARTESIAN_POINT ( 'NONE',  ( -26.49999999999971578, -45.89934640057541060, 8.000000000000000000 ) ) ;
#10083=DIRECTION ( 'NONE',  ( -0.000000000000000000, -0.000000000000000000, 1.000000000000000000 ) ) ;
#10084=ORIENTED_EDGE ( 'NONE', *, *, #8388, .T. ) ;
#10085=LINE ( 'NONE', #7657, #14302 ) ;
#10086=ORIENTED_EDGE ( 'NONE', *, *, #12062, .F. ) ;
#10087=ORIENTED_EDGE ( 'NONE', *, *, #8096, .F. ) ;
#10088=FACE_OUTER_BOUND ( 'NONE', #34, .T. ) ;
#10089=CIRCLE ( 'NONE', #11564, 3.000000000000002665 ) ;
#10090=PLANE ( 'NONE',  #18 ) ;
#10091=EDGE_CURVE ( 'NONE', #9453, #8412, #1948, .T. ) ;
#10093=EDGE_CURVE ( 'NONE', #8421, #6180, #5844, .T. ) ;
#10094=CARTESIAN_POINT ( 'NONE',  ( 2.449293598294700991E-16, -97.00000000000000000, 10.49999999999999822 ) ) ;
#10095=CARTESIAN_POINT ( 'NONE',  ( 71.53347797788771345, 69.16568774265620334, -13.00000000000000178 ) ) ;
#10096=DIRECTION ( 'NONE',  ( 0.000000000000000000, 0.000000000000000000, 1.000000000000000000 ) ) ;
#10097=ADVANCED_FACE ( 'NONE', ( #2290 ), #80, .T. ) ;
#10098=VERTEX_POINT ( 'NONE', #1745 ) ;
#10099=VECTOR ( 'NONE', #3217, 1000.000000000000000 ) ;
#10100=DIRECTION ( 'NONE',  ( 1.000000000000000000, 0.000000000000000000, 0.000000000000000000 ) ) ;
#10102=EDGE_CURVE ( 'NONE', #8421, #7767, #1224, .T. ) ;
#10103=CARTESIAN_POINT ( 'NONE',  ( -12.86891638962156215, 56.43380494353993271, 10.49999999999999822 ) ) ;
#10104=DIRECTION ( 'NONE',  ( 1.000000000000000000, 0.000000000000000000, 0.000000000000000000 ) ) ;
#10108=ORIENTED_EDGE ( 'NONE', *, *, #13306, .T. ) ;
#10113=FACE_OUTER_BOUND ( 'NONE', #2252, .T. ) ;
#10114=CARTESIAN_POINT ( 'NONE',  ( 52.54657765281197612, -6.917888187662545540, -13.00000000000000178 ) ) ;
#10116=CARTESIAN_POINT ( 'NONE',  ( 9.714003807514266953, 53.63365512954683112, 8.000000000000000000 ) ) ;
#10118=CARTESIAN_POINT ( 'NONE',  ( -68.58935777509427112, 68.58935777509594800, 8.000000000000000000 ) ) ;
#10120=DIRECTION ( 'NONE',  ( -1.000000000000000000, 0.000000000000000000, 0.000000000000000000 ) ) ;
#10121=CYLINDRICAL_SURFACE ( 'NONE', #5206, 63.00000000000000000 ) ;
#10122=ORIENTED_EDGE ( 'NONE', *, *, #7217, .F. ) ;
#10123=CARTESIAN_POINT ( 'NONE',  ( -32.26435573746199736, 42.04772703543562073, -10.50000000000000000 ) ) ;
#10124=ORIENTED_EDGE ( 'NONE', *, *, #14358, .F. ) ;
#10127=ORIENTED_EDGE ( 'NONE', *, *, #5862, .F. ) ;
#10129=LINE ( 'NONE', #2010, #11676 ) ;
#10132=ORIENTED_EDGE ( 'NONE', *, *, #10093, .T. ) ;
#10133=ORIENTED_EDGE ( 'NONE', *, *, #2111, .F. ) ;
#10134=ORIENTED_EDGE ( 'NONE', *, *, #10073, .F. ) ;
#10138=DIRECTION ( 'NONE',  ( 1.000000000000000000, 0.000000000000000000, 0.000000000000000000 ) ) ;
#10139=VERTEX_POINT ( 'NONE', #14210 ) ;
#10141=ORIENTED_EDGE ( 'NONE', *, *, #2021, .F. ) ;
#10144=DIRECTION ( 'NONE',  ( 1.000000000000000000, 0.000000000000000000, 0.000000000000000000 ) ) ;
#10147=DIRECTION ( 'NONE',  ( 0.000000000000000000, 0.000000000000000000, 1.000000000000000000 ) ) ;
#10148=CARTESIAN_POINT ( 'NONE',  ( -41.94820822869193222, -33.29654390035832279, -10.50000000000000000 ) ) ;
#10149=ORIENTED_EDGE ( 'NONE', *, *, #4079, .F. ) ;
#10150=EDGE_CURVE ( 'NONE', #5988, #9656, #6291, .T. ) ;
#10152=CARTESIAN_POINT ( 'NONE',  ( -2.449293598294700991E-16, 97.00000000000000000, -10.50000000000000000 ) ) ;
#10153=VERTEX_POINT ( 'NONE', #9775 ) ;
#10154=ORIENTED_EDGE ( 'NONE', *, *, #13980, .T. ) ;
#10155=FACE_OUTER_BOUND ( 'NONE', #13085, .T. ) ;
#10156=CARTESIAN_POINT ( 'NONE',  ( -52.54657765281192638, 6.917888187662934563, -10.50000000000000000 ) ) ;
#10157=AXIS2_PLACEMENT_3D ( 'NONE', #9486, #3885, #9632 ) ;
#10158=CARTESIAN_POINT ( 'NONE',  ( -26.49999999999971578, -45.89934640057541060, -10.50000000000000000 ) ) ;
#10161=DIRECTION ( 'NONE',  ( -0.000000000000000000, -0.000000000000000000, 1.000000000000000000 ) ) ;
#10162=DIRECTION ( 'NONE',  ( -1.000000000000000000, 0.000000000000000000, 0.000000000000000000 ) ) ;
#10166=ORIENTED_EDGE ( 'NONE', *, *, #8469, .T. ) ;
#10167=DIRECTION ( 'NONE',  ( 0.000000000000000000, 0.000000000000000000, 1.000000000000000000 ) ) ;
#10168=AXIS2_PLACEMENT_3D ( 'NONE', #3497, #11624, #10471 ) ;
#10169=CARTESIAN_POINT ( 'NONE',  ( -96.58511096861892042, -0.2790467552922097916, 10.49999999999999822 ) ) ;
#10170=ADVANCED_FACE ( 'NONE', ( #13220 ), #14427, .T. ) ;
#10171=ORIENTED_EDGE ( 'NONE', *, *, #733, .T. ) ;
#10172=CARTESIAN_POINT ( 'NONE',  ( 9.706953719245472456, 57.06275842387054098, -13.00000000000000178 ) ) ;
#10175=ADVANCED_FACE ( 'NONE', ( #5162 ), #7354, .T. ) ;
#10176=DIRECTION ( 'NONE',  ( 1.000000000000000000, 0.000000000000000000, 0.000000000000000000 ) ) ;
#10179=VECTOR ( 'NONE', #6627, 1000.000000000000000 ) ;
#10180=DIRECTION ( 'NONE',  ( 0.000000000000000000, 0.000000000000000000, 1.000000000000000000 ) ) ;
#10181=DIRECTION ( 'NONE',  ( 0.000000000000000000, 0.000000000000000000, 1.000000000000000000 ) ) ;
#10182=EDGE_CURVE ( 'NONE', #9719, #13003, #3735, .T. ) ;
#10183=AXIS2_PLACEMENT_3D ( 'NONE', #2377, #3533, #178 ) ;
#10184=CYLINDRICAL_SURFACE ( 'NONE', #5070, 3.000000000000002665 ) ;
#10188=CARTESIAN_POINT ( 'NONE',  ( -53.63365512954686665, 9.714003807514082212, -13.00000000000000178 ) ) ;
#10189=CYLINDRICAL_SURFACE ( 'NONE', #6145, 0.5000000000000004441 ) ;
#10190=EDGE_CURVE ( 'NONE', #9586, #11551, #8251, .T. ) ;
#10192=EDGE_CURVE ( 'NONE', #12171, #8537, #13339, .T. ) ;
#10193=CARTESIAN_POINT ( 'NONE',  ( 41.59008834022645829, 32.46576781417968505, -10.50000000000000000 ) ) ;
#10194=CIRCLE ( 'NONE', #7515, 3.000000000000002665 ) ;
#10195=CARTESIAN_POINT ( 'NONE',  ( 0.000000000000000000, 0.000000000000000000, -8.000000000000000000 ) ) ;
#10196=VECTOR ( 'NONE', #1433, 1000.000000000000000 ) ;
#10201=DIRECTION ( 'NONE',  ( -1.000000000000000000, 0.000000000000000000, 0.000000000000000000 ) ) ;
#10205=AXIS2_PLACEMENT_3D ( 'NONE', #8874, #13508, #11240 ) ;
#10206=CARTESIAN_POINT ( 'NONE',  ( -52.54657765281192638, 6.917888187662934563, -13.00000000000000178 ) ) ;
#10207=DIRECTION ( 'NONE',  ( 0.000000000000000000, 0.000000000000000000, -1.000000000000000000 ) ) ;
#10209=ORIENTED_EDGE ( 'NONE', *, *, #1930, .T. ) ;
#10210=CIRCLE ( 'NONE', #11926, 0.5000000000000004441 ) ;
#10211=ORIENTED_EDGE ( 'NONE', *, *, #3291, .T. ) ;
#10214=DIRECTION ( 'NONE',  ( 0.000000000000000000, 0.000000000000000000, -1.000000000000000000 ) ) ;
#10217=ORIENTED_EDGE ( 'NONE', *, *, #1066, .T. ) ;
#10218=AXIS2_PLACEMENT_3D ( 'NONE', #7454, #1351, #14456 ) ;
#10221=AXIS2_PLACEMENT_3D ( 'NONE', #5646, #14922, #12562 ) ;
#10223=CARTESIAN_POINT ( 'NONE',  ( 0.000000000000000000, 0.000000000000000000, -13.00000000000000178 ) ) ;
#10226=FACE_OUTER_BOUND ( 'NONE', #13181, .T. ) ;
#10228=DIRECTION ( 'NONE',  ( -0.000000000000000000, -0.000000000000000000, 1.000000000000000000 ) ) ;
#10231=CARTESIAN_POINT ( 'NONE',  ( -26.49999999999971578, -45.89934640057541060, -8.000000000000000000 ) ) ;
#10232=ORIENTED_EDGE ( 'NONE', *, *, #7202, .F. ) ;
#10234=ORIENTED_EDGE ( 'NONE', *, *, #10451, .T. ) ;
#10235=ORIENTED_EDGE ( 'NONE', *, *, #7437, .F. ) ;
#10236=DIRECTION ( 'NONE',  ( -1.000000000000000000, 0.000000000000000000, 0.000000000000000000 ) ) ;
#10238=CIRCLE ( 'NONE', #9504, 0.5000000000000004441 ) ;
#10239=EDGE_CURVE ( 'NONE', #12645, #7413, #7577, .T. ) ;
#10240=ORIENTED_EDGE ( 'NONE', *, *, #8851, .T. ) ;
#10241=ADVANCED_FACE ( 'NONE', ( #3042 ), #14499, .F. ) ;
#10242=EDGE_CURVE ( 'NONE', #12545, #13279, #4136, .T. ) ;
#10243=FACE_OUTER_BOUND ( 'NONE', #8199, .T. ) ;
#10244=CARTESIAN_POINT ( 'NONE',  ( 9.706953719245472456, 57.06275842387054098, -13.00000000000000178 ) ) ;
#10245=ORIENTED_EDGE ( 'NONE', *, *, #3993, .T. ) ;
#10246=VECTOR ( 'NONE', #2901, 1000.000000000000000 ) ;
#10249=CARTESIAN_POINT ( 'NONE',  ( 71.58935777509475429, -68.58935777509547904, -13.00000000000000178 ) ) ;
#10253=CARTESIAN_POINT ( 'NONE',  ( -97.41488903138106537, 0.2790467552942557661, -10.50000000000000000 ) ) ;
#10255=CIRCLE ( 'NONE', #2263, 53.55662432702593634 ) ;
#10256=ORIENTED_EDGE ( 'NONE', *, *, #14604, .F. ) ;
#10258=CARTESIAN_POINT ( 'NONE',  ( -97.00000000000000000, 1.015776140243522349E-12, 10.49999999999999822 ) ) ;
#10260=CARTESIAN_POINT ( 'NONE',  ( -51.19406879332065330, -13.71740939043347041, -13.00000000000000178 ) ) ;
#10261=EDGE_CURVE ( 'NONE', #10098, #5511, #1462, .T. ) ;
#10262=DIRECTION ( 'NONE',  ( 1.000000000000000000, 0.000000000000000000, 0.000000000000000000 ) ) ;
#10269=DIRECTION ( 'NONE',  ( 1.000000000000000000, 0.000000000000000000, 0.000000000000000000 ) ) ;
#10270=CONICAL_SURFACE ( 'NONE', #7098, 55.00000000000000000, 0.5235987755983000369 ) ;
#10271=ORIENTED_EDGE ( 'NONE', *, *, #9138, .T. ) ;
#10272=DIRECTION ( 'NONE',  ( 1.000000000000000000, 0.000000000000000000, 0.000000000000000000 ) ) ;
#10273=DIRECTION ( 'NONE',  ( 0.000000000000000000, 0.000000000000000000, 1.000000000000000000 ) ) ;
#10276=CARTESIAN_POINT ( 'NONE',  ( 26.49999999999971578, 45.89934640057541060, -8.000000000000000000 ) ) ;
#10277=ORIENTED_EDGE ( 'NONE', *, *, #5225, .F. ) ;
#10278=DIRECTION ( 'NONE',  ( -0.000000000000000000, -0.000000000000000000, 1.000000000000000000 ) ) ;
#10279=AXIS2_PLACEMENT_3D ( 'NONE', #6461, #7755, #11265 ) ;
#10280=EDGE_LOOP ( 'NONE', ( #860, #3397, #5194, #3581 ) ) ;
#10282=DIRECTION ( 'NONE',  ( -1.000000000000000000, 0.000000000000000000, 0.000000000000000000 ) ) ;
#10283=EDGE_CURVE ( 'NONE', #6334, #1631, #10679, .T. ) ;
#10286=CARTESIAN_POINT ( 'NONE',  ( -42.50536573064432133, -32.06294366074479996, 10.49999999999999822 ) ) ;
#10287=VERTEX_POINT ( 'NONE', #917 ) ;
#10288=ADVANCED_FACE ( 'NONE', ( #3113 ), #1967, .F. ) ;
#10289=ORIENTED_EDGE ( 'NONE', *, *, #3098, .F. ) ;
#10290=VECTOR ( 'NONE', #3851, 1000.000000000000000 ) ;
#10291=CYLINDRICAL_SURFACE ( 'NONE', #7418, 0.5000000000000004441 ) ;
#10294=VERTEX_POINT ( 'NONE', #1892 ) ;
#10295=ADVANCED_FACE ( 'NONE', ( #843 ), #8714, .T. ) ;
#10296=ORIENTED_EDGE ( 'NONE', *, *, #10013, .F. ) ;
#10297=CIRCLE ( 'NONE', #11533, 3.000000000000002665 ) ;
#10301=AXIS2_PLACEMENT_3D ( 'NONE', #228, #84, #8278 ) ;
#10302=DIRECTION ( 'NONE',  ( -1.000000000000000000, 0.000000000000000000, 0.000000000000000000 ) ) ;
#10303=ADVANCED_FACE ( 'NONE', ( #13359 ), #10090, .F. ) ;
#10304=CARTESIAN_POINT ( 'NONE',  ( -22.33583958711380646, -30.74264578624812927, -28.00000000000000000 ) ) ;
#10305=DIRECTION ( 'NONE',  ( 0.000000000000000000, 0.000000000000000000, -1.000000000000000000 ) ) ;
#10306=ORIENTED_EDGE ( 'NONE', *, *, #2398, .T. ) ;
#10307=DIRECTION ( 'NONE',  ( 1.000000000000000000, 0.000000000000000000, 0.000000000000000000 ) ) ;
#10308=ORIENTED_EDGE ( 'NONE', *, *, #11567, .F. ) ;
#10309=EDGE_LOOP ( 'NONE', ( #7104, #5284, #4095, #519 ) ) ;
#10312=AXIS2_PLACEMENT_3D ( 'NONE', #13912, #3507, #8126 ) ;
#10313=ORIENTED_EDGE ( 'NONE', *, *, #9060, .F. ) ;
#10314=AXIS2_PLACEMENT_3D ( 'NONE', #11698, #3494, #8186 ) ;
#10316=DIRECTION ( 'NONE',  ( -1.000000000000000000, 0.000000000000000000, 0.000000000000000000 ) ) ;
#10317=EDGE_LOOP ( 'NONE', ( #9010, #6395, #8933, #11522 ) ) ;
#10318=ORIENTED_EDGE ( 'NONE', *, *, #3161, .F. ) ;
#10321=DIRECTION ( 'NONE',  ( 0.000000000000000000, 0.000000000000000000, -1.000000000000000000 ) ) ;
#10324=CARTESIAN_POINT ( 'NONE',  ( 89.61631465359468507, -37.12029293941410657, -13.00000000000000178 ) ) ;
#10325=CYLINDRICAL_SURFACE ( 'NONE', #12608, 0.5000000000000022204 ) ;
#10326=ORIENTED_EDGE ( 'NONE', *, *, #5517, .F. ) ;
#10327=CARTESIAN_POINT ( 'NONE',  ( -100.0000000000000000, 0.000000000000000000, 13.00000000000000178 ) ) ;
#10328=EDGE_CURVE ( 'NONE', #12813, #14403, #2046, .T. ) ;
#10329=CIRCLE ( 'NONE', #14216, 20.00000000000000000 ) ;
#10330=CARTESIAN_POINT ( 'NONE',  ( -6.917888187662729393, -52.54657765281195481, -8.000000000000000000 ) ) ;
#10332=EDGE_CURVE ( 'NONE', #13279, #3803, #5354, .T. ) ;
#10334=CARTESIAN_POINT ( 'NONE',  ( 56.43380494353997534, 12.86891638962136319, -13.00000000000000178 ) ) ;
#10335=ORIENTED_EDGE ( 'NONE', *, *, #275, .F. ) ;
#10338=CARTESIAN_POINT ( 'NONE',  ( 47.21331623427115431, 33.48561063518610581, -8.000000000000000000 ) ) ;
#10344=DIRECTION ( 'NONE',  ( -1.000000000000000000, -1.765157221169382931E-15, 0.000000000000000000 ) ) ;
#10345=ORIENTED_EDGE ( 'NONE', *, *, #10472, .T. ) ;
#10346=EDGE_CURVE ( 'NONE', #13523, #6738, #4411, .T. ) ;
#10347=EDGE_CURVE ( 'NONE', #9024, #11429, #3669, .T. ) ;
#10348=CARTESIAN_POINT ( 'NONE',  ( 70.20695371924547601, 57.06275842387054098, -13.00000000000000178 ) ) ;
#10351=AXIS2_PLACEMENT_3D ( 'NONE', #542, #773, #5171 ) ;
#10352=DIRECTION ( 'NONE',  ( -0.000000000000000000, -0.000000000000000000, 1.000000000000000000 ) ) ;
#10353=ORIENTED_EDGE ( 'NONE', *, *, #12062, .T. ) ;
#10354=CYLINDRICAL_SURFACE ( 'NONE', #10697, 56.99999999999999289 ) ;
#10355=VERTEX_POINT ( 'NONE', #4628 ) ;
#10356=FACE_OUTER_BOUND ( 'NONE', #2558, .T. ) ;
#10357=CARTESIAN_POINT ( 'NONE',  ( -45.89934640057513349, 26.50000000000019540, -10.50000000000000000 ) ) ;
#10358=DIRECTION ( 'NONE',  ( -0.000000000000000000, -0.000000000000000000, -1.000000000000000000 ) ) ;
#10359=DIRECTION ( 'NONE',  ( -1.000000000000000000, -1.776356839400250465E-15, 0.000000000000000000 ) ) ;
#10360=ORIENTED_EDGE ( 'NONE', *, *, #6039, .F. ) ;
#10362=VERTEX_POINT ( 'NONE', #14037 ) ;
#10363=FACE_OUTER_BOUND ( 'NONE', #12554, .T. ) ;
#10364=CARTESIAN_POINT ( 'NONE',  ( 68.58935777509475429, -68.58935777509547904, -13.00000000000000178 ) ) ;
#10365=DIRECTION ( 'NONE',  ( 0.000000000000000000, 0.000000000000000000, 1.000000000000000000 ) ) ;
#10366=ORIENTED_EDGE ( 'NONE', *, *, #9036, .T. ) ;
#10369=EDGE_CURVE ( 'NONE', #7243, #10452, #13748, .T. ) ;
#10370=ORIENTED_EDGE ( 'NONE', *, *, #13933, .F. ) ;
#10373=CARTESIAN_POINT ( 'NONE',  ( 0.000000000000000000, 0.000000000000000000, -28.00000000000000000 ) ) ;
#10374=DIRECTION ( 'NONE',  ( 1.000000000000000000, 0.000000000000000000, 0.000000000000000000 ) ) ;
#10377=DIRECTION ( 'NONE',  ( 0.000000000000000000, 0.000000000000000000, 1.000000000000000000 ) ) ;
#10378=EDGE_CURVE ( 'NONE', #14446, #4759, #7038, .T. ) ;
#10379=ORIENTED_EDGE ( 'NONE', *, *, #14648, .F. ) ;
#10383=CARTESIAN_POINT ( 'NONE',  ( -29.26435573746199381, 42.04772703543562073, -13.00000000000000178 ) ) ;
#10386=EDGE_CURVE ( 'NONE', #1155, #8687, #7954, .T. ) ;
#10387=ADVANCED_FACE ( 'NONE', ( #10243 ), #5607, .F. ) ;
#10388=ORIENTED_EDGE ( 'NONE', *, *, #5009, .F. ) ;
#10390=ORIENTED_EDGE ( 'NONE', *, *, #2040, .T. ) ;
#10391=VERTEX_POINT ( 'NONE', #12821 ) ;
#10392=DIRECTION ( 'NONE',  ( -1.000000000000000000, 0.000000000000000000, 0.000000000000000000 ) ) ;
#10393=DIRECTION ( 'NONE',  ( -1.000000000000000000, 0.000000000000000000, 0.000000000000000000 ) ) ;
#10395=DIRECTION ( 'NONE',  ( 1.000000000000000000, 0.000000000000000000, -0.000000000000000000 ) ) ;
#10396=VERTEX_POINT ( 'NONE', #1145 ) ;
#10398=ORIENTED_EDGE ( 'NONE', *, *, #7477, .F. ) ;
#10399=DIRECTION ( 'NONE',  ( 0.000000000000000000, 0.000000000000000000, 1.000000000000000000 ) ) ;
#10400=CARTESIAN_POINT ( 'NONE',  ( -89.12622059913283579, -37.21932736666236963, -13.00000000000000178 ) ) ;
#10402=FACE_OUTER_BOUND ( 'NONE', #11531, .T. ) ;
#10404=DIRECTION ( 'NONE',  ( 0.000000000000000000, 0.000000000000000000, 1.000000000000000000 ) ) ;
#10406=CARTESIAN_POINT ( 'NONE',  ( -33.48561063518626923, 47.21331623427104063, 8.000000000000000000 ) ) ;
#10410=CARTESIAN_POINT ( 'NONE',  ( -49.00442420935969778, 30.80502811811250297, 10.49999999999999822 ) ) ;
#10412=CARTESIAN_POINT ( 'NONE',  ( -57.06275842387042729, 9.706953719246069312, -8.000000000000000000 ) ) ;
#10413=ORIENTED_EDGE ( 'NONE', *, *, #8764, .T. ) ;
#10415=CARTESIAN_POINT ( 'NONE',  ( 45.91029614918936375, -26.00011991137331790, -13.00000000000000178 ) ) ;
#10416=DIRECTION ( 'NONE',  ( 0.000000000000000000, 0.000000000000000000, 1.000000000000000000 ) ) ;
#10417=AXIS2_PLACEMENT_3D ( 'NONE', #8486, #13135, #3804 ) ;
#10418=DIRECTION ( 'NONE',  ( 0.000000000000000000, 0.000000000000000000, 1.000000000000000000 ) ) ;
#10420=CIRCLE ( 'NONE', #5330, 53.55662432702593634 ) ;
#10421=DIRECTION ( 'NONE',  ( 1.000000000000000000, 0.000000000000000000, 0.000000000000000000 ) ) ;
#10422=AXIS2_PLACEMENT_3D ( 'NONE', #7151, #5865, #1032 ) ;
#10423=ORIENTED_EDGE ( 'NONE', *, *, #1088, .F. ) ;
#10424=EDGE_CURVE ( 'NONE', #5889, #10698, #7525, .T. ) ;
#10425=AXIS2_PLACEMENT_3D ( 'NONE', #14132, #13000, #1528 ) ;
#10427=EDGE_CURVE ( 'NONE', #11737, #7919, #12153, .T. ) ;
#10428=CARTESIAN_POINT ( 'NONE',  ( 0.000000000000000000, 0.000000000000000000, -13.00000000000000178 ) ) ;
#10429=EDGE_CURVE ( 'NONE', #10153, #1144, #14324, .T. ) ;
#10431=CARTESIAN_POINT ( 'NONE',  ( 0.000000000000000000, 0.000000000000000000, -10.50000000000000000 ) ) ;
#10432=AXIS2_PLACEMENT_3D ( 'NONE', #11491, #1223, #12693 ) ;
#10433=ORIENTED_EDGE ( 'NONE', *, *, #7731, .T. ) ;
#10435=AXIS2_PLACEMENT_3D ( 'NONE', #8203, #5770, #163 ) ;
#10437=CARTESIAN_POINT ( 'NONE',  ( -41.59008834022669987, -32.46576781417940794, -10.50000000000000000 ) ) ;
#10438=EDGE_LOOP ( 'NONE', ( #1835, #1245, #13913, #8165, #12497, #4132, #11726, #1149, #3821, #14184, #12096, #7999 ) ) ;
#10439=ORIENTED_EDGE ( 'NONE', *, *, #14836, .T. ) ;
#10442=CIRCLE ( 'NONE', #12389, 0.5000000000000004441 ) ;
#10443=FACE_OUTER_BOUND ( 'NONE', #488, .T. ) ;
#10444=CIRCLE ( 'NONE', #12877, 52.50000000000000711 ) ;
#10445=DIRECTION ( 'NONE',  ( 1.000000000000000000, 0.000000000000000000, 0.000000000000000000 ) ) ;
#10446=CIRCLE ( 'NONE', #13123, 56.99999999999999289 ) ;
#10447=CARTESIAN_POINT ( 'NONE',  ( 50.00000000000000000, 6.123233995736766085E-15, 13.00000000000000178 ) ) ;
#10449=CARTESIAN_POINT ( 'NONE',  ( 30.80502811811196295, 49.00442420936003174, -10.50000000000000000 ) ) ;
#10450=DIRECTION ( 'NONE',  ( 0.000000000000000000, 0.000000000000000000, 1.000000000000000000 ) ) ;
#10451=EDGE_CURVE ( 'NONE', #5144, #14021, #4635, .T. ) ;
#10452=VERTEX_POINT ( 'NONE', #14962 ) ;
#10453=ORIENTED_EDGE ( 'NONE', *, *, #9911, .F. ) ;
#10456=CARTESIAN_POINT ( 'NONE',  ( -42.89934640057513349, 26.50000000000019540, 8.000000000000000000 ) ) ;
#10457=VECTOR ( 'NONE', #12140, 1000.000000000000000 ) ;
#10458=ORIENTED_EDGE ( 'NONE', *, *, #9144, .F. ) ;
#10459=AXIS2_PLACEMENT_3D ( 'NONE', #10646, #13862, #8155 ) ;
#10461=ORIENTED_EDGE ( 'NONE', *, *, #9437, .F. ) ;
#10462=DIRECTION ( 'NONE',  ( -1.000000000000000000, 0.000000000000000000, 0.000000000000000000 ) ) ;
#10463=ORIENTED_EDGE ( 'NONE', *, *, #8552, .F. ) ;
#10464=ORIENTED_EDGE ( 'NONE', *, *, #11085, .F. ) ;
#10467=CIRCLE ( 'NONE', #6822, 56.99999999999999289 ) ;
#10468=CARTESIAN_POINT ( 'NONE',  ( -49.00442420935969778, 30.80502811811250297, -13.00000000000000178 ) ) ;
#10470=ADVANCED_FACE ( 'NONE', ( #9172 ), #6811, .F. ) ;
#10471=DIRECTION ( 'NONE',  ( -1.000000000000000000, 0.000000000000000000, 0.000000000000000000 ) ) ;
#10472=EDGE_CURVE ( 'NONE', #2085, #13671, #10442, .T. ) ;
#10475=CYLINDRICAL_SURFACE ( 'NONE', #1004, 0.5000000000000022204 ) ;
#10476=CARTESIAN_POINT ( 'NONE',  ( 47.63108361037843252, 56.43380494353993271, 10.49999999999999822 ) ) ;
#10477=EDGE_LOOP ( 'NONE', ( #1274, #1600, #14204, #3269, #3239, #6943 ) ) ;
#10478=FACE_OUTER_BOUND ( 'NONE', #6366, .T. ) ;
#10479=EDGE_CURVE ( 'NONE', #345, #12576, #6804, .T. ) ;
#10480=DIRECTION ( 'NONE',  ( 0.000000000000000000, 0.000000000000000000, 1.000000000000000000 ) ) ;
#10481=AXIS2_PLACEMENT_3D ( 'NONE', #10357, #1249, #11433 ) ;
#10482=ORIENTED_EDGE ( 'NONE', *, *, #6099, .F. ) ;
#10483=CARTESIAN_POINT ( 'NONE',  ( 33.49014761921571193, 11.74264578624841171, -28.00000000000000000 ) ) ;
#10484=CARTESIAN_POINT ( 'NONE',  ( 24.99999999999971934, 43.30127018922209459, 8.000000000000000000 ) ) ;
#10485=CARTESIAN_POINT ( 'NONE',  ( 44.13108361037843252, 56.43380494353993271, 8.000000000000000000 ) ) ;
#10486=DIRECTION ( 'NONE',  ( 1.000000000000000000, 0.000000000000000000, 0.000000000000000000 ) ) ;
#10489=AXIS2_PLACEMENT_3D ( 'NONE', #10589, #5122, #9734 ) ;
#10492=ORIENTED_EDGE ( 'NONE', *, *, #133, .T. ) ;
#10494=CARTESIAN_POINT ( 'NONE',  ( -68.49330278050074128, 68.09867107463051639, -10.50000000000000000 ) ) ;
#10496=DIRECTION ( 'NONE',  ( 0.000000000000000000, 0.000000000000000000, 1.000000000000000000 ) ) ;
#10498=AXIS2_PLACEMENT_3D ( 'NONE', #8146, #2147, #12629 ) ;
#10499=ORIENTED_EDGE ( 'NONE', *, *, #1891, .T. ) ;
#10500=CARTESIAN_POINT ( 'NONE',  ( 24.98583958711423492, -30.74264578624780597, -28.00000000000000000 ) ) ;
#10501=ORIENTED_EDGE ( 'NONE', *, *, #5877, .T. ) ;
#10502=CIRCLE ( 'NONE', #12451, 57.00000000000000000 ) ;
#10503=CARTESIAN_POINT ( 'NONE',  ( 50.00000000000000000, 6.123233995736766085E-15, 8.000000000000000000 ) ) ;
#10505=AXIS2_PLACEMENT_3D ( 'NONE', #336, #10874, #14232 ) ;
#10507=CARTESIAN_POINT ( 'NONE',  ( -6.917888187662729393, -52.54657765281195481, -10.50000000000000000 ) ) ;
#10512=CARTESIAN_POINT ( 'NONE',  ( 89.61631465359468507, -37.12029293941410657, -8.000000000000000000 ) ) ;
#10513=ADVANCED_FACE ( 'NONE', ( #1364 ), #14189, .F. ) ;
#10514=ORIENTED_EDGE ( 'NONE', *, *, #10346, .F. ) ;
#10515=EDGE_CURVE ( 'NONE', #5248, #12429, #4843, .T. ) ;
#10516=AXIS2_PLACEMENT_3D ( 'NONE', #5946, #10810, #5040 ) ;
#10517=ORIENTED_EDGE ( 'NONE', *, *, #11827, .F. ) ;
#10518=ORIENTED_EDGE ( 'NONE', *, *, #8969, .F. ) ;
#10519=DIRECTION ( 'NONE',  ( -1.000000000000000000, 0.000000000000000000, 0.000000000000000000 ) ) ;
#10521=CARTESIAN_POINT ( 'NONE',  ( 52.54657765281197612, -6.917888187662545540, -10.50000000000000000 ) ) ;
#10522=VECTOR ( 'NONE', #13930, 1000.000000000000000 ) ;
#10523=CARTESIAN_POINT ( 'NONE',  ( -13.35619814848797837, 51.53979475227131246, -13.00000000000000178 ) ) ;
#10524=AXIS2_PLACEMENT_3D ( 'NONE', #12468, #1984, #11027 ) ;
#10525=CIRCLE ( 'NONE', #3991, 59.50000000000000000 ) ;
#10526=AXIS2_PLACEMENT_3D ( 'NONE', #477, #14011, #12860 ) ;
#10528=EDGE_LOOP ( 'NONE', ( #9853, #12979, #8765, #7935, #8229 ) ) ;
#10532=ADVANCED_FACE ( 'NONE', ( #5066 ), #3938, .F. ) ;
#10533=ORIENTED_EDGE ( 'NONE', *, *, #4347, .F. ) ;
#10535=EDGE_LOOP ( 'NONE', ( #8104, #1927, #14442, #864 ) ) ;
#10536=CARTESIAN_POINT ( 'NONE',  ( -49.54657765281192638, 6.917888187662934563, -8.000000000000000000 ) ) ;
#10537=AXIS2_PLACEMENT_3D ( 'NONE', #7201, #2425, #387 ) ;
#10538=CIRCLE ( 'NONE', #13446, 3.000000000000002665 ) ;
#10539=ORIENTED_EDGE ( 'NONE', *, *, #7123, .T. ) ;
#10542=FACE_OUTER_BOUND ( 'NONE', #6315, .T. ) ;
#10543=CARTESIAN_POINT ( 'NONE',  ( 100.0000000000000000, 1.224646799147353217E-14, 13.00000000000000178 ) ) ;
#10548=AXIS2_PLACEMENT_3D ( 'NONE', #12485, #946, #12333 ) ;
#10549=DIRECTION ( 'NONE',  ( -0.000000000000000000, -0.000000000000000000, -1.000000000000000000 ) ) ;
#10550=VECTOR ( 'NONE', #1672, 1000.000000000000000 ) ;
#10551=ORIENTED_EDGE ( 'NONE', *, *, #14241, .F. ) ;
#10552=CARTESIAN_POINT ( 'NONE',  ( 97.00000000000000000, -3.384287605079545030E-13, -10.50000000000000000 ) ) ;
#10554=EDGE_CURVE ( 'NONE', #3770, #4485, #3419, .T. ) ;
#10555=CIRCLE ( 'NONE', #12509, 3.000000000000002665 ) ;
#10557=ADVANCED_FACE ( 'NONE', ( #7254 ), #7419, .T. ) ;
#10559=CARTESIAN_POINT ( 'NONE',  ( -57.06275842387042729, 9.706953719246069312, 8.000000000000000000 ) ) ;
#10560=AXIS2_PLACEMENT_3D ( 'NONE', #1603, #13144, #13222 ) ;
#10561=EDGE_CURVE ( 'NONE', #11882, #5656, #13851, .T. ) ;
#10562=CARTESIAN_POINT ( 'NONE',  ( -34.62083247296263266, -87.95718916809180143, -8.000000000000000000 ) ) ;
#10563=CARTESIAN_POINT ( 'NONE',  ( 12.86891638962116247, -56.43380494354001087, -13.00000000000000178 ) ) ;
#10564=CARTESIAN_POINT ( 'NONE',  ( 0.000000000000000000, 0.000000000000000000, 10.50000000000000000 ) ) ;
#10565=CYLINDRICAL_SURFACE ( 'NONE', #14536, 59.50000000000000000 ) ;
#10566=AXIS2_PLACEMENT_3D ( 'NONE', #10066, #14479, #4155 ) ;
#10567=EDGE_CURVE ( 'NONE', #14620, #7243, #5115, .T. ) ;
#10569=AXIS2_PLACEMENT_3D ( 'NONE', #367, #7027, #4927 ) ;
#10573=DIRECTION ( 'NONE',  ( 0.000000000000000000, 0.000000000000000000, 1.000000000000000000 ) ) ;
#10575=EDGE_CURVE ( 'NONE', #7243, #2878, #2442, .T. ) ;
#10576=VERTEX_POINT ( 'NONE', #8335 ) ;
#10577=AXIS2_PLACEMENT_3D ( 'NONE', #2910, #1999, #563 ) ;
#10578=FACE_OUTER_BOUND ( 'NONE', #13423, .T. ) ;
#10579=ORIENTED_EDGE ( 'NONE', *, *, #3665, .F. ) ;
#10580=DIRECTION ( 'NONE',  ( 1.000000000000000000, 0.000000000000000000, 0.000000000000000000 ) ) ;
#10581=DIRECTION ( 'NONE',  ( -0.000000000000000000, -0.000000000000000000, 1.000000000000000000 ) ) ;
#10582=CARTESIAN_POINT ( 'NONE',  ( 49.00442420935993226, -30.80502811811213704, 10.49999999999999822 ) ) ;
#10583=CARTESIAN_POINT ( 'NONE',  ( 0.000000000000000000, 0.000000000000000000, -10.50000000000000000 ) ) ;
#10584=ORIENTED_EDGE ( 'NONE', *, *, #2597, .T. ) ;
#10585=CIRCLE ( 'NONE', #13754, 3.000000000000002665 ) ;
#10587=CARTESIAN_POINT ( 'NONE',  ( 0.000000000000000000, 0.000000000000000000, 10.50000000000000000 ) ) ;
#10588=CYLINDRICAL_SURFACE ( 'NONE', #8094, 3.000000000000002665 ) ;
#10589=CARTESIAN_POINT ( 'NONE',  ( -6.917888187662729393, -52.54657765281195481, -13.00000000000000178 ) ) ;
#10590=VERTEX_POINT ( 'NONE', #13049 ) ;
#10592=ORIENTED_EDGE ( 'NONE', *, *, #13309, .F. ) ;
#10594=CARTESIAN_POINT ( 'NONE',  ( 0.000000000000000000, 0.000000000000000000, -8.000000000000000000 ) ) ;
#10597=DIRECTION ( 'NONE',  ( 0.000000000000000000, 0.000000000000000000, 1.000000000000000000 ) ) ;
#10599=ORIENTED_EDGE ( 'NONE', *, *, #13458, .F. ) ;
#10600=ORIENTED_EDGE ( 'NONE', *, *, #2278, .F. ) ;
#10601=FACE_OUTER_BOUND ( 'NONE', #358, .T. ) ;
#10602=CARTESIAN_POINT ( 'NONE',  ( 37.12029293941379393, 89.61631465359479876, 8.000000000000000000 ) ) ;
#10605=VERTEX_POINT ( 'NONE', #12975 ) ;
#10606=DIRECTION ( 'NONE',  ( 1.000000000000000000, 0.000000000000000000, 0.000000000000000000 ) ) ;
#10607=ORIENTED_EDGE ( 'NONE', *, *, #9727, .F. ) ;
#10608=DIRECTION ( 'NONE',  ( 0.000000000000000000, 0.000000000000000000, 1.000000000000000000 ) ) ;
#10611=DIRECTION ( 'NONE',  ( 1.000000000000000000, 0.000000000000000000, 0.000000000000000000 ) ) ;
#10612=CARTESIAN_POINT ( 'NONE',  ( 0.000000000000000000, 0.000000000000000000, -8.000000000000000000 ) ) ;
#10613=EDGE_CURVE ( 'NONE', #13122, #914, #11016, .T. ) ;
#10615=VERTEX_POINT ( 'NONE', #12066 ) ;
#10617=CIRCLE ( 'NONE', #11113, 56.99999999999999289 ) ;
#10618=CARTESIAN_POINT ( 'NONE',  ( -6.117650515114348764, -53.20607447915235610, -10.50000000000000000 ) ) ;
#10619=ORIENTED_EDGE ( 'NONE', *, *, #4545, .F. ) ;
#10621=EDGE_LOOP ( 'NONE', ( #3486, #4233, #8661, #10999, #13928 ) ) ;
#10624=DIRECTION ( 'NONE',  ( -1.000000000000000000, 0.000000000000000000, 0.000000000000000000 ) ) ;
#10625=DIRECTION ( 'NONE',  ( 0.000000000000000000, 0.000000000000000000, 1.000000000000000000 ) ) ;
#10627=DIRECTION ( 'NONE',  ( -1.000000000000000000, 0.000000000000000000, 0.000000000000000000 ) ) ;
#10628=DIRECTION ( 'NONE',  ( -0.000000000000000000, -0.000000000000000000, -1.000000000000000000 ) ) ;
#10629=CARTESIAN_POINT ( 'NONE',  ( -51.49712671369403694, -14.70911110638321873, -10.50000000000000000 ) ) ;
#10630=CYLINDRICAL_SURFACE ( 'NONE', #222, 3.000000000000002665 ) ;
#10631=ORIENTED_EDGE ( 'NONE', *, *, #12416, .T. ) ;
#10634=ADVANCED_FACE ( 'NONE', ( #6260 ), #516, .F. ) ;
#10635=CARTESIAN_POINT ( 'NONE',  ( -3.492805317593278058, 46.55633131742322917, -10.50000000000000000 ) ) ;
#10636=CARTESIAN_POINT ( 'NONE',  ( -47.21331623427138879, -33.48561063518577896, -10.50000000000000000 ) ) ;
#10638=CARTESIAN_POINT ( 'NONE',  ( 37.12029293941379393, 89.61631465359479876, -10.50000000000000000 ) ) ;
#10639=DIRECTION ( 'NONE',  ( -0.000000000000000000, -0.000000000000000000, 1.000000000000000000 ) ) ;
#10640=EDGE_LOOP ( 'NONE', ( #13831, #11462, #894, #8573, #11003 ) ) ;
#10641=CYLINDRICAL_SURFACE ( 'NONE', #7545, 60.50000000000000000 ) ;
#10644=DIRECTION ( 'NONE',  ( 1.000000000000000000, 0.000000000000000000, -0.000000000000000000 ) ) ;
#10645=AXIS2_PLACEMENT_3D ( 'NONE', #10018, #5310, #3050 ) ;
#10646=CARTESIAN_POINT ( 'NONE',  ( 89.61631465359468507, -37.12029293941410657, -13.00000000000000178 ) ) ;
#10650=ADVANCED_FACE ( 'NONE', ( #13420 ), #592, .F. ) ;
#10651=CARTESIAN_POINT ( 'NONE',  ( 6.917888187663118416, 52.54657765281190507, 10.49999999999999822 ) ) ;
#10654=AXIS2_PLACEMENT_3D ( 'NONE', #12987, #2578, #7194 ) ;
#10655=DIRECTION ( 'NONE',  ( -1.000000000000000000, 0.000000000000000000, 0.000000000000000000 ) ) ;
#10656=VECTOR ( 'NONE', #7039, 1000.000000000000000 ) ;
#10659=EDGE_CURVE ( 'NONE', #10704, #13133, #14487, .T. ) ;
#10660=ORIENTED_EDGE ( 'NONE', *, *, #6328, .T. ) ;
#10664=CARTESIAN_POINT ( 'NONE',  ( -37.71449950290985953, 86.67575032682117353, -13.00000000000000178 ) ) ;
#10665=CARTESIAN_POINT ( 'NONE',  ( 0.000000000000000000, 0.000000000000000000, -8.000000000000000000 ) ) ;
#10667=LINE ( 'NONE', #1568, #624 ) ;
#10668=AXIS2_PLACEMENT_3D ( 'NONE', #14828, #2068, #12472 ) ;
#10669=VERTEX_POINT ( 'NONE', #2866 ) ;
#10670=VERTEX_POINT ( 'NONE', #11301 ) ;
#10672=ORIENTED_EDGE ( 'NONE', *, *, #6202, .T. ) ;
#10673=ORIENTED_EDGE ( 'NONE', *, *, #252, .F. ) ;
#10675=DIRECTION ( 'NONE',  ( 0.000000000000000000, 0.000000000000000000, 1.000000000000000000 ) ) ;
#10676=DIRECTION ( 'NONE',  ( 1.000000000000000000, 0.000000000000000000, -0.000000000000000000 ) ) ;
#10678=VERTEX_POINT ( 'NONE', #1949 ) ;
#10679=CIRCLE ( 'NONE', #10205, 53.55662432702593634 ) ;
#10680=ORIENTED_EDGE ( 'NONE', *, *, #6776, .T. ) ;
#10681=CARTESIAN_POINT ( 'NONE',  ( 0.000000000000000000, 0.000000000000000000, -13.00000000000000178 ) ) ;
#10682=CIRCLE ( 'NONE', #7270, 3.000000000000002665 ) ;
#10684=AXIS2_PLACEMENT_3D ( 'NONE', #1978, #2057, #10104 ) ;
#10686=DIRECTION ( 'NONE',  ( 0.000000000000000000, 0.000000000000000000, 1.000000000000000000 ) ) ;
#10687=CARTESIAN_POINT ( 'NONE',  ( -11.55014193876141171, 53.26842454702440222, 8.000000000000000000 ) ) ;
#10688=CARTESIAN_POINT ( 'NONE',  ( -33.48561063518626923, 47.21331623427104063, -13.00000000000000178 ) ) ;
#10689=AXIS2_PLACEMENT_3D ( 'NONE', #12685, #13906, #11480 ) ;
#10690=EDGE_LOOP ( 'NONE', ( #12969, #9920, #7681, #9414, #5124, #13717 ) ) ;
#10691=DIRECTION ( 'NONE',  ( 0.000000000000000000, 0.000000000000000000, -1.000000000000000000 ) ) ;
#10692=CIRCLE ( 'NONE', #6562, 0.5000000000000038858 ) ;
#10693=DIRECTION ( 'NONE',  ( 0.000000000000000000, 0.000000000000000000, 1.000000000000000000 ) ) ;
#10694=ORIENTED_EDGE ( 'NONE', *, *, #5681, .T. ) ;
#10696=CARTESIAN_POINT ( 'NONE',  ( -12.86891638962156215, 56.43380494353993271, -13.00000000000000178 ) ) ;
#10697=AXIS2_PLACEMENT_3D ( 'NONE', #4891, #11588, #9420 ) ;
#10698=VERTEX_POINT ( 'NONE', #3022 ) ;
#10700=EDGE_LOOP ( 'NONE', ( #8935, #5972, #2896, #1420, #10025 ) ) ;
#10702=EDGE_CURVE ( 'NONE', #13295, #5812, #6646, .T. ) ;
#10704=VERTEX_POINT ( 'NONE', #13275 ) ;
#10706=DIRECTION ( 'NONE',  ( 1.000000000000000000, 0.000000000000000000, 0.000000000000000000 ) ) ;
#10708=CIRCLE ( 'NONE', #1985, 59.50000000000000000 ) ;
#10709=DIRECTION ( 'NONE',  ( 0.000000000000000000, 0.000000000000000000, -1.000000000000000000 ) ) ;
#10710=DIRECTION ( 'NONE',  ( 0.000000000000000000, 0.000000000000000000, 1.000000000000000000 ) ) ;
#10711=DIRECTION ( 'NONE',  ( 0.000000000000000000, 0.000000000000000000, -1.000000000000000000 ) ) ;
#10713=DIRECTION ( 'NONE',  ( 0.000000000000000000, 0.000000000000000000, 1.000000000000000000 ) ) ;
#10714=ORIENTED_EDGE ( 'NONE', *, *, #5096, .T. ) ;
#10717=ORIENTED_EDGE ( 'NONE', *, *, #2963, .T. ) ;
#10719=LINE ( 'NONE', #7060, #6442 ) ;
#10722=DIRECTION ( 'NONE',  ( 0.000000000000000000, 0.000000000000000000, -1.000000000000000000 ) ) ;
#10723=EDGE_CURVE ( 'NONE', #571, #12166, #8780, .T. ) ;
#10724=CARTESIAN_POINT ( 'NONE',  ( -68.68541276968778675, 69.08004447556137961, -13.00000000000000178 ) ) ;
#10727=ORIENTED_EDGE ( 'NONE', *, *, #5474, .T. ) ;
#10729=CARTESIAN_POINT ( 'NONE',  ( 0.000000000000000000, 0.000000000000000000, -8.000000000000000000 ) ) ;
#10735=DIRECTION ( 'NONE',  ( 1.000000000000000000, 0.000000000000000000, 0.000000000000000000 ) ) ;
#10736=PLANE ( 'NONE',  #5212 ) ;
#10737=VECTOR ( 'NONE', #14695, 1000.000000000000000 ) ;
#10738=DIRECTION ( 'NONE',  ( -1.000000000000000000, 0.000000000000000000, 0.000000000000000000 ) ) ;
#10739=ORIENTED_EDGE ( 'NONE', *, *, #14758, .F. ) ;
#10742=AXIS2_PLACEMENT_3D ( 'NONE', #2011, #13479, #7626 ) ;
#10744=ADVANCED_FACE ( 'NONE', ( #14784 ), #824, .T. ) ;
#10746=EDGE_LOOP ( 'NONE', ( #3750, #6581, #3466, #9295 ) ) ;
#10747=EDGE_CURVE ( 'NONE', #14193, #12545, #1095, .T. ) ;
#10748=AXIS2_PLACEMENT_3D ( 'NONE', #7178, #2791, #13269 ) ;
#10749=DIRECTION ( 'NONE',  ( 0.000000000000000000, 0.000000000000000000, 1.000000000000000000 ) ) ;
#10751=DIRECTION ( 'NONE',  ( 0.000000000000000000, 0.000000000000000000, 1.000000000000000000 ) ) ;
#10753=EDGE_CURVE ( 'NONE', #8417, #1677, #10538, .T. ) ;
#10754=DIRECTION ( 'NONE',  ( 0.000000000000000000, 0.000000000000000000, 1.000000000000000000 ) ) ;
#10755=CARTESIAN_POINT ( 'NONE',  ( -49.00442420935969778, 30.80502811811250297, -8.000000000000000000 ) ) ;
#10756=AXIS2_PLACEMENT_3D ( 'NONE', #13628, #5356, #9984 ) ;
#10760=DIRECTION ( 'NONE',  ( 1.000000000000000000, 0.000000000000000000, 0.000000000000000000 ) ) ;
#10761=VERTEX_POINT ( 'NONE', #10992 ) ;
#10763=VECTOR ( 'NONE', #12030, 1000.000000000000000 ) ;
#10764=CIRCLE ( 'NONE', #6886, 20.00000000000000000 ) ;
#10765=CARTESIAN_POINT ( 'NONE',  ( 57.06275842387049835, -9.706953719245678514, -8.000000000000000000 ) ) ;
#10766=AXIS2_PLACEMENT_3D ( 'NONE', #10039, #870, #9805 ) ;
#10767=CARTESIAN_POINT ( 'NONE',  ( -0.2790467552932217599, 96.58511096861892042, -13.00000000000000178 ) ) ;
#10768=DIRECTION ( 'NONE',  ( 1.000000000000000000, 0.000000000000000000, 0.000000000000000000 ) ) ;
#10770=CARTESIAN_POINT ( 'NONE',  ( 36.14014761921570340, 11.74264578624841171, -28.00000000000000000 ) ) ;
#10771=DIRECTION ( 'NONE',  ( 0.000000000000000000, 0.000000000000000000, 1.000000000000000000 ) ) ;
#10773=CARTESIAN_POINT ( 'NONE',  ( 2.449293598294700991E-16, -97.00000000000000000, -13.00000000000000178 ) ) ;
#10774=AXIS2_PLACEMENT_3D ( 'NONE', #11709, #4867, #9481 ) ;
#10775=EDGE_LOOP ( 'NONE', ( #4097, #14422, #5647, #58, #8071, #2795 ) ) ;
#10776=AXIS2_PLACEMENT_3D ( 'NONE', #7562, #14564, #6489 ) ;
#10777=ORIENTED_EDGE ( 'NONE', *, *, #7268, .F. ) ;
#10779=DIRECTION ( 'NONE',  ( 0.000000000000000000, 0.000000000000000000, 1.000000000000000000 ) ) ;
#10780=DIRECTION ( 'NONE',  ( -1.000000000000000000, 0.000000000000000000, 0.000000000000000000 ) ) ;
#10781=CIRCLE ( 'NONE', #3034, 0.5000000000000004441 ) ;
#10782=AXIS2_PLACEMENT_3D ( 'NONE', #583, #9834, #11294 ) ;
#10784=CARTESIAN_POINT ( 'NONE',  ( 0.000000000000000000, 0.000000000000000000, -10.50000000000000000 ) ) ;
#10785=CARTESIAN_POINT ( 'NONE',  ( 0.000000000000000000, 0.000000000000000000, -10.50000000000000000 ) ) ;
#10787=EDGE_CURVE ( 'NONE', #13104, #14416, #2529, .T. ) ;
#10788=AXIS2_PLACEMENT_3D ( 'NONE', #12918, #7052, #3437 ) ;
#10789=DIRECTION ( 'NONE',  ( 0.000000000000000000, 0.000000000000000000, 1.000000000000000000 ) ) ;
#10790=ORIENTED_EDGE ( 'NONE', *, *, #6420, .F. ) ;
#10791=EDGE_CURVE ( 'NONE', #14250, #10988, #12490, .T. ) ;
#10792=DIRECTION ( 'NONE',  ( 1.000000000000000000, 0.000000000000000000, 0.000000000000000000 ) ) ;
#10794=ORIENTED_EDGE ( 'NONE', *, *, #9144, .T. ) ;
#10796=CARTESIAN_POINT ( 'NONE',  ( 45.89934640057532533, -26.49999999999987566, -13.00000000000000178 ) ) ;
#10798=AXIS2_PLACEMENT_3D ( 'NONE', #11771, #8113, #14964 ) ;
#10799=CARTESIAN_POINT ( 'NONE',  ( -33.48561063518626923, 47.21331623427104063, -8.000000000000000000 ) ) ;
#10802=ORIENTED_EDGE ( 'NONE', *, *, #8286, .F. ) ;
#10803=ORIENTED_EDGE ( 'NONE', *, *, #2296, .F. ) ;
#10804=EDGE_CURVE ( 'NONE', #7348, #10294, #4246, .T. ) ;
#10805=DIRECTION ( 'NONE',  ( -0.000000000000000000, -0.000000000000000000, -1.000000000000000000 ) ) ;
#10806=CARTESIAN_POINT ( 'NONE',  ( 89.61631465359468507, -37.12029293941410657, 8.000000000000000000 ) ) ;
#10807=AXIS2_PLACEMENT_3D ( 'NONE', #10894, #498, #9745 ) ;
#10808=AXIS2_PLACEMENT_3D ( 'NONE', #11238, #6662, #10316 ) ;
#10810=DIRECTION ( 'NONE',  ( 0.000000000000000000, 0.000000000000000000, -1.000000000000000000 ) ) ;
#10811=EDGE_CURVE ( 'NONE', #2518, #4822, #852, .T. ) ;
#10812=EDGE_CURVE ( 'NONE', #14416, #13104, #9551, .T. ) ;
#10814=ORIENTED_EDGE ( 'NONE', *, *, #11333, .T. ) ;
#10815=CARTESIAN_POINT ( 'NONE',  ( 0.000000000000000000, 0.000000000000000000, -10.50000000000000000 ) ) ;
#10816=DIRECTION ( 'NONE',  ( 1.000000000000000000, 0.000000000000000000, 0.000000000000000000 ) ) ;
#10817=LINE ( 'NONE', #418, #8542 ) ;
#10818=AXIS2_PLACEMENT_3D ( 'NONE', #2691, #2613, #13093 ) ;
#10819=VERTEX_POINT ( 'NONE', #4467 ) ;
#10820=CARTESIAN_POINT ( 'NONE',  ( -87.95718916809170196, 34.62083247296289557, 8.000000000000000000 ) ) ;
#10821=ORIENTED_EDGE ( 'NONE', *, *, #9620, .F. ) ;
#10822=FACE_OUTER_BOUND ( 'NONE', #12048, .T. ) ;
#10823=DIRECTION ( 'NONE',  ( -0.000000000000000000, -0.000000000000000000, 1.000000000000000000 ) ) ;
#10826=CARTESIAN_POINT ( 'NONE',  ( 68.01302780753354682, -65.64523757230297463, -13.00000000000000178 ) ) ;
#10828=ORIENTED_EDGE ( 'NONE', *, *, #9676, .F. ) ;
#10829=CARTESIAN_POINT ( 'NONE',  ( 97.50000000000000000, -3.384287605079545030E-13, -13.00000000000000178 ) ) ;
#10831=EDGE_CURVE ( 'NONE', #9394, #6432, #5914, .T. ) ;
#10833=ORIENTED_EDGE ( 'NONE', *, *, #6268, .T. ) ;
#10834=EDGE_CURVE ( 'NONE', #5876, #11296, #2253, .T. ) ;
#10836=CARTESIAN_POINT ( 'NONE',  ( -37.12029293941250074, 89.61631465359532456, -8.000000000000000000 ) ) ;
#10837=ORIENTED_EDGE ( 'NONE', *, *, #12268, .T. ) ;
#10838=DIRECTION ( 'NONE',  ( -1.000000000000000000, 0.000000000000000000, 0.000000000000000000 ) ) ;
#10839=EDGE_CURVE ( 'NONE', #12197, #14062, #6888, .T. ) ;
#10841=PLANE ( 'NONE',  #1952 ) ;
#10844=DIRECTION ( 'NONE',  ( -1.000000000000000000, 0.000000000000000000, 0.000000000000000000 ) ) ;
#10846=CARTESIAN_POINT ( 'NONE',  ( 26.00011991137315803, 45.91029614918951296, 10.49999999999999822 ) ) ;
#10849=ORIENTED_EDGE ( 'NONE', *, *, #9856, .F. ) ;
#10850=VERTEX_POINT ( 'NONE', #2328 ) ;
#10851=CARTESIAN_POINT ( 'NONE',  ( -70.71067811865387398, 70.71067811865562192, 8.000000000000000000 ) ) ;
#10852=DIRECTION ( 'NONE',  ( -1.000000000000000000, 0.000000000000000000, 0.000000000000000000 ) ) ;
#10853=ADVANCED_FACE ( 'NONE', ( #10443 ), #46, .T. ) ;
#10856=CYLINDRICAL_SURFACE ( 'NONE', #1479, 0.5000000000000004441 ) ;
#10858=CARTESIAN_POINT ( 'NONE',  ( 41.59008834022645829, 32.46576781417968505, 10.49999999999999822 ) ) ;
#10859=ORIENTED_EDGE ( 'NONE', *, *, #7489, .F. ) ;
#10860=CARTESIAN_POINT ( 'NONE',  ( -6.917888187662729393, -52.54657765281195481, -8.000000000000000000 ) ) ;
#10861=ORIENTED_EDGE ( 'NONE', *, *, #11049, .F. ) ;
#10862=DIRECTION ( 'NONE',  ( -1.000000000000000000, 0.000000000000000000, 0.000000000000000000 ) ) ;
#10863=CARTESIAN_POINT ( 'NONE',  ( -91.27544013909712817, 39.61975340586647576, 8.000000000000000000 ) ) ;
#10864=VERTEX_POINT ( 'NONE', #1266 ) ;
#10865=DIRECTION ( 'NONE',  ( -1.000000000000000000, -1.065907399692639811E-13, 0.000000000000000000 ) ) ;
#10866=DIRECTION ( 'NONE',  ( -1.000000000000000000, 0.000000000000000000, 0.000000000000000000 ) ) ;
#10867=ORIENTED_EDGE ( 'NONE', *, *, #8788, .F. ) ;
#10868=DIRECTION ( 'NONE',  ( 0.000000000000000000, 0.000000000000000000, 1.000000000000000000 ) ) ;
#10871=FACE_OUTER_BOUND ( 'NONE', #2024, .T. ) ;
#10872=CARTESIAN_POINT ( 'NONE',  ( -33.29654390035820910, 41.94820822869202459, -10.50000000000000000 ) ) ;
#10874=DIRECTION ( 'NONE',  ( 0.000000000000000000, 0.000000000000000000, 1.000000000000000000 ) ) ;
#10875=DIRECTION ( 'NONE',  ( 1.000000000000000000, 1.826024711554534012E-15, 0.000000000000000000 ) ) ;
#10877=DIRECTION ( 'NONE',  ( 1.000000000000000000, 0.000000000000000000, 0.000000000000000000 ) ) ;
#10878=CYLINDRICAL_SURFACE ( 'NONE', #6405, 56.99999999999998579 ) ;
#10879=DIRECTION ( 'NONE',  ( 0.000000000000000000, 0.000000000000000000, -1.000000000000000000 ) ) ;
#10880=ADVANCED_FACE ( 'NONE', ( #12804 ), #2391, .F. ) ;
#10882=ADVANCED_FACE ( 'NONE', ( #14165 ), #12254, .T. ) ;
#10883=ORIENTED_EDGE ( 'NONE', *, *, #11687, .T. ) ;
#10887=EDGE_LOOP ( 'NONE', ( #6840, #8086, #14052, #7790 ) ) ;
#10888=ADVANCED_FACE ( 'NONE', ( #14521 ), #5261, .F. ) ;
#10889=CARTESIAN_POINT ( 'NONE',  ( 0.000000000000000000, 0.000000000000000000, -25.50000000000000355 ) ) ;
#10890=LINE ( 'NONE', #8682, #9730 ) ;
#10891=CARTESIAN_POINT ( 'NONE',  ( 12.86891638962116247, -56.43380494354001087, -10.50000000000000000 ) ) ;
#10894=CARTESIAN_POINT ( 'NONE',  ( -13.71740939043329277, 51.19406879332069593, -8.000000000000000000 ) ) ;
#10895=EDGE_CURVE ( 'NONE', #8551, #1906, #9785, .T. ) ;
#10899=CARTESIAN_POINT ( 'NONE',  ( 36.70371619500516402, 89.33979373934434420, -10.50000000000000000 ) ) ;
#10900=AXIS2_PLACEMENT_3D ( 'NONE', #4417, #1751, #14504 ) ;
#10901=FACE_OUTER_BOUND ( 'NONE', #630, .T. ) ;
#10902=DIRECTION ( 'NONE',  ( 0.5000000000000009992, -6.123233995736778362E-17, 0.8660254037844380415 ) ) ;
#10903=ORIENTED_EDGE ( 'NONE', *, *, #9613, .T. ) ;
#10906=ORIENTED_EDGE ( 'NONE', *, *, #14202, .T. ) ;
#10907=CIRCLE ( 'NONE', #11648, 3.000000000000004441 ) ;
#10908=AXIS2_PLACEMENT_3D ( 'NONE', #3606, #14075, #9212 ) ;
#10910=AXIS2_PLACEMENT_3D ( 'NONE', #14997, #8218, #14073 ) ;
#10911=ADVANCED_FACE ( 'NONE', ( #8395 ), #2622, .T. ) ;
#10912=AXIS2_PLACEMENT_3D ( 'NONE', #9342, #5849, #4729 ) ;
#10914=ORIENTED_EDGE ( 'NONE', *, *, #4652, .F. ) ;
#10915=DIRECTION ( 'NONE',  ( 0.000000000000000000, 0.000000000000000000, 1.000000000000000000 ) ) ;
#10916=DIRECTION ( 'NONE',  ( 0.000000000000000000, 0.000000000000000000, 1.000000000000000000 ) ) ;
#10919=CIRCLE ( 'NONE', #1713, 56.99999999999999289 ) ;
#10921=CIRCLE ( 'NONE', #8489, 60.50000000000000000 ) ;
#10924=CYLINDRICAL_SURFACE ( 'NONE', #1357, 59.50000000000000711 ) ;
#10926=CIRCLE ( 'NONE', #3417, 3.000000000000002665 ) ;
#10927=EDGE_CURVE ( 'NONE', #11092, #10391, #9564, .T. ) ;
#10928=AXIS2_PLACEMENT_3D ( 'NONE', #207, #8478, #6123 ) ;
#10930=DIRECTION ( 'NONE',  ( -0.000000000000000000, -0.000000000000000000, 1.000000000000000000 ) ) ;
#10931=DIRECTION ( 'NONE',  ( 1.000000000000000000, 0.000000000000000000, 0.000000000000000000 ) ) ;
#10933=AXIS2_PLACEMENT_3D ( 'NONE', #8089, #5883, #10445 ) ;
#10934=CARTESIAN_POINT ( 'NONE',  ( 69.16568774265594755, -71.53347797788796925, -13.00000000000000178 ) ) ;
#10935=AXIS2_PLACEMENT_3D ( 'NONE', #10082, #9921, #14571 ) ;
#10936=ORIENTED_EDGE ( 'NONE', *, *, #6862, .T. ) ;
#10938=ORIENTED_EDGE ( 'NONE', *, *, #9164, .T. ) ;
#10939=ADVANCED_FACE ( 'NONE', ( #1488 ), #11034, .T. ) ;
#10941=DIRECTION ( 'NONE',  ( -0.000000000000000000, -0.000000000000000000, -1.000000000000000000 ) ) ;
#10942=AXIS2_PLACEMENT_3D ( 'NONE', #12520, #9806, #10875 ) ;
#10946=CARTESIAN_POINT ( 'NONE',  ( -90.10640870805754332, -37.02125851216322872, -13.00000000000000178 ) ) ;
#10947=VECTOR ( 'NONE', #12493, 1000.000000000000000 ) ;
#10948=ORIENTED_EDGE ( 'NONE', *, *, #11876, .T. ) ;
#10949=DIRECTION ( 'NONE',  ( 0.000000000000000000, 0.000000000000000000, 1.000000000000000000 ) ) ;
#10953=CARTESIAN_POINT ( 'NONE',  ( -36.70371619500578220, -89.33979373934407420, -13.00000000000000178 ) ) ;
#10954=PLANE ( 'NONE',  #4923 ) ;
#10955=AXIS2_PLACEMENT_3D ( 'NONE', #10040, #12328, #4356 ) ;
#10956=DIRECTION ( 'NONE',  ( -0.000000000000000000, -0.000000000000000000, 1.000000000000000000 ) ) ;
#10957=FACE_OUTER_BOUND ( 'NONE', #11254, .T. ) ;
#10958=DIRECTION ( 'NONE',  ( -1.000000000000000000, 0.000000000000000000, 0.000000000000000000 ) ) ;
#10960=ORIENTED_EDGE ( 'NONE', *, *, #9207, .T. ) ;
#10961=CIRCLE ( 'NONE', #3447, 0.5000000000000022204 ) ;
#10962=CARTESIAN_POINT ( 'NONE',  ( 37.62029293941316155, -89.61631465359504034, -10.50000000000000000 ) ) ;
#10965=ORIENTED_EDGE ( 'NONE', *, *, #8446, .F. ) ;
#10966=VECTOR ( 'NONE', #2768, 1000.000000000000000 ) ;
#10967=ORIENTED_EDGE ( 'NONE', *, *, #6657, .T. ) ;
#10969=ORIENTED_EDGE ( 'NONE', *, *, #4957, .T. ) ;
#10977=ORIENTED_EDGE ( 'NONE', *, *, #14991, .T. ) ;
#10979=EDGE_LOOP ( 'NONE', ( #8476, #7654, #13386, #3051, #9402, #6563, #2953, #8271, #9837 ) ) ;
#10981=EDGE_CURVE ( 'NONE', #9738, #2014, #7389, .T. ) ;
#10983=DIRECTION ( 'NONE',  ( 1.000000000000000000, 0.000000000000000000, 0.000000000000000000 ) ) ;
#10984=ADVANCED_FACE ( 'NONE', ( #7088 ), #2220, .F. ) ;
#10986=VERTEX_POINT ( 'NONE', #12619 ) ;
#10987=AXIS2_PLACEMENT_3D ( 'NONE', #809, #13404, #11207 ) ;
#10988=VERTEX_POINT ( 'NONE', #2067 ) ;
#10989=DIRECTION ( 'NONE',  ( -1.000000000000000000, 0.000000000000000000, 0.000000000000000000 ) ) ;
#10990=ORIENTED_EDGE ( 'NONE', *, *, #2721, .F. ) ;
#10991=AXIS2_PLACEMENT_3D ( 'NONE', #2099, #11135, #11065 ) ;
#10992=CARTESIAN_POINT ( 'NONE',  ( -100.0000000000000000, 1.047191897158270473E-12, 8.000000000000000000 ) ) ;
#10996=AXIS2_PLACEMENT_3D ( 'NONE', #10507, #4670, #2092 ) ;
#10997=CARTESIAN_POINT ( 'NONE',  ( -37.12029293941250074, 89.61631465359532456, 8.000000000000000000 ) ) ;
#10999=ORIENTED_EDGE ( 'NONE', *, *, #1034, .F. ) ;
#11000=ADVANCED_FACE ( 'NONE', ( #11338 ), #11257, .F. ) ;
#11003=ORIENTED_EDGE ( 'NONE', *, *, #2217, .T. ) ;
#11004=VERTEX_POINT ( 'NONE', #11185 ) ;
#11007=AXIS2_PLACEMENT_3D ( 'NONE', #10583, #182, #4815 ) ;
#11009=DIRECTION ( 'NONE',  ( 0.000000000000000000, 0.000000000000000000, 1.000000000000000000 ) ) ;
#11011=DIRECTION ( 'NONE',  ( 0.000000000000000000, 0.000000000000000000, 1.000000000000000000 ) ) ;
#11012=CARTESIAN_POINT ( 'NONE',  ( -36.70371619500578220, -89.33979373934407420, 10.49999999999999822 ) ) ;
#11016=CIRCLE ( 'NONE', #4731, 56.99999999999999289 ) ;
#11018=DIRECTION ( 'NONE',  ( 1.000000000000000000, 0.000000000000000000, 0.000000000000000000 ) ) ;
#11019=EDGE_CURVE ( 'NONE', #2144, #6138, #6902, .T. ) ;
#11020=DIRECTION ( 'NONE',  ( 1.000000000000000000, 0.000000000000000000, 0.000000000000000000 ) ) ;
#11021=EDGE_CURVE ( 'NONE', #7084, #8152, #5554, .T. ) ;
#11022=EDGE_CURVE ( 'NONE', #9994, #15024, #9799, .T. ) ;
#11025=ORIENTED_EDGE ( 'NONE', *, *, #5593, .T. ) ;
#11026=AXIS2_PLACEMENT_3D ( 'NONE', #10681, #291, #8410 ) ;
#11027=DIRECTION ( 'NONE',  ( 1.000000000000000000, 0.000000000000000000, 0.000000000000000000 ) ) ;
#11028=ORIENTED_EDGE ( 'NONE', *, *, #11417, .F. ) ;
#11029=AXIS2_PLACEMENT_3D ( 'NONE', #12202, #1574, #12058 ) ;
#11030=AXIS2_PLACEMENT_3D ( 'NONE', #7770, #12413, #8761 ) ;
#11033=ORIENTED_EDGE ( 'NONE', *, *, #4781, .F. ) ;
#11034=PLANE ( 'NONE',  #14919 ) ;
#11035=DIRECTION ( 'NONE',  ( 0.000000000000000000, 0.000000000000000000, 1.000000000000000000 ) ) ;
#11036=DIRECTION ( 'NONE',  ( 0.000000000000000000, 0.000000000000000000, 1.000000000000000000 ) ) ;
#11038=CARTESIAN_POINT ( 'NONE',  ( 9.706953719245472456, 57.06275842387054098, 10.49999999999999822 ) ) ;
#11039=CARTESIAN_POINT ( 'NONE',  ( 13.35619814848834075, -51.53979475227123430, -10.50000000000000000 ) ) ;
#11040=VERTEX_POINT ( 'NONE', #13766 ) ;
#11041=CARTESIAN_POINT ( 'NONE',  ( 47.21331623427115431, 33.48561063518610581, -13.00000000000000178 ) ) ;
#11042=AXIS2_PLACEMENT_3D ( 'NONE', #8212, #12849, #2443 ) ;
#11044=AXIS2_PLACEMENT_3D ( 'NONE', #4369, #3306, #954 ) ;
#11046=DIRECTION ( 'NONE',  ( 1.000000000000000000, 0.000000000000000000, 0.000000000000000000 ) ) ;
#11047=AXIS2_PLACEMENT_3D ( 'NONE', #14808, #11321, #7581 ) ;
#11048=EDGE_CURVE ( 'NONE', #2937, #14795, #5464, .T. ) ;
#11049=EDGE_CURVE ( 'NONE', #8993, #3488, #8602, .T. ) ;
#11050=DIRECTION ( 'NONE',  ( -0.000000000000000000, -0.000000000000000000, 1.000000000000000000 ) ) ;
#11051=ORIENTED_EDGE ( 'NONE', *, *, #12718, .T. ) ;
#11052=AXIS2_PLACEMENT_3D ( 'NONE', #3622, #14947, #12882 ) ;
#11053=DIRECTION ( 'NONE',  ( 0.000000000000000000, 0.000000000000000000, -1.000000000000000000 ) ) ;
#11054=ORIENTED_EDGE ( 'NONE', *, *, #12338, .T. ) ;
#11055=DIRECTION ( 'NONE',  ( 0.000000000000000000, 0.000000000000000000, 1.000000000000000000 ) ) ;
#11056=CARTESIAN_POINT ( 'NONE',  ( 0.000000000000000000, 0.000000000000000000, -10.50000000000000000 ) ) ;
#11058=DIRECTION ( 'NONE',  ( 1.000000000000000000, 0.000000000000000000, 0.000000000000000000 ) ) ;
#11060=ORIENTED_EDGE ( 'NONE', *, *, #2649, .T. ) ;
#11061=VERTEX_POINT ( 'NONE', #7973 ) ;
#11062=CIRCLE ( 'NONE', #13251, 3.000000000000002665 ) ;
#11064=CARTESIAN_POINT ( 'NONE',  ( 86.67575032682076142, 37.71449950291080455, 8.000000000000000000 ) ) ;
#11065=DIRECTION ( 'NONE',  ( 1.000000000000000000, 0.000000000000000000, -0.000000000000000000 ) ) ;
#11067=ORIENTED_EDGE ( 'NONE', *, *, #8762, .T. ) ;
#11070=AXIS2_PLACEMENT_3D ( 'NONE', #169, #3745, #1458 ) ;
#11071=DIRECTION ( 'NONE',  ( 0.000000000000000000, 0.000000000000000000, 1.000000000000000000 ) ) ;
#11073=CARTESIAN_POINT ( 'NONE',  ( 47.21331623427115431, 33.48561063518610581, -10.50000000000000000 ) ) ;
#11075=ORIENTED_EDGE ( 'NONE', *, *, #3879, .T. ) ;
#11076=DIRECTION ( 'NONE',  ( -0.000000000000000000, -0.000000000000000000, 1.000000000000000000 ) ) ;
#11077=DIRECTION ( 'NONE',  ( -1.000000000000000000, 0.000000000000000000, 0.000000000000000000 ) ) ;
#11078=VERTEX_POINT ( 'NONE', #14905 ) ;
#11079=DIRECTION ( 'NONE',  ( -1.000000000000000000, 0.000000000000000000, 0.000000000000000000 ) ) ;
#11080=AXIS2_PLACEMENT_3D ( 'NONE', #4960, #3822, #4884 ) ;
#11081=VERTEX_POINT ( 'NONE', #4429 ) ;
#11084=ADVANCED_FACE ( 'NONE', ( #13682 ), #3284, .F. ) ;
#11085=EDGE_CURVE ( 'NONE', #8383, #14537, #2542, .T. ) ;
#11086=ADVANCED_FACE ( 'NONE', ( #3354 ), #8816, .T. ) ;
#11087=DIRECTION ( 'NONE',  ( -1.000000000000000000, 0.000000000000000000, 0.000000000000000000 ) ) ;
#11089=FACE_OUTER_BOUND ( 'NONE', #6554, .T. ) ;
#11090=LINE ( 'NONE', #6507, #13099 ) ;
#11092=VERTEX_POINT ( 'NONE', #7 ) ;
#11094=EDGE_CURVE ( 'NONE', #9519, #2565, #3528, .T. ) ;
#11095=CARTESIAN_POINT ( 'NONE',  ( 22.33583958711425055, -30.74264578624780597, -28.00000000000000000 ) ) ;
#11096=ORIENTED_EDGE ( 'NONE', *, *, #8873, .F. ) ;
#11097=CARTESIAN_POINT ( 'NONE',  ( -45.91029614918924295, 26.00011991137363765, -13.00000000000000178 ) ) ;
#11098=FACE_OUTER_BOUND ( 'NONE', #2472, .T. ) ;
#11100=PRESENTATION_STYLE_ASSIGNMENT (( #6449 ) ) ;
#11101=CARTESIAN_POINT ( 'NONE',  ( -94.51066581171356518, -1.674280531758327140, -13.00000000000000178 ) ) ;
#11102=AXIS2_PLACEMENT_3D ( 'NONE', #7877, #6724, #2266 ) ;
#11103=EDGE_LOOP ( 'NONE', ( #9440, #5459, #6744, #10539, #4177 ) ) ;
#11104=DIRECTION ( 'NONE',  ( 0.000000000000000000, 0.000000000000000000, 1.000000000000000000 ) ) ;
#11105=VERTEX_POINT ( 'NONE', #10484 ) ;
#11107=CARTESIAN_POINT ( 'NONE',  ( 27.01438936481372721, 47.21331623427104063, 10.49999999999999822 ) ) ;
#11108=CARTESIAN_POINT ( 'NONE',  ( 0.000000000000000000, 0.000000000000000000, 13.00000000000000178 ) ) ;
#11109=CARTESIAN_POINT ( 'NONE',  ( -26.49999999999971578, -45.89934640057541060, -13.00000000000000178 ) ) ;
#11110=ADVANCED_FACE ( 'NONE', ( #12998 ), #14978, .T. ) ;
#11111=DIRECTION ( 'NONE',  ( 0.000000000000000000, 0.000000000000000000, 1.000000000000000000 ) ) ;
#11112=DIRECTION ( 'NONE',  ( 1.000000000000000000, 0.000000000000000000, 0.000000000000000000 ) ) ;
#11113=AXIS2_PLACEMENT_3D ( 'NONE', #10755, #13192, #4081 ) ;
#11114=ADVANCED_FACE ( 'NONE', ( #5991 ), #8057, .F. ) ;
#11115=ORIENTED_EDGE ( 'NONE', *, *, #2040, .F. ) ;
#11123=EDGE_LOOP ( 'NONE', ( #3124, #14088, #12443, #10124, #9674 ) ) ;
#11124=CYLINDRICAL_SURFACE ( 'NONE', #4493, 59.50000000000000000 ) ;
#11126=DIRECTION ( 'NONE',  ( 0.000000000000000000, 0.000000000000000000, 1.000000000000000000 ) ) ;
#11128=DIRECTION ( 'NONE',  ( -1.000000000000000000, 0.000000000000000000, 0.000000000000000000 ) ) ;
#11130=EDGE_LOOP ( 'NONE', ( #2523, #10439, #7116, #10777 ) ) ;
#11131=VERTEX_POINT ( 'NONE', #3586 ) ;
#11132=ORIENTED_EDGE ( 'NONE', *, *, #11520, .T. ) ;
#11133=CARTESIAN_POINT ( 'NONE',  ( -51.19406879332065330, -13.71740939043347041, 8.000000000000000000 ) ) ;
#11135=DIRECTION ( 'NONE',  ( 0.000000000000000000, 0.000000000000000000, 1.000000000000000000 ) ) ;
#11136=ORIENTED_EDGE ( 'NONE', *, *, #3332, .T. ) ;
#11137=ADVANCED_FACE ( 'NONE', ( #3655 ), #13838, .T. ) ;
#11138=AXIS2_PLACEMENT_3D ( 'NONE', #2050, #9023, #13584 ) ;
#11139=ORIENTED_EDGE ( 'NONE', *, *, #11689, .T. ) ;
#11141=CARTESIAN_POINT ( 'NONE',  ( 23.51438936481372366, 47.21331623427104063, -13.00000000000000178 ) ) ;
#11143=EDGE_CURVE ( 'NONE', #406, #11311, #2428, .T. ) ;
#11144=DIRECTION ( 'NONE',  ( 0.000000000000000000, 0.000000000000000000, 1.000000000000000000 ) ) ;
#11146=VECTOR ( 'NONE', #12457, 1000.000000000000000 ) ;
#11147=CARTESIAN_POINT ( 'NONE',  ( -15.88467684210512942, 49.11971303961693280, 8.000000000000000000 ) ) ;
#11148=DIRECTION ( 'NONE',  ( 1.000000000000000000, 0.000000000000000000, 0.000000000000000000 ) ) ;
#11149=ORIENTED_EDGE ( 'NONE', *, *, #7637, .F. ) ;
#11150=CARTESIAN_POINT ( 'NONE',  ( -38.26834323650970049, -92.38795325112837986, -8.000000000000000000 ) ) ;
#11151=ORIENTED_EDGE ( 'NONE', *, *, #11937, .T. ) ;
#11152=ORIENTED_EDGE ( 'NONE', *, *, #918, .F. ) ;
#11153=AXIS2_PLACEMENT_3D ( 'NONE', #4328, #8790, #11079 ) ;
#11155=ORIENTED_EDGE ( 'NONE', *, *, #14901, .F. ) ;
#11156=DIRECTION ( 'NONE',  ( 0.000000000000000000, 0.000000000000000000, 1.000000000000000000 ) ) ;
#11157=AXIS2_PLACEMENT_3D ( 'NONE', #3085, #10056, #14704 ) ;
#11160=CARTESIAN_POINT ( 'NONE',  ( 0.000000000000000000, 0.000000000000000000, -8.000000000000000000 ) ) ;
#11161=CARTESIAN_POINT ( 'NONE',  ( -48.19406879332065330, -13.71740939043347041, -13.00000000000000178 ) ) ;
#11162=DIRECTION ( 'NONE',  ( 1.000000000000000000, 0.000000000000000000, 0.000000000000000000 ) ) ;
#11163=CIRCLE ( 'NONE', #11895, 3.000000000000002665 ) ;
#11165=ORIENTED_EDGE ( 'NONE', *, *, #1747, .F. ) ;
#11166=EDGE_CURVE ( 'NONE', #9753, #9297, #14434, .T. ) ;
#11167=AXIS2_PLACEMENT_3D ( 'NONE', #7867, #13730, #4034 ) ;
#11170=CARTESIAN_POINT ( 'NONE',  ( 42.04772703543530099, 32.26435573746242369, 10.49999999999999822 ) ) ;
#11171=DIRECTION ( 'NONE',  ( 0.000000000000000000, 0.000000000000000000, 1.000000000000000000 ) ) ;
#11173=ORIENTED_EDGE ( 'NONE', *, *, #11085, .T. ) ;
#11175=EDGE_LOOP ( 'NONE', ( #5735, #3305, #9137, #12684 ) ) ;
#11176=AXIS2_PLACEMENT_3D ( 'NONE', #7030, #990, #13094 ) ;
#11177=FACE_OUTER_BOUND ( 'NONE', #13592, .T. ) ;
#11178=VERTEX_POINT ( 'NONE', #2361 ) ;
#11179=LINE ( 'NONE', #10029, #13105 ) ;
#11181=AXIS2_PLACEMENT_3D ( 'NONE', #11821, #3619, #9444 ) ;
#11182=ORIENTED_EDGE ( 'NONE', *, *, #10328, .F. ) ;
#11184=ORIENTED_EDGE ( 'NONE', *, *, #206, .T. ) ;
#11185=CARTESIAN_POINT ( 'NONE',  ( -24.99999999999972644, -43.30127018922209459, -8.000000000000000000 ) ) ;
#11186=DIRECTION ( 'NONE',  ( -0.000000000000000000, -0.000000000000000000, 1.000000000000000000 ) ) ;
#11188=DIRECTION ( 'NONE',  ( 1.000000000000000000, 0.000000000000000000, 0.000000000000000000 ) ) ;
#11189=CARTESIAN_POINT ( 'NONE',  ( 0.000000000000000000, 0.000000000000000000, -13.00000000000000178 ) ) ;
#11191=ORIENTED_EDGE ( 'NONE', *, *, #1376, .T. ) ;
#11193=DIRECTION ( 'NONE',  ( -1.000000000000000000, 1.776356839400250465E-15, 0.000000000000000000 ) ) ;
#11194=AXIS2_PLACEMENT_3D ( 'NONE', #9880, #476, #5039 ) ;
#11196=AXIS2_PLACEMENT_3D ( 'NONE', #3753, #11653, #10421 ) ;
#11199=ORIENTED_EDGE ( 'NONE', *, *, #5645, .T. ) ;
#11201=ORIENTED_EDGE ( 'NONE', *, *, #1289, .T. ) ;
#11203=DIRECTION ( 'NONE',  ( 0.000000000000000000, 0.000000000000000000, 1.000000000000000000 ) ) ;
#11206=AXIS2_PLACEMENT_3D ( 'NONE', #11390, #9174, #13818 ) ;
#11207=DIRECTION ( 'NONE',  ( -1.000000000000000000, 0.000000000000000000, 0.000000000000000000 ) ) ;
#11210=EDGE_LOOP ( 'NONE', ( #12071, #704, #12817, #13102, #11075 ) ) ;
#11211=VERTEX_POINT ( 'NONE', #10562 ) ;
#11215=EDGE_LOOP ( 'NONE', ( #11331, #9183, #189, #3729 ) ) ;
#11216=EDGE_CURVE ( 'NONE', #2876, #7167, #11634, .T. ) ;
#11218=AXIS2_PLACEMENT_3D ( 'NONE', #10806, #2608, #14230 ) ;
#11221=EDGE_CURVE ( 'NONE', #5777, #5446, #534, .T. ) ;
#11224=CARTESIAN_POINT ( 'NONE',  ( 0.000000000000000000, 0.000000000000000000, 8.000000000000000000 ) ) ;
#11226=DIRECTION ( 'NONE',  ( 0.000000000000000000, 0.000000000000000000, 1.000000000000000000 ) ) ;
#11228=ORIENTED_EDGE ( 'NONE', *, *, #1657, .F. ) ;
#11229=FACE_BOUND ( 'NONE', #13894, .T. ) ;
#11230=DIRECTION ( 'NONE',  ( 0.000000000000000000, 0.000000000000000000, 1.000000000000000000 ) ) ;
#11231=AXIS2_PLACEMENT_3D ( 'NONE', #10564, #14980, #7975 ) ;
#11232=ORIENTED_EDGE ( 'NONE', *, *, #7958, .T. ) ;
#11233=DIRECTION ( 'NONE',  ( 1.000000000000000000, 0.000000000000000000, 0.000000000000000000 ) ) ;
#11235=AXIS2_PLACEMENT_3D ( 'NONE', #3824, #14066, #7292 ) ;
#11236=EDGE_CURVE ( 'NONE', #14062, #8423, #3273, .T. ) ;
#11238=CARTESIAN_POINT ( 'NONE',  ( -30.80502811811232888, -49.00442420935981147, -8.000000000000000000 ) ) ;
#11239=AXIS2_PLACEMENT_3D ( 'NONE', #5172, #9789, #12090 ) ;
#11240=DIRECTION ( 'NONE',  ( 1.000000000000000000, 9.237055564881302416E-14, 0.000000000000000000 ) ) ;
#11241=VECTOR ( 'NONE', #12277, 1000.000000000000000 ) ;
#11243=DIRECTION ( 'NONE',  ( -0.000000000000000000, -0.000000000000000000, 1.000000000000000000 ) ) ;
#11245=AXIS2_PLACEMENT_3D ( 'NONE', #10330, #14032, #13590 ) ;
#11247=CARTESIAN_POINT ( 'NONE',  ( -12.86891638962156215, 56.43380494353993271, -13.00000000000000178 ) ) ;
#11249=DIRECTION ( 'NONE',  ( 1.000000000000000000, 0.000000000000000000, 0.000000000000000000 ) ) ;
#11250=CIRCLE ( 'NONE', #2504, 56.99999999999999289 ) ;
#11251=ORIENTED_EDGE ( 'NONE', *, *, #6372, .T. ) ;
#11253=DIRECTION ( 'NONE',  ( -1.000000000000000000, 0.000000000000000000, 0.000000000000000000 ) ) ;
#11254=EDGE_LOOP ( 'NONE', ( #9755, #4316, #5783, #3629 ) ) ;
#11255=CARTESIAN_POINT ( 'NONE',  ( -9.706953719245875689, -57.06275842387046993, -10.50000000000000000 ) ) ;
#11256=CIRCLE ( 'NONE', #1319, 3.000000000000002665 ) ;
#11257=PLANE ( 'NONE',  #611 ) ;
#11258=PLANE ( 'NONE',  #2189 ) ;
#11259=EDGE_CURVE ( 'NONE', #1589, #13568, #3880, .T. ) ;
#11260=CARTESIAN_POINT ( 'NONE',  ( 45.83364790889049090, -29.49928053175916887, 8.000000000000000000 ) ) ;
#11261=VECTOR ( 'NONE', #9794, 1000.000000000000000 ) ;
#11264=CARTESIAN_POINT ( 'NONE',  ( 45.96504489226007450, -23.50071946824056823, -13.00000000000000178 ) ) ;
#11265=DIRECTION ( 'NONE',  ( 1.000000000000000000, 0.000000000000000000, 0.000000000000000000 ) ) ;
#11268=DIRECTION ( 'NONE',  ( 0.000000000000000000, 0.000000000000000000, -1.000000000000000000 ) ) ;
#11269=CARTESIAN_POINT ( 'NONE',  ( -68.58935777509570642, -68.58935777509452691, -8.000000000000000000 ) ) ;
#11271=AXIS2_PLACEMENT_3D ( 'NONE', #11988, #8689, #13114 ) ;
#11275=DIRECTION ( 'NONE',  ( 0.000000000000000000, 0.000000000000000000, 1.000000000000000000 ) ) ;
#11276=ORIENTED_EDGE ( 'NONE', *, *, #13823, .T. ) ;
#11277=CARTESIAN_POINT ( 'NONE',  ( 49.57224306869054686, -6.526309611002390376, 8.000000000000000000 ) ) ;
#11280=EDGE_CURVE ( 'NONE', #14497, #218, #5213, .T. ) ;
#11281=DIRECTION ( 'NONE',  ( -1.000000000000000000, 0.000000000000000000, 0.000000000000000000 ) ) ;
#11284=AXIS2_PLACEMENT_3D ( 'NONE', #10836, #4298, #6335 ) ;
#11285=FACE_OUTER_BOUND ( 'NONE', #14653, .T. ) ;
#11286=DIRECTION ( 'NONE',  ( 1.000000000000000000, 0.000000000000000000, 0.000000000000000000 ) ) ;
#11291=AXIS2_PLACEMENT_3D ( 'NONE', #7904, #1908, #2137 ) ;
#11294=DIRECTION ( 'NONE',  ( -1.000000000000000000, -1.387778780781443624E-14, 0.000000000000000000 ) ) ;
#11296=VERTEX_POINT ( 'NONE', #2738 ) ;
#11297=CIRCLE ( 'NONE', #9093, 3.000000000000002665 ) ;
#11298=ORIENTED_EDGE ( 'NONE', *, *, #1944, .F. ) ;
#11299=AXIS2_PLACEMENT_3D ( 'NONE', #6065, #10709, #4948 ) ;
#11300=EDGE_LOOP ( 'NONE', ( #9602, #429, #13454, #8087, #5254, #1570, #5106, #2832, #8341 ) ) ;
#11301=CARTESIAN_POINT ( 'NONE',  ( 7.417888187663120192, 52.54657765281190507, 10.49999999999999822 ) ) ;
#11302=CARTESIAN_POINT ( 'NONE',  ( 32.46576781417953583, -41.59008834022656487, -10.50000000000000000 ) ) ;
#11303=DIRECTION ( 'NONE',  ( -1.000000000000000000, 0.000000000000000000, 0.000000000000000000 ) ) ;
#11305=AXIS2_PLACEMENT_3D ( 'NONE', #6186, #10751, #2625 ) ;
#11306=AXIS2_PLACEMENT_3D ( 'NONE', #6582, #985, #9015 ) ;
#11307=EDGE_LOOP ( 'NONE', ( #9790, #5800, #175, #12031, #8870, #580, #3548, #712, #10579 ) ) ;
#11311=VERTEX_POINT ( 'NONE', #2880 ) ;
#11313=EDGE_CURVE ( 'NONE', #12813, #1620, #12973, .T. ) ;
#11315=VERTEX_POINT ( 'NONE', #1748 ) ;
#11316=CARTESIAN_POINT ( 'NONE',  ( 69.16568774265594755, -71.53347797788796925, 8.000000000000000000 ) ) ;
#11317=CIRCLE ( 'NONE', #10818, 59.50000000000000000 ) ;
#11319=DIRECTION ( 'NONE',  ( 1.000000000000000000, 0.000000000000000000, 0.000000000000000000 ) ) ;
#11320=DIRECTION ( 'NONE',  ( -1.000000000000000000, 0.000000000000000000, 0.000000000000000000 ) ) ;
#11321=DIRECTION ( 'NONE',  ( 0.000000000000000000, 0.000000000000000000, 1.000000000000000000 ) ) ;
#11322=LINE ( 'NONE', #10095, #13332 ) ;
#11323=EDGE_CURVE ( 'NONE', #10864, #13229, #12266, .T. ) ;
#11324=DIRECTION ( 'NONE',  ( -0.000000000000000000, -0.000000000000000000, 1.000000000000000000 ) ) ;
#11326=VERTEX_POINT ( 'NONE', #13285 ) ;
#11327=VECTOR ( 'NONE', #14356, 1000.000000000000000 ) ;
#11328=DIRECTION ( 'NONE',  ( 1.000000000000000000, 0.000000000000000000, 0.000000000000000000 ) ) ;
#11329=CARTESIAN_POINT ( 'NONE',  ( 42.50536573064410106, 32.06294366074510549, 10.49999999999999822 ) ) ;
#11330=CARTESIAN_POINT ( 'NONE',  ( -36.52608637591512775, 92.55687898036946137, 8.000000000000000000 ) ) ;
#11331=ORIENTED_EDGE ( 'NONE', *, *, #5003, .F. ) ;
#11332=PLANE ( 'NONE',  #872 ) ;
#11333=EDGE_CURVE ( 'NONE', #8562, #452, #380, .T. ) ;
#11334=EDGE_LOOP ( 'NONE', ( #11401, #9462, #8035, #8755 ) ) ;
#11336=ORIENTED_EDGE ( 'NONE', *, *, #11502, .T. ) ;
#11337=CARTESIAN_POINT ( 'NONE',  ( -47.21331623427138879, -33.48561063518577896, 10.49999999999999822 ) ) ;
#11338=FACE_OUTER_BOUND ( 'NONE', #1214, .T. ) ;
#11339=CARTESIAN_POINT ( 'NONE',  ( 0.000000000000000000, 0.000000000000000000, 8.000000000000000000 ) ) ;
#11340=DIRECTION ( 'NONE',  ( 0.000000000000000000, 0.000000000000000000, 1.000000000000000000 ) ) ;
#11341=DIRECTION ( 'NONE',  ( 0.000000000000000000, 0.000000000000000000, 1.000000000000000000 ) ) ;
#11344=CYLINDRICAL_SURFACE ( 'NONE', #2341, 3.000000000000002665 ) ;
#11345=CARTESIAN_POINT ( 'NONE',  ( 2.649999999999987033, 38.00000000000000000, -28.00000000000000000 ) ) ;
#11346=FACE_OUTER_BOUND ( 'NONE', #7371, .T. ) ;
#11347=CARTESIAN_POINT ( 'NONE',  ( 97.41488903138106537, -0.2790467552935826934, -10.50000000000000000 ) ) ;
#11350=ORIENTED_EDGE ( 'NONE', *, *, #11166, .T. ) ;
#11351=DIRECTION ( 'NONE',  ( -1.000000000000000000, 0.000000000000000000, 0.000000000000000000 ) ) ;
#11352=DIRECTION ( 'NONE',  ( -1.000000000000000000, 2.653106492670410595E-15, 0.000000000000000000 ) ) ;
#11353=ORIENTED_EDGE ( 'NONE', *, *, #4130, .T. ) ;
#11354=AXIS2_PLACEMENT_3D ( 'NONE', #6032, #9240, #10676 ) ;
#11358=EDGE_LOOP ( 'NONE', ( #13505, #1819, #13324, #3498 ) ) ;
#11359=VERTEX_POINT ( 'NONE', #1526 ) ;
#11360=ORIENTED_EDGE ( 'NONE', *, *, #7452, .F. ) ;
#11364=EDGE_CURVE ( 'NONE', #5169, #11991, #139, .T. ) ;
#11365=DIRECTION ( 'NONE',  ( -0.000000000000000000, -0.000000000000000000, 1.000000000000000000 ) ) ;
#11366=EDGE_CURVE ( 'NONE', #11429, #6857, #11547, .T. ) ;
#11368=ORIENTED_EDGE ( 'NONE', *, *, #7489, .T. ) ;
#11369=ORIENTED_EDGE ( 'NONE', *, *, #1951, .F. ) ;
#11370=EDGE_CURVE ( 'NONE', #10704, #1787, #14694, .T. ) ;
#11371=VERTEX_POINT ( 'NONE', #9560 ) ;
#11375=CARTESIAN_POINT ( 'NONE',  ( 13.71740939043365337, -51.19406879332061067, 8.000000000000000000 ) ) ;
#11376=LINE ( 'NONE', #14790, #1767 ) ;
#11378=CARTESIAN_POINT ( 'NONE',  ( -3.492805317593278058, 46.55633131742322917, -10.50000000000000000 ) ) ;
#11379=ORIENTED_EDGE ( 'NONE', *, *, #13638, .F. ) ;
#11380=ORIENTED_EDGE ( 'NONE', *, *, #9314, .T. ) ;
#11381=LINE ( 'NONE', #2968, #12073 ) ;
#11383=ORIENTED_EDGE ( 'NONE', *, *, #14833, .T. ) ;
#11385=DIRECTION ( 'NONE',  ( 0.000000000000000000, 0.000000000000000000, 1.000000000000000000 ) ) ;
#11386=VERTEX_POINT ( 'NONE', #5470 ) ;
#11388=CARTESIAN_POINT ( 'NONE',  ( -52.54657765281192638, 6.917888187662934563, -8.000000000000000000 ) ) ;
#11389=CIRCLE ( 'NONE', #6755, 3.000000000000002665 ) ;
#11390=CARTESIAN_POINT ( 'NONE',  ( 12.86891638962116247, -56.43380494354001087, 8.000000000000000000 ) ) ;
#11391=CARTESIAN_POINT ( 'NONE',  ( 40.12029293941316155, -89.61631465359504034, -13.00000000000000178 ) ) ;
#11392=FACE_OUTER_BOUND ( 'NONE', #2166, .T. ) ;
#11393=FACE_OUTER_BOUND ( 'NONE', #8626, .T. ) ;
#11394=ORIENTED_EDGE ( 'NONE', *, *, #2118, .F. ) ;
#11395=DIRECTION ( 'NONE',  ( 1.000000000000000000, 0.000000000000000000, 0.000000000000000000 ) ) ;
#11396=AXIS2_PLACEMENT_3D ( 'NONE', #4854, #13210, #6270 ) ;
#11398=AXIS2_PLACEMENT_3D ( 'NONE', #14967, #1150, #8475 ) ;
#11399=DIRECTION ( 'NONE',  ( -0.000000000000000000, -0.000000000000000000, -1.000000000000000000 ) ) ;
#11400=CIRCLE ( 'NONE', #11890, 3.000000000000002665 ) ;
#11401=ORIENTED_EDGE ( 'NONE', *, *, #225, .F. ) ;
#11402=CARTESIAN_POINT ( 'NONE',  ( 69.08004447556065486, 68.68541276968852571, -13.00000000000000178 ) ) ;
#11403=ADVANCED_FACE ( 'NONE', ( #13581 ), #14661, .F. ) ;
#11405=ADVANCED_FACE ( 'NONE', ( #1894, #1969 ), #4335, .F. ) ;
#11408=EDGE_CURVE ( 'NONE', #219, #11737, #12029, .T. ) ;
#11409=DIRECTION ( 'NONE',  ( 0.000000000000000000, 0.000000000000000000, 1.000000000000000000 ) ) ;
#11410=AXIS2_PLACEMENT_3D ( 'NONE', #14231, #3831, #8449 ) ;
#11411=DIRECTION ( 'NONE',  ( 0.000000000000000000, 0.000000000000000000, -1.000000000000000000 ) ) ;
#11413=AXIS2_PLACEMENT_3D ( 'NONE', #2531, #1247, #12857 ) ;
#11414=CARTESIAN_POINT ( 'NONE',  ( 38.79014761921569487, 11.74264578624841171, -25.50000000000000355 ) ) ;
#11417=EDGE_CURVE ( 'NONE', #10986, #303, #12988, .T. ) ;
#11418=DIRECTION ( 'NONE',  ( 0.000000000000000000, 0.000000000000000000, 1.000000000000000000 ) ) ;
#11419=ORIENTED_EDGE ( 'NONE', *, *, #4574, .F. ) ;
#11421=DIRECTION ( 'NONE',  ( 1.000000000000000000, 0.000000000000000000, 0.000000000000000000 ) ) ;
#11422=CIRCLE ( 'NONE', #743, 0.5000000000000004441 ) ;
#11423=DIRECTION ( 'NONE',  ( 0.000000000000000000, 0.000000000000000000, 1.000000000000000000 ) ) ;
#11425=CARTESIAN_POINT ( 'NONE',  ( -89.61631465359519666, -37.12029293941281338, -10.50000000000000000 ) ) ;
#11426=AXIS2_PLACEMENT_3D ( 'NONE', #5694, #6743, #9113 ) ;
#11428=AXIS2_PLACEMENT_3D ( 'NONE', #4067, #7538, #2773 ) ;
#11429=VERTEX_POINT ( 'NONE', #6585 ) ;
#11431=EDGE_LOOP ( 'NONE', ( #632, #202, #12394, #4638 ) ) ;
#11432=DIRECTION ( 'NONE',  ( 0.000000000000000000, 0.000000000000000000, -1.000000000000000000 ) ) ;
#11433=DIRECTION ( 'NONE',  ( -1.000000000000000000, 0.000000000000000000, 0.000000000000000000 ) ) ;
#11434=AXIS2_PLACEMENT_3D ( 'NONE', #11927, #14199, #4022 ) ;
#11437=DIRECTION ( 'NONE',  ( 1.000000000000000000, 1.778456000581264310E-15, 0.000000000000000000 ) ) ;
#11440=ORIENTED_EDGE ( 'NONE', *, *, #14748, .T. ) ;
#11441=ORIENTED_EDGE ( 'NONE', *, *, #3201, .T. ) ;
#11443=CARTESIAN_POINT ( 'NONE',  ( 6.917888187663118416, 52.54657765281190507, -13.00000000000000178 ) ) ;
#11444=DIRECTION ( 'NONE',  ( 0.000000000000000000, 0.000000000000000000, 1.000000000000000000 ) ) ;
#11445=PLANE ( 'NONE',  #11706 ) ;
#11446=EDGE_LOOP ( 'NONE', ( #14708, #14800, #11383, #2100 ) ) ;
#11447=CIRCLE ( 'NONE', #764, 0.5000000000000004441 ) ;
#11448=ORIENTED_EDGE ( 'NONE', *, *, #3186, .T. ) ;
#11449=VERTEX_POINT ( 'NONE', #13509 ) ;
#11450=AXIS2_PLACEMENT_3D ( 'NONE', #10244, #6812, #14884 ) ;
#11454=CARTESIAN_POINT ( 'NONE',  ( 92.55687898036906347, 36.52608637591612961, -8.000000000000000000 ) ) ;
#11457=DIRECTION ( 'NONE',  ( 1.000000000000000000, 0.000000000000000000, 0.000000000000000000 ) ) ;
#11458=EDGE_CURVE ( 'NONE', #7611, #10669, #9021, .T. ) ;
#11460=AXIS2_PLACEMENT_3D ( 'NONE', #13245, #2840, #3981 ) ;
#11462=ORIENTED_EDGE ( 'NONE', *, *, #225, .T. ) ;
#11463=DIRECTION ( 'NONE',  ( 1.000000000000000000, 0.000000000000000000, 0.000000000000000000 ) ) ;
#11464=ORIENTED_EDGE ( 'NONE', *, *, #1001, .F. ) ;
#11465=AXIS2_PLACEMENT_3D ( 'NONE', #7955, #12533, #14963 ) ;
#11467=ORIENTED_EDGE ( 'NONE', *, *, #1728, .F. ) ;
#11469=VERTEX_POINT ( 'NONE', #766 ) ;
#11470=ORIENTED_EDGE ( 'NONE', *, *, #171, .F. ) ;
#11472=CARTESIAN_POINT ( 'NONE',  ( 56.43380494353997534, 12.86891638962136319, 8.000000000000000000 ) ) ;
#11473=AXIS2_PLACEMENT_3D ( 'NONE', #11808, #1403, #6011 ) ;
#11474=CYLINDRICAL_SURFACE ( 'NONE', #10798, 3.000000000000002665 ) ;
#11475=CARTESIAN_POINT ( 'NONE',  ( 19.68583958711426263, -30.74264578624780597, -28.00000000000000000 ) ) ;
#11476=EDGE_CURVE ( 'NONE', #11873, #4338, #8095, .T. ) ;
#11477=EDGE_CURVE ( 'NONE', #3464, #9394, #12712, .T. ) ;
#11478=CARTESIAN_POINT ( 'NONE',  ( 3.000000000000004885, -97.00000000000000000, 8.000000000000000000 ) ) ;
#11479=EDGE_LOOP ( 'NONE', ( #2234, #11051, #5578, #156, #13148 ) ) ;
#11480=DIRECTION ( 'NONE',  ( 1.000000000000000000, 0.000000000000000000, 0.000000000000000000 ) ) ;
#11481=ORIENTED_EDGE ( 'NONE', *, *, #1834, .T. ) ;
#11485=CIRCLE ( 'NONE', #11239, 0.5000000000000004441 ) ;
#11486=ORIENTED_EDGE ( 'NONE', *, *, #10332, .T. ) ;
#11487=DIRECTION ( 'NONE',  ( 0.000000000000000000, 0.000000000000000000, 1.000000000000000000 ) ) ;
#11488=EDGE_LOOP ( 'NONE', ( #2074, #4596, #3755, #5034 ) ) ;
#11489=CIRCLE ( 'NONE', #1538, 0.5000000000000022204 ) ;
#11491=CARTESIAN_POINT ( 'NONE',  ( -56.43380494354004639, -12.86891638962099549, 10.49999999999999822 ) ) ;
#11492=CIRCLE ( 'NONE', #11978, 3.000000000000002665 ) ;
#11495=DIRECTION ( 'NONE',  ( -0.000000000000000000, -0.000000000000000000, -1.000000000000000000 ) ) ;
#11497=ADVANCED_FACE ( 'NONE', ( #11089 ), #5394, .F. ) ;
#11498=CARTESIAN_POINT ( 'NONE',  ( 15.88467684210547226, -49.11971303961683333, -13.00000000000000178 ) ) ;
#11499=ADVANCED_FACE ( 'NONE', ( #5538 ), #13664, .F. ) ;
#11500=CIRCLE ( 'NONE', #8556, 0.5000000000000004441 ) ;
#11501=ORIENTED_EDGE ( 'NONE', *, *, #10424, .T. ) ;
#11502=EDGE_CURVE ( 'NONE', #6680, #10072, #6735, .T. ) ;
#11503=CARTESIAN_POINT ( 'NONE',  ( 45.83364790889049090, -29.49928053175917242, -8.000000000000000000 ) ) ;
#11505=EDGE_CURVE ( 'NONE', #6495, #9656, #6414, .T. ) ;
#11506=CARTESIAN_POINT ( 'NONE',  ( 87.95718916809192933, -34.62083247296232713, 8.000000000000000000 ) ) ;
#11508=DIRECTION ( 'NONE',  ( 0.000000000000000000, 0.000000000000000000, 1.000000000000000000 ) ) ;
#11509=EDGE_LOOP ( 'NONE', ( #13760, #7364, #8957, #6296 ) ) ;
#11510=CIRCLE ( 'NONE', #9065, 2.649999999999985700 ) ;
#11511=AXIS2_PLACEMENT_3D ( 'NONE', #13597, #14749, #13453 ) ;
#11513=DIRECTION ( 'NONE',  ( 0.000000000000000000, 0.000000000000000000, 1.000000000000000000 ) ) ;
#11514=AXIS2_PLACEMENT_3D ( 'NONE', #2610, #8304, #3832 ) ;
#11515=ORIENTED_EDGE ( 'NONE', *, *, #13917, .F. ) ;
#11516=CARTESIAN_POINT ( 'NONE',  ( -89.12622059913283579, -37.21932736666236963, -10.50000000000000000 ) ) ;
#11518=FACE_OUTER_BOUND ( 'NONE', #6093, .T. ) ;
#11519=ORIENTED_EDGE ( 'NONE', *, *, #13805, .T. ) ;
#11520=EDGE_CURVE ( 'NONE', #4183, #10362, #9339, .T. ) ;
#11522=ORIENTED_EDGE ( 'NONE', *, *, #3965, .T. ) ;
#11524=AXIS2_PLACEMENT_3D ( 'NONE', #2933, #5138, #6189 ) ;
#11527=FACE_OUTER_BOUND ( 'NONE', #13878, .T. ) ;
#11528=DIRECTION ( 'NONE',  ( 0.000000000000000000, 0.000000000000000000, -1.000000000000000000 ) ) ;
#11529=AXIS2_PLACEMENT_3D ( 'NONE', #6869, #8015, #8168 ) ;
#11530=CARTESIAN_POINT ( 'NONE',  ( 0.000000000000000000, 0.000000000000000000, 13.00000000000000178 ) ) ;
#11531=EDGE_LOOP ( 'NONE', ( #8854, #10501, #7334, #11992 ) ) ;
#11532=VERTEX_POINT ( 'NONE', #3637 ) ;
#11533=AXIS2_PLACEMENT_3D ( 'NONE', #1283, #8181, #10760 ) ;
#11534=ORIENTED_EDGE ( 'NONE', *, *, #14238, .F. ) ;
#11536=AXIS2_PLACEMENT_3D ( 'NONE', #6116, #3843, #5204 ) ;
#11537=CARTESIAN_POINT ( 'NONE',  ( 68.58935777509475429, -68.58935777509547904, -8.000000000000000000 ) ) ;
#11540=DIRECTION ( 'NONE',  ( 0.000000000000000000, 0.000000000000000000, 1.000000000000000000 ) ) ;
#11541=EDGE_LOOP ( 'NONE', ( #1559, #9500, #6479, #11467 ) ) ;
#11543=ORIENTED_EDGE ( 'NONE', *, *, #10451, .F. ) ;
#11544=FACE_OUTER_BOUND ( 'NONE', #13111, .T. ) ;
#11546=VERTEX_POINT ( 'NONE', #9251 ) ;
#11547=CIRCLE ( 'NONE', #620, 3.000000000000002665 ) ;
#11549=DIRECTION ( 'NONE',  ( 0.000000000000000000, 0.000000000000000000, -1.000000000000000000 ) ) ;
#11550=EDGE_CURVE ( 'NONE', #14062, #12763, #3049, .T. ) ;
#11551=VERTEX_POINT ( 'NONE', #5685 ) ;
#11553=VECTOR ( 'NONE', #13633, 1000.000000000000000 ) ;
#11554=DIRECTION ( 'NONE',  ( 0.000000000000000000, 0.000000000000000000, 1.000000000000000000 ) ) ;
#11555=DIRECTION ( 'NONE',  ( -0.000000000000000000, -0.000000000000000000, -1.000000000000000000 ) ) ;
#11557=FACE_OUTER_BOUND ( 'NONE', #14036, .T. ) ;
#11559=VERTEX_POINT ( 'NONE', #3570 ) ;
#11560=CARTESIAN_POINT ( 'NONE',  ( -13.71740939043329277, 51.19406879332069593, -13.00000000000000178 ) ) ;
#11561=VERTEX_POINT ( 'NONE', #8260 ) ;
#11562=CARTESIAN_POINT ( 'NONE',  ( 70.71067811865437136, -70.71067811865513875, -8.000000000000000000 ) ) ;
#11563=ORIENTED_EDGE ( 'NONE', *, *, #5416, .T. ) ;
#11564=AXIS2_PLACEMENT_3D ( 'NONE', #1258, #961, #5871 ) ;
#11567=EDGE_CURVE ( 'NONE', #5532, #10072, #13715, .T. ) ;
#11568=ORIENTED_EDGE ( 'NONE', *, *, #6202, .F. ) ;
#11569=DIRECTION ( 'NONE',  ( 0.000000000000000000, 0.000000000000000000, 1.000000000000000000 ) ) ;
#11570=ADVANCED_FACE ( 'NONE', ( #4630 ), #7956, .T. ) ;
#11571=EDGE_CURVE ( 'NONE', #215, #6876, #6911, .T. ) ;
#11573=CARTESIAN_POINT ( 'NONE',  ( -33.48561063518626923, 47.21331623427104063, -13.00000000000000178 ) ) ;
#11577=DIRECTION ( 'NONE',  ( -1.000000000000000000, 0.000000000000000000, 0.000000000000000000 ) ) ;
#11579=CIRCLE ( 'NONE', #1387, 63.00000000000000000 ) ;
#11580=DIRECTION ( 'NONE',  ( 1.000000000000000000, 0.000000000000000000, 0.000000000000000000 ) ) ;
#11581=CARTESIAN_POINT ( 'NONE',  ( -30.80502811811232888, -49.00442420935981147, 8.000000000000000000 ) ) ;
#11583=DIRECTION ( 'NONE',  ( 0.000000000000000000, 0.000000000000000000, 1.000000000000000000 ) ) ;
#11584=DIRECTION ( 'NONE',  ( 0.000000000000000000, 0.000000000000000000, 1.000000000000000000 ) ) ;
#11585=DIRECTION ( 'NONE',  ( 0.000000000000000000, 0.000000000000000000, -1.000000000000000000 ) ) ;
#11586=CARTESIAN_POINT ( 'NONE',  ( -33.49014761921588956, 11.74264578624790190, -25.50000000000000355 ) ) ;
#11587=ORIENTED_EDGE ( 'NONE', *, *, #546, .F. ) ;
#11588=DIRECTION ( 'NONE',  ( 0.000000000000000000, 0.000000000000000000, 1.000000000000000000 ) ) ;
#11590=ADVANCED_FACE ( 'NONE', ( #5759 ), #11474, .T. ) ;
#11591=DIRECTION ( 'NONE',  ( -1.000000000000000000, 1.826024711554534012E-15, 0.000000000000000000 ) ) ;
#11592=DIRECTION ( 'NONE',  ( -0.000000000000000000, -0.000000000000000000, -1.000000000000000000 ) ) ;
#11595=CARTESIAN_POINT ( 'NONE',  ( -13.71740939043329277, 51.19406879332069593, 8.000000000000000000 ) ) ;
#11597=DIRECTION ( 'NONE',  ( -1.000000000000000000, 0.000000000000000000, 0.000000000000000000 ) ) ;
#11598=ORIENTED_EDGE ( 'NONE', *, *, #14241, .T. ) ;
#11599=ORIENTED_EDGE ( 'NONE', *, *, #13168, .T. ) ;
#11601=ORIENTED_EDGE ( 'NONE', *, *, #14273, .F. ) ;
#11604=CARTESIAN_POINT ( 'NONE',  ( 66.70695371924546180, 57.06275842387054098, -13.00000000000000178 ) ) ;
#11605=CARTESIAN_POINT ( 'NONE',  ( 26.49999999999971578, 45.89934640057541060, 8.000000000000000000 ) ) ;
#11607=ORIENTED_EDGE ( 'NONE', *, *, #8696, .T. ) ;
#11608=ORIENTED_EDGE ( 'NONE', *, *, #13027, .T. ) ;
#11609=ORIENTED_EDGE ( 'NONE', *, *, #12757, .T. ) ;
#11610=ADVANCED_FACE ( 'NONE', ( #10542 ), #4779, .F. ) ;
#11611=PLANE ( 'NONE',  #14407 ) ;
#11616=CIRCLE ( 'NONE', #8205, 59.50000000000000000 ) ;
#11619=EDGE_CURVE ( 'NONE', #452, #8824, #13819, .T. ) ;
#11621=CARTESIAN_POINT ( 'NONE',  ( 0.000000000000000000, 0.000000000000000000, -8.000000000000000000 ) ) ;
#11622=CARTESIAN_POINT ( 'NONE',  ( 0.000000000000000000, 0.000000000000000000, -10.50000000000000000 ) ) ;
#11623=CARTESIAN_POINT ( 'NONE',  ( 6.852625091553089298, 52.05085522212500138, -10.50000000000000000 ) ) ;
#11624=DIRECTION ( 'NONE',  ( 0.000000000000000000, 0.000000000000000000, -1.000000000000000000 ) ) ;
#11625=ORIENTED_EDGE ( 'NONE', *, *, #14805, .T. ) ;
#11627=DIRECTION ( 'NONE',  ( 0.000000000000000000, 0.000000000000000000, -1.000000000000000000 ) ) ;
#11628=ORIENTED_EDGE ( 'NONE', *, *, #3061, .F. ) ;
#11629=DIRECTION ( 'NONE',  ( 0.000000000000000000, 0.000000000000000000, -1.000000000000000000 ) ) ;
#11633=DIRECTION ( 'NONE',  ( -1.000000000000000000, 0.000000000000000000, 0.000000000000000000 ) ) ;
#11634=LINE ( 'NONE', #162, #8123 ) ;
#11635=DIRECTION ( 'NONE',  ( 0.000000000000000000, 0.000000000000000000, -1.000000000000000000 ) ) ;
#11641=DIRECTION ( 'NONE',  ( 1.000000000000000000, 0.000000000000000000, 0.000000000000000000 ) ) ;
#11642=ADVANCED_FACE ( 'NONE', ( #11557 ), #1367, .T. ) ;
#11643=ORIENTED_EDGE ( 'NONE', *, *, #3112, .F. ) ;
#11644=DIRECTION ( 'NONE',  ( 1.000000000000000000, 0.000000000000000000, 0.000000000000000000 ) ) ;
#11647=EDGE_CURVE ( 'NONE', #7296, #5870, #4752, .T. ) ;
#11648=AXIS2_PLACEMENT_3D ( 'NONE', #4117, #10949, #8517 ) ;
#11649=DIRECTION ( 'NONE',  ( -1.000000000000000000, 0.000000000000000000, 0.000000000000000000 ) ) ;
#11652=VECTOR ( 'NONE', #5652, 1000.000000000000000 ) ;
#11653=DIRECTION ( 'NONE',  ( 0.000000000000000000, 0.000000000000000000, 1.000000000000000000 ) ) ;
#11656=AXIS2_PLACEMENT_3D ( 'NONE', #12682, #1073, #2195 ) ;
#11658=DIRECTION ( 'NONE',  ( -0.000000000000000000, -0.000000000000000000, 1.000000000000000000 ) ) ;
#11659=CARTESIAN_POINT ( 'NONE',  ( 0.000000000000000000, 0.000000000000000000, -8.000000000000000000 ) ) ;
#11660=CARTESIAN_POINT ( 'NONE',  ( 0.000000000000000000, 0.000000000000000000, 8.000000000000000000 ) ) ;
#11661=CARTESIAN_POINT ( 'NONE',  ( 30.80502811811196295, 49.00442420936003174, -8.000000000000000000 ) ) ;
#11662=EDGE_CURVE ( 'NONE', #1485, #15024, #14412, .T. ) ;
#11664=ORIENTED_EDGE ( 'NONE', *, *, #2686, .F. ) ;
#11665=CARTESIAN_POINT ( 'NONE',  ( 44.13108361037843252, 56.43380494353993271, -8.000000000000000000 ) ) ;
#11666=DIRECTION ( 'NONE',  ( -0.000000000000000000, -0.000000000000000000, 1.000000000000000000 ) ) ;
#11670=VERTEX_POINT ( 'NONE', #12977 ) ;
#11672=VERTEX_POINT ( 'NONE', #3719 ) ;
#11673=AXIS2_PLACEMENT_3D ( 'NONE', #14111, #9611, #9757 ) ;
#11674=ORIENTED_EDGE ( 'NONE', *, *, #9033, .F. ) ;
#11675=DIRECTION ( 'NONE',  ( 0.000000000000000000, 0.000000000000000000, -1.000000000000000000 ) ) ;
#11676=VECTOR ( 'NONE', #11126, 1000.000000000000000 ) ;
#11677=DIRECTION ( 'NONE',  ( 1.000000000000000000, 0.000000000000000000, 0.000000000000000000 ) ) ;
#11679=CARTESIAN_POINT ( 'NONE',  ( -50.00000000000000000, 0.000000000000000000, 13.00000000000000178 ) ) ;
#11680=DIRECTION ( 'NONE',  ( 0.000000000000000000, 0.000000000000000000, 1.000000000000000000 ) ) ;
#11681=CARTESIAN_POINT ( 'NONE',  ( 94.51066581171355097, 1.674280531758986834, 8.000000000000000000 ) ) ;
#11682=ORIENTED_EDGE ( 'NONE', *, *, #1088, .T. ) ;
#11683=ORIENTED_EDGE ( 'NONE', *, *, #1746, .F. ) ;
#11685=CARTESIAN_POINT ( 'NONE',  ( -6.123233995736766085E-15, -100.0000000000000000, -8.000000000000000000 ) ) ;
#11687=EDGE_CURVE ( 'NONE', #11105, #12545, #4714, .T. ) ;
#11688=AXIS2_PLACEMENT_3D ( 'NONE', #5455, #1882, #8635 ) ;
#11689=EDGE_CURVE ( 'NONE', #12431, #2546, #2044, .T. ) ;
#11690=VERTEX_POINT ( 'NONE', #10687 ) ;
#11692=LINE ( 'NONE', #6958, #1366 ) ;
#11693=EDGE_LOOP ( 'NONE', ( #3476, #1837 ) ) ;
#11694=DIRECTION ( 'NONE',  ( 1.000000000000000000, 0.000000000000000000, 0.000000000000000000 ) ) ;
#11697=CIRCLE ( 'NONE', #10955, 0.5000000000000004441 ) ;
#11698=CARTESIAN_POINT ( 'NONE',  ( 37.12029293941315444, -89.61631465359504034, 8.000000000000000000 ) ) ;
#11701=DIRECTION ( 'NONE',  ( 0.000000000000000000, 0.000000000000000000, 1.000000000000000000 ) ) ;
#11704=CARTESIAN_POINT ( 'NONE',  ( 13.71740939043365337, -51.19406879332061067, -13.00000000000000178 ) ) ;
#11706=AXIS2_PLACEMENT_3D ( 'NONE', #12799, #5874, #1044 ) ;
#11708=DIRECTION ( 'NONE',  ( 0.000000000000000000, 0.000000000000000000, 1.000000000000000000 ) ) ;
#11709=CARTESIAN_POINT ( 'NONE',  ( -37.12029293941250074, 89.61631465359532456, -10.50000000000000000 ) ) ;
#11710=CIRCLE ( 'NONE', #11218, 3.000000000000002665 ) ;
#11715=DIRECTION ( 'NONE',  ( 0.000000000000000000, 0.000000000000000000, 1.000000000000000000 ) ) ;
#11716=AXIS2_PLACEMENT_3D ( 'NONE', #8677, #799, #2001 ) ;
#11717=LINE ( 'NONE', #11498, #14113 ) ;
#11718=EDGE_LOOP ( 'NONE', ( #4838, #4021, #1340, #9247, #14912, #7212 ) ) ;
#11719=DIRECTION ( 'NONE',  ( 0.000000000000000000, 0.000000000000000000, -1.000000000000000000 ) ) ;
#11720=CARTESIAN_POINT ( 'NONE',  ( -39.61975340586620575, -91.27544013909724185, 8.000000000000000000 ) ) ;
#11721=AXIS2_PLACEMENT_3D ( 'NONE', #3025, #7646, #9234 ) ;
#11722=LINE ( 'NONE', #4962, #4929 ) ;
#11724=FACE_OUTER_BOUND ( 'NONE', #288, .T. ) ;
#11725=CIRCLE ( 'NONE', #14380, 2.649999999999993694 ) ;
#11726=ORIENTED_EDGE ( 'NONE', *, *, #1891, .F. ) ;
#11727=EDGE_CURVE ( 'NONE', #9073, #13137, #5068, .T. ) ;
#11728=DIRECTION ( 'NONE',  ( 1.000000000000000000, 0.000000000000000000, 0.000000000000000000 ) ) ;
#11729=EDGE_LOOP ( 'NONE', ( #5390, #4892, #3084, #1410, #2131 ) ) ;
#11730=DIRECTION ( 'NONE',  ( 0.000000000000000000, 0.000000000000000000, 1.000000000000000000 ) ) ;
#11731=DIRECTION ( 'NONE',  ( -1.000000000000000000, 0.000000000000000000, 0.000000000000000000 ) ) ;
#11732=AXIS2_PLACEMENT_3D ( 'NONE', #1179, #13943, #1253 ) ;
#11733=DIRECTION ( 'NONE',  ( -0.000000000000000000, -0.000000000000000000, 1.000000000000000000 ) ) ;
#11734=DIRECTION ( 'NONE',  ( 0.000000000000000000, 0.000000000000000000, 1.000000000000000000 ) ) ;
#11736=AXIS2_PLACEMENT_3D ( 'NONE', #4384, #1942, #10138 ) ;
#11737=VERTEX_POINT ( 'NONE', #9760 ) ;
#11738=CARTESIAN_POINT ( 'NONE',  ( -33.48561063518626923, 47.21331623427104063, -13.00000000000000178 ) ) ;
#11739=DIRECTION ( 'NONE',  ( -0.000000000000000000, -0.000000000000000000, 1.000000000000000000 ) ) ;
#11740=CARTESIAN_POINT ( 'NONE',  ( -52.54657765281192638, 6.917888187662934563, 8.000000000000000000 ) ) ;
#11741=CIRCLE ( 'NONE', #5899, 100.0000000000000000 ) ;
#11742=VERTEX_POINT ( 'NONE', #13050 ) ;
#11745=EDGE_CURVE ( 'NONE', #13021, #8628, #841, .T. ) ;
#11746=EDGE_CURVE ( 'NONE', #11672, #14620, #13201, .T. ) ;
#11748=DIRECTION ( 'NONE',  ( 0.000000000000000000, 0.000000000000000000, 1.000000000000000000 ) ) ;
#11749=DIRECTION ( 'NONE',  ( 0.000000000000000000, 0.000000000000000000, 1.000000000000000000 ) ) ;
#11751=CIRCLE ( 'NONE', #3988, 100.0000000000000000 ) ;
#11753=LINE ( 'NONE', #10523, #8138 ) ;
#11757=DIRECTION ( 'NONE',  ( -1.000000000000000000, 0.000000000000000000, 0.000000000000000000 ) ) ;
#11759=CARTESIAN_POINT ( 'NONE',  ( -52.72775723226775568, 7.383907457638128058, -10.50000000000000000 ) ) ;
#11760=VERTEX_POINT ( 'NONE', #3862 ) ;
#11761=AXIS2_PLACEMENT_3D ( 'NONE', #14002, #8213, #11649 ) ;
#11762=ORIENTED_EDGE ( 'NONE', *, *, #5636, .T. ) ;
#11764=AXIS2_PLACEMENT_3D ( 'NONE', #9454, #1646, #6253 ) ;
#11765=AXIS2_PLACEMENT_3D ( 'NONE', #9732, #7229, #1781 ) ;
#11766=VECTOR ( 'NONE', #11009, 1000.000000000000000 ) ;
#11768=CARTESIAN_POINT ( 'NONE',  ( 56.43380494353997534, 12.86891638962136319, -8.000000000000000000 ) ) ;
#11769=CARTESIAN_POINT ( 'NONE',  ( 68.58935777509475429, -68.58935777509547904, 8.000000000000000000 ) ) ;
#11771=CARTESIAN_POINT ( 'NONE',  ( 37.12029293941379393, 89.61631465359479876, -13.00000000000000178 ) ) ;
#11772=DIRECTION ( 'NONE',  ( 1.000000000000000000, 0.000000000000000000, 0.000000000000000000 ) ) ;
#11780=ORIENTED_EDGE ( 'NONE', *, *, #8742, .T. ) ;
#11781=DIRECTION ( 'NONE',  ( 1.000000000000000000, 0.000000000000000000, 0.000000000000000000 ) ) ;
#11783=AXIS2_PLACEMENT_3D ( 'NONE', #9771, #13283, #2877 ) ;
#11785=ORIENTED_EDGE ( 'NONE', *, *, #9533, .T. ) ;
#11788=ADVANCED_FACE ( 'NONE', ( #907 ), #2943, .F. ) ;
#11794=DIRECTION ( 'NONE',  ( -1.000000000000000000, 0.000000000000000000, 0.000000000000000000 ) ) ;
#11795=VECTOR ( 'NONE', #9317, 1000.000000000000000 ) ;
#11797=ADVANCED_FACE ( 'NONE', ( #8924 ), #5525, .T. ) ;
#11798=FACE_OUTER_BOUND ( 'NONE', #224, .T. ) ;
#11799=DIRECTION ( 'NONE',  ( -1.000000000000000000, 0.000000000000000000, 0.000000000000000000 ) ) ;
#11800=DIRECTION ( 'NONE',  ( 1.000000000000000000, 2.664535259100375697E-15, 0.000000000000000000 ) ) ;
#11802=ORIENTED_EDGE ( 'NONE', *, *, #9856, .T. ) ;
#11803=AXIS2_PLACEMENT_3D ( 'NONE', #12797, #2382, #9068 ) ;
#11804=FACE_OUTER_BOUND ( 'NONE', #2636, .T. ) ;
#11805=ORIENTED_EDGE ( 'NONE', *, *, #14627, .T. ) ;
#11807=DIRECTION ( 'NONE',  ( 1.000000000000000000, 0.000000000000000000, 0.000000000000000000 ) ) ;
#11808=CARTESIAN_POINT ( 'NONE',  ( 0.000000000000000000, 0.000000000000000000, -8.000000000000000000 ) ) ;
#11809=CARTESIAN_POINT ( 'NONE',  ( 30.43807145043611584, -39.66766701456170097, 8.000000000000000000 ) ) ;
#11810=CARTESIAN_POINT ( 'NONE',  ( -37.12029293941441210, -89.61631465359452875, 8.000000000000000000 ) ) ;
#11812=ORIENTED_EDGE ( 'NONE', *, *, #9362, .F. ) ;
#11813=CIRCLE ( 'NONE', #904, 50.00000000000000000 ) ;
#11814=CYLINDRICAL_SURFACE ( 'NONE', #3795, 59.50000000000000000 ) ;
#11815=CARTESIAN_POINT ( 'NONE',  ( 0.000000000000000000, 0.000000000000000000, -10.50000000000000000 ) ) ;
#11816=DIRECTION ( 'NONE',  ( 1.000000000000000000, -4.440892098500626162E-15, 0.000000000000000000 ) ) ;
#11817=VERTEX_POINT ( 'NONE', #9999 ) ;
#11818=ORIENTED_EDGE ( 'NONE', *, *, #12369, .F. ) ;
#11820=CARTESIAN_POINT ( 'NONE',  ( -45.89934640057513349, 26.50000000000019540, -13.00000000000000178 ) ) ;
#11821=CARTESIAN_POINT ( 'NONE',  ( 68.58935777509523746, 68.58935777509499587, -8.000000000000000000 ) ) ;
#11823=DIRECTION ( 'NONE',  ( 0.000000000000000000, 0.000000000000000000, 1.000000000000000000 ) ) ;
#11824=ADVANCED_FACE ( 'NONE', ( #1953 ), #13496, .F. ) ;
#11827=EDGE_CURVE ( 'NONE', #12492, #1887, #10525, .T. ) ;
#11829=EDGE_CURVE ( 'NONE', #7998, #13011, #5912, .T. ) ;
#11830=DIRECTION ( 'NONE',  ( 0.000000000000000000, 0.000000000000000000, 1.000000000000000000 ) ) ;
#11831=LINE ( 'NONE', #3707, #934 ) ;
#11832=LINE ( 'NONE', #14321, #12458 ) ;
#11833=ADVANCED_FACE ( 'NONE', ( #9005 ), #13647, .F. ) ;
#11835=ORIENTED_EDGE ( 'NONE', *, *, #12941, .T. ) ;
#11836=ORIENTED_EDGE ( 'NONE', *, *, #5512, .F. ) ;
#11837=DIRECTION ( 'NONE',  ( -1.000000000000000000, 0.000000000000000000, 0.000000000000000000 ) ) ;
#11838=VERTEX_POINT ( 'NONE', #6719 ) ;
#11840=LINE ( 'NONE', #6397, #533 ) ;
#11841=CARTESIAN_POINT ( 'NONE',  ( 6.917888187663118416, 52.54657765281190507, -8.000000000000000000 ) ) ;
#11842=ADVANCED_FACE ( 'NONE', ( #13561 ), #6570, .F. ) ;
#11845=CIRCLE ( 'NONE', #13786, 3.000000000000002665 ) ;
#11849=FACE_OUTER_BOUND ( 'NONE', #10887, .T. ) ;
#11850=ORIENTED_EDGE ( 'NONE', *, *, #9865, .T. ) ;
#11851=ORIENTED_EDGE ( 'NONE', *, *, #10063, .T. ) ;
#11854=DIRECTION ( 'NONE',  ( 0.000000000000000000, 0.000000000000000000, -1.000000000000000000 ) ) ;
#11856=CARTESIAN_POINT ( 'NONE',  ( -89.61631465359519666, -37.12029293941281338, -13.00000000000000178 ) ) ;
#11857=DIRECTION ( 'NONE',  ( 0.000000000000000000, 0.000000000000000000, -1.000000000000000000 ) ) ;
#11858=DIRECTION ( 'NONE',  ( -0.000000000000000000, -0.000000000000000000, -1.000000000000000000 ) ) ;
#11860=ORIENTED_EDGE ( 'NONE', *, *, #14225, .F. ) ;
#11861=DIRECTION ( 'NONE',  ( 0.000000000000000000, 0.000000000000000000, 1.000000000000000000 ) ) ;
#11866=EDGE_CURVE ( 'NONE', #13570, #10850, #4247, .T. ) ;
#11867=EDGE_CURVE ( 'NONE', #8628, #14193, #8860, .T. ) ;
#11868=CARTESIAN_POINT ( 'NONE',  ( 68.68541276968825571, -69.08004447556089644, 10.49999999999999822 ) ) ;
#11873=VERTEX_POINT ( 'NONE', #10078 ) ;
#11874=FACE_OUTER_BOUND ( 'NONE', #1127, .T. ) ;
#11875=FACE_OUTER_BOUND ( 'NONE', #5360, .T. ) ;
#11876=EDGE_CURVE ( 'NONE', #1886, #5824, #4212, .T. ) ;
#11877=CIRCLE ( 'NONE', #2409, 2.649999999999987477 ) ;
#11879=DIRECTION ( 'NONE',  ( 1.000000000000000000, 0.000000000000000000, 0.000000000000000000 ) ) ;
#11881=ORIENTED_EDGE ( 'NONE', *, *, #3367, .F. ) ;
#11882=VERTEX_POINT ( 'NONE', #14723 ) ;
#11883=FACE_OUTER_BOUND ( 'NONE', #5232, .T. ) ;
#11884=CARTESIAN_POINT ( 'NONE',  ( 2.449293598294700991E-16, -97.00000000000000000, 8.000000000000000000 ) ) ;
#11886=EDGE_CURVE ( 'NONE', #6680, #3464, #5651, .T. ) ;
#11887=CARTESIAN_POINT ( 'NONE',  ( 66.70695371924546180, 57.06275842387054098, -8.000000000000000000 ) ) ;
#11888=CIRCLE ( 'NONE', #8239, 59.50000000000000711 ) ;
#11889=CIRCLE ( 'NONE', #735, 0.5000000000000004441 ) ;
#11890=AXIS2_PLACEMENT_3D ( 'NONE', #7131, #10711, #3657 ) ;
#11891=ORIENTED_EDGE ( 'NONE', *, *, #5175, .F. ) ;
#11892=ORIENTED_EDGE ( 'NONE', *, *, #3818, .T. ) ;
#11893=FACE_OUTER_BOUND ( 'NONE', #9986, .T. ) ;
#11895=AXIS2_PLACEMENT_3D ( 'NONE', #9953, #3063, #3282 ) ;
#11896=CARTESIAN_POINT ( 'NONE',  ( -7.383907457637922889, -52.72775723226778410, -10.50000000000000000 ) ) ;
#11897=CARTESIAN_POINT ( 'NONE',  ( 14.70911110638339814, -51.49712671369398720, -10.50000000000000000 ) ) ;
#11899=DIRECTION ( 'NONE',  ( 0.000000000000000000, 0.000000000000000000, 1.000000000000000000 ) ) ;
#11900=VECTOR ( 'NONE', #312, 1000.000000000000000 ) ;
#11901=ORIENTED_EDGE ( 'NONE', *, *, #12247, .F. ) ;
#11903=ORIENTED_EDGE ( 'NONE', *, *, #9716, .F. ) ;
#11904=VECTOR ( 'NONE', #7258, 1000.000000000000000 ) ;
#11905=EDGE_LOOP ( 'NONE', ( #7490, #6485, #11201, #4476 ) ) ;
#11907=DIRECTION ( 'NONE',  ( 0.000000000000000000, 0.000000000000000000, 1.000000000000000000 ) ) ;
#11908=DIRECTION ( 'NONE',  ( 0.000000000000000000, 0.000000000000000000, -1.000000000000000000 ) ) ;
#11910=ORIENTED_EDGE ( 'NONE', *, *, #5136, .T. ) ;
#11911=AXIS2_PLACEMENT_3D ( 'NONE', #8435, #11861, #10792 ) ;
#11912=AXIS2_PLACEMENT_3D ( 'NONE', #10156, #5468, #4261 ) ;
#11913=ORIENTED_EDGE ( 'NONE', *, *, #451, .F. ) ;
#11914=CARTESIAN_POINT ( 'NONE',  ( -32.06294366074467206, 42.50536573064442081, -10.50000000000000000 ) ) ;
#11915=AXIS2_PLACEMENT_3D ( 'NONE', #390, #7206, #10931 ) ;
#11916=ORIENTED_EDGE ( 'NONE', *, *, #11094, .F. ) ;
#11917=AXIS2_PLACEMENT_3D ( 'NONE', #14466, #9594, #652 ) ;
#11918=EDGE_CURVE ( 'NONE', #14678, #6775, #12209, .T. ) ;
#11921=DIRECTION ( 'NONE',  ( -1.000000000000000000, 0.000000000000000000, 0.000000000000000000 ) ) ;
#11922=DIRECTION ( 'NONE',  ( 0.000000000000000000, 0.000000000000000000, 1.000000000000000000 ) ) ;
#11923=AXIS2_PLACEMENT_3D ( 'NONE', #3398, #8023, #2110 ) ;
#11924=DIRECTION ( 'NONE',  ( 0.000000000000000000, 0.000000000000000000, 1.000000000000000000 ) ) ;
#11925=ORIENTED_EDGE ( 'NONE', *, *, #1460, .F. ) ;
#11926=AXIS2_PLACEMENT_3D ( 'NONE', #2029, #6647, #4392 ) ;
#11927=CARTESIAN_POINT ( 'NONE',  ( -33.48561063518626923, 47.21331623427104063, 8.000000000000000000 ) ) ;
#11928=AXIS2_PLACEMENT_3D ( 'NONE', #1244, #1400, #11728 ) ;
#11929=ORIENTED_EDGE ( 'NONE', *, *, #8325, .T. ) ;
#11933=CIRCLE ( 'NONE', #6089, 3.000000000000002665 ) ;
#11935=ORIENTED_EDGE ( 'NONE', *, *, #13230, .T. ) ;
#11936=ADVANCED_FACE ( 'NONE', ( #4543 ), #7941, .F. ) ;
#11937=EDGE_CURVE ( 'NONE', #14224, #9901, #11489, .T. ) ;
#11938=DIRECTION ( 'NONE',  ( 0.000000000000000000, 0.000000000000000000, -1.000000000000000000 ) ) ;
#11941=DIRECTION ( 'NONE',  ( 1.000000000000000000, 0.000000000000000000, 0.000000000000000000 ) ) ;
#11944=ORIENTED_EDGE ( 'NONE', *, *, #11370, .T. ) ;
#11950=CIRCLE ( 'NONE', #10481, 0.5000000000000004441 ) ;
#11951=CARTESIAN_POINT ( 'NONE',  ( 0.000000000000000000, 0.000000000000000000, 8.000000000000000000 ) ) ;
#11952=CARTESIAN_POINT ( 'NONE',  ( -50.00000000000000000, 0.000000000000000000, -13.00000000000000178 ) ) ;
#11953=ORIENTED_EDGE ( 'NONE', *, *, #1585, .T. ) ;
#11956=AXIS2_PLACEMENT_3D ( 'NONE', #8532, #187, #13175 ) ;
#11958=CARTESIAN_POINT ( 'NONE',  ( 44.89637028918152595, -6.028507236160502272E-15, -25.50000000000000355 ) ) ;
#11960=EDGE_CURVE ( 'NONE', #8252, #14878, #6353, .T. ) ;
#11961=CIRCLE ( 'NONE', #10912, 50.00000000000000000 ) ;
#11965=DIRECTION ( 'NONE',  ( 1.000000000000000000, 0.000000000000000000, 0.000000000000000000 ) ) ;
#11966=DIRECTION ( 'NONE',  ( 0.000000000000000000, 0.000000000000000000, 1.000000000000000000 ) ) ;
#11967=AXIS2_PLACEMENT_3D ( 'NONE', #9279, #19, #4581 ) ;
#11970=AXIS2_PLACEMENT_3D ( 'NONE', #4517, #11584, #1170 ) ;
#11971=ORIENTED_EDGE ( 'NONE', *, *, #8463, .T. ) ;
#11972=CARTESIAN_POINT ( 'NONE',  ( 0.000000000000000000, 0.000000000000000000, -25.50000000000000355 ) ) ;
#11973=VECTOR ( 'NONE', #193, 1000.000000000000000 ) ;
#11975=CARTESIAN_POINT ( 'NONE',  ( -37.12029293941441210, -89.61631465359452875, -13.00000000000000178 ) ) ;
#11976=VERTEX_POINT ( 'NONE', #8170 ) ;
#11978=AXIS2_PLACEMENT_3D ( 'NONE', #287, #9836, #8470 ) ;
#11979=CARTESIAN_POINT ( 'NONE',  ( 0.000000000000000000, 0.000000000000000000, -10.50000000000000000 ) ) ;
#11980=EDGE_CURVE ( 'NONE', #8921, #9550, #3955, .T. ) ;
#11984=VERTEX_POINT ( 'NONE', #11679 ) ;
#11985=ORIENTED_EDGE ( 'NONE', *, *, #13646, .F. ) ;
#11986=ORIENTED_EDGE ( 'NONE', *, *, #1529, .T. ) ;
#11987=CARTESIAN_POINT ( 'NONE',  ( 51.53979475227119167, 13.35619814848851483, -10.50000000000000000 ) ) ;
#11988=CARTESIAN_POINT ( 'NONE',  ( -42.04772703543551415, -32.26435573746212526, -8.000000000000000000 ) ) ;
#11989=CIRCLE ( 'NONE', #10996, 0.5000000000000022204 ) ;
#11991=VERTEX_POINT ( 'NONE', #2256 ) ;
#11992=ORIENTED_EDGE ( 'NONE', *, *, #7066, .F. ) ;
#11993=PLANE ( 'NONE',  #8117 ) ;
#11994=VERTEX_POINT ( 'NONE', #13883 ) ;
#11995=CIRCLE ( 'NONE', #12950, 53.55662432702593634 ) ;
#11998=CIRCLE ( 'NONE', #2045, 50.00000000000000000 ) ;
#12000=DIRECTION ( 'NONE',  ( -0.000000000000000000, -0.000000000000000000, 1.000000000000000000 ) ) ;
#12001=ORIENTED_EDGE ( 'NONE', *, *, #3098, .T. ) ;
#12002=CARTESIAN_POINT ( 'NONE',  ( 6.451868917687939131, 52.36539807335604024, 10.49999999999999822 ) ) ;
#12003=DIRECTION ( 'NONE',  ( 0.000000000000000000, 0.000000000000000000, -1.000000000000000000 ) ) ;
#12004=ORIENTED_EDGE ( 'NONE', *, *, #10261, .F. ) ;
#12005=CARTESIAN_POINT ( 'NONE',  ( -100.0000000000000000, 0.000000000000000000, -13.00000000000000178 ) ) ;
#12006=AXIS2_PLACEMENT_3D ( 'NONE', #8468, #9905, #5216 ) ;
#12007=ORIENTED_EDGE ( 'NONE', *, *, #12524, .T. ) ;
#12010=DIRECTION ( 'NONE',  ( 0.000000000000000000, 0.000000000000000000, 1.000000000000000000 ) ) ;
#12011=DIRECTION ( 'NONE',  ( 1.000000000000000000, 0.000000000000000000, -0.000000000000000000 ) ) ;
#12012=AXIS2_PLACEMENT_3D ( 'NONE', #9605, #6326, #9749 ) ;
#12013=DIRECTION ( 'NONE',  ( 1.000000000000000000, 0.000000000000000000, 0.000000000000000000 ) ) ;
#12014=CARTESIAN_POINT ( 'NONE',  ( 94.51066581171355097, 1.674280531758986834, -13.00000000000000178 ) ) ;
#12015=DIRECTION ( 'NONE',  ( -1.000000000000000000, 0.000000000000000000, 0.000000000000000000 ) ) ;
#12016=CIRCLE ( 'NONE', #11030, 0.5000000000000073275 ) ;
#12021=ORIENTED_EDGE ( 'NONE', *, *, #4887, .T. ) ;
#12023=EDGE_CURVE ( 'NONE', #10391, #215, #14143, .T. ) ;
#12025=CARTESIAN_POINT ( 'NONE',  ( 49.00442420935993226, -30.80502811811213704, -8.000000000000000000 ) ) ;
#12027=MECHANICAL_DESIGN_GEOMETRIC_PRESENTATION_REPRESENTATION('',(#117),#13709);
#12028=CARTESIAN_POINT ( 'NONE',  ( 12.86891638962116247, -56.43380494354001087, -10.50000000000000000 ) ) ;
#12029=CIRCLE ( 'NONE', #8611, 50.00000000000000000 ) ;
#12030=DIRECTION ( 'NONE',  ( 0.000000000000000000, 0.000000000000000000, 1.000000000000000000 ) ) ;
#12031=ORIENTED_EDGE ( 'NONE', *, *, #12616, .T. ) ;
#12032=DIRECTION ( 'NONE',  ( -0.000000000000000000, -0.000000000000000000, -1.000000000000000000 ) ) ;
#12033=ORIENTED_EDGE ( 'NONE', *, *, #6929, .T. ) ;
#12034=ORIENTED_EDGE ( 'NONE', *, *, #42, .F. ) ;
#12035=CARTESIAN_POINT ( 'NONE',  ( -14.70911110638303754, 51.49712671369408667, -10.50000000000000000 ) ) ;
#12036=DIRECTION ( 'NONE',  ( 1.000000000000000000, 8.746504920891464822E-16, 0.000000000000000000 ) ) ;
#12037=AXIS2_PLACEMENT_3D ( 'NONE', #582, #5285, #5215 ) ;
#12038=AXIS2_PLACEMENT_3D ( 'NONE', #14801, #11385, #3406 ) ;
#12039=DIRECTION ( 'NONE',  ( -1.000000000000000000, 0.000000000000000000, 0.000000000000000000 ) ) ;
#12040=CYLINDRICAL_SURFACE ( 'NONE', #10505, 59.50000000000000000 ) ;
#12041=DIRECTION ( 'NONE',  ( -1.000000000000000000, 0.000000000000000000, 0.000000000000000000 ) ) ;
#12042=VERTEX_POINT ( 'NONE', #11454 ) ;
#12043=DIRECTION ( 'NONE',  ( 1.000000000000000000, 0.000000000000000000, 0.000000000000000000 ) ) ;
#12044=DIRECTION ( 'NONE',  ( 0.000000000000000000, 0.000000000000000000, 1.000000000000000000 ) ) ;
#12046=CIRCLE ( 'NONE', #1845, 0.5000000000000004441 ) ;
#12048=EDGE_LOOP ( 'NONE', ( #11903, #8010, #9451, #2347 ) ) ;
#12049=DIRECTION ( 'NONE',  ( 0.000000000000000000, 0.000000000000000000, 1.000000000000000000 ) ) ;
#12050=VERTEX_POINT ( 'NONE', #12739 ) ;
#12051=LINE ( 'NONE', #7541, #9796 ) ;
#12052=VERTEX_POINT ( 'NONE', #10447 ) ;
#12053=DIRECTION ( 'NONE',  ( 1.000000000000000000, 0.000000000000000000, -0.000000000000000000 ) ) ;
#12054=CARTESIAN_POINT ( 'NONE',  ( 24.98583958711424202, -30.74264578624780597, -25.50000000000000355 ) ) ;
#12055=LINE ( 'NONE', #10826, #2082 ) ;
#12058=DIRECTION ( 'NONE',  ( 1.000000000000000000, 0.000000000000000000, 0.000000000000000000 ) ) ;
#12060=ORIENTED_EDGE ( 'NONE', *, *, #7670, .T. ) ;
#12062=EDGE_CURVE ( 'NONE', #13092, #14329, #9598, .T. ) ;
#12063=EDGE_LOOP ( 'NONE', ( #5202, #8403, #8434, #12829, #8535, #1363 ) ) ;
#12065=ORIENTED_EDGE ( 'NONE', *, *, #3434, .F. ) ;
#12066=CARTESIAN_POINT ( 'NONE',  ( -37.71449950290985953, 86.67575032682117353, -8.000000000000000000 ) ) ;
#12069=LINE ( 'NONE', #1660, #1241 ) ;
#12070=CARTESIAN_POINT ( 'NONE',  ( -3.492805317593278058, 46.55633131742322917, -10.50000000000000000 ) ) ;
#12071=ORIENTED_EDGE ( 'NONE', *, *, #2597, .F. ) ;
#12072=DIRECTION ( 'NONE',  ( 0.000000000000000000, 0.000000000000000000, 1.000000000000000000 ) ) ;
#12073=VECTOR ( 'NONE', #13292, 1000.000000000000000 ) ;
#12075=EDGE_CURVE ( 'NONE', #9694, #1381, #3925, .T. ) ;
#12077=DIRECTION ( 'NONE',  ( 0.000000000000000000, 0.000000000000000000, -1.000000000000000000 ) ) ;
#12080=CIRCLE ( 'NONE', #5531, 59.50000000000000000 ) ;
#12083=DIRECTION ( 'NONE',  ( -1.000000000000000000, 0.000000000000000000, 0.000000000000000000 ) ) ;
#12085=ORIENTED_EDGE ( 'NONE', *, *, #1001, .T. ) ;
#12088=ORIENTED_EDGE ( 'NONE', *, *, #7731, .F. ) ;
#12089=CARTESIAN_POINT ( 'NONE',  ( -51.53979475227126983, -13.35619814848815601, -10.50000000000000000 ) ) ;
#12090=DIRECTION ( 'NONE',  ( -1.000000000000000000, 0.000000000000000000, 0.000000000000000000 ) ) ;
#12091=ORIENTED_EDGE ( 'NONE', *, *, #9779, .F. ) ;
#12092=DIRECTION ( 'NONE',  ( -0.000000000000000000, -0.000000000000000000, 1.000000000000000000 ) ) ;
#12095=PLANE ( 'NONE',  #2897 ) ;
#12096=ORIENTED_EDGE ( 'NONE', *, *, #6698, .F. ) ;
#12098=EDGE_CURVE ( 'NONE', #11105, #13418, #5163, .T. ) ;
#12099=CARTESIAN_POINT ( 'NONE',  ( 0.000000000000000000, 0.000000000000000000, 8.000000000000000000 ) ) ;
#12102=DIRECTION ( 'NONE',  ( 0.000000000000000000, 0.000000000000000000, -1.000000000000000000 ) ) ;
#12103=CARTESIAN_POINT ( 'NONE',  ( 68.49330278050122445, -68.09867107463004743, -10.50000000000000000 ) ) ;
#12106=CARTESIAN_POINT ( 'NONE',  ( -47.21331623427138879, -33.48561063518577896, -13.00000000000000178 ) ) ;
#12107=DIRECTION ( 'NONE',  ( 0.000000000000000000, 0.000000000000000000, 1.000000000000000000 ) ) ;
#12109=ORIENTED_EDGE ( 'NONE', *, *, #6844, .T. ) ;
#12113=DIRECTION ( 'NONE',  ( 1.000000000000000000, 0.000000000000000000, 0.000000000000000000 ) ) ;
#12114=EDGE_CURVE ( 'NONE', #1055, #1207, #1778, .T. ) ;
#12121=ORIENTED_EDGE ( 'NONE', *, *, #6369, .F. ) ;
#12123=CIRCLE ( 'NONE', #8951, 3.000000000000002665 ) ;
#12124=CARTESIAN_POINT ( 'NONE',  ( 33.48561063518626923, -47.21331623427104063, -13.00000000000000178 ) ) ;
#12126=CARTESIAN_POINT ( 'NONE',  ( -37.12029293941441210, -89.61631465359452875, -8.000000000000000000 ) ) ;
#12129=DIRECTION ( 'NONE',  ( 1.000000000000000000, 0.000000000000000000, -0.000000000000000000 ) ) ;
#12131=ORIENTED_EDGE ( 'NONE', *, *, #1376, .F. ) ;
#12134=DIRECTION ( 'NONE',  ( 1.000000000000000000, 0.000000000000000000, 0.000000000000000000 ) ) ;
#12136=AXIS2_PLACEMENT_3D ( 'NONE', #12920, #1450, #1605 ) ;
#12138=EDGE_CURVE ( 'NONE', #9656, #5604, #7085, .T. ) ;
#12139=FACE_OUTER_BOUND ( 'NONE', #8064, .T. ) ;
#12140=DIRECTION ( 'NONE',  ( -0.000000000000000000, -0.000000000000000000, -1.000000000000000000 ) ) ;
#12141=EDGE_CURVE ( 'NONE', #6102, #13227, #1061, .T. ) ;
#12142=ORIENTED_EDGE ( 'NONE', *, *, #10239, .F. ) ;
#12143=CARTESIAN_POINT ( 'NONE',  ( -33.48561063518626923, 47.21331623427104063, -13.00000000000000178 ) ) ;
#12145=VERTEX_POINT ( 'NONE', #4991 ) ;
#12146=AXIS2_PLACEMENT_3D ( 'NONE', #6835, #9120, #1161 ) ;
#12147=AXIS2_PLACEMENT_3D ( 'NONE', #4342, #13675, #5479 ) ;
#12149=DIRECTION ( 'NONE',  ( 1.000000000000000000, 0.000000000000000000, 0.000000000000000000 ) ) ;
#12153=CIRCLE ( 'NONE', #11176, 50.00000000000000000 ) ;
#12154=DIRECTION ( 'NONE',  ( 0.000000000000000000, 0.000000000000000000, -1.000000000000000000 ) ) ;
#12155=LINE ( 'NONE', #2255, #5835 ) ;
#12156=FACE_OUTER_BOUND ( 'NONE', #8779, .T. ) ;
#12157=CARTESIAN_POINT ( 'NONE',  ( -3.492805317593278058, 46.55633131742322917, -10.50000000000000000 ) ) ;
#12159=AXIS2_PLACEMENT_3D ( 'NONE', #677, #6426, #5298 ) ;
#12161=CARTESIAN_POINT ( 'NONE',  ( -45.83364790889027773, 29.49928053175948506, -13.00000000000000178 ) ) ;
#12164=CARTESIAN_POINT ( 'NONE',  ( -49.57224306869049713, 6.526309611002767852, 8.000000000000000000 ) ) ;
#12165=DIRECTION ( 'NONE',  ( -1.000000000000000000, 0.000000000000000000, 0.000000000000000000 ) ) ;
#12166=VERTEX_POINT ( 'NONE', #7237 ) ;
#12169=ORIENTED_EDGE ( 'NONE', *, *, #7672, .T. ) ;
#12170=DIRECTION ( 'NONE',  ( 0.000000000000000000, 0.000000000000000000, 1.000000000000000000 ) ) ;
#12171=VERTEX_POINT ( 'NONE', #12054 ) ;
#12172=DIRECTION ( 'NONE',  ( 0.000000000000000000, 0.000000000000000000, 1.000000000000000000 ) ) ;
#12173=DIRECTION ( 'NONE',  ( -1.000000000000000000, 0.000000000000000000, 0.000000000000000000 ) ) ;
#12174=DIRECTION ( 'NONE',  ( 0.000000000000000000, 0.000000000000000000, 1.000000000000000000 ) ) ;
#12175=AXIS2_PLACEMENT_3D ( 'NONE', #3661, #8139, #8285 ) ;
#12177=DIRECTION ( 'NONE',  ( 0.000000000000000000, 0.000000000000000000, -1.000000000000000000 ) ) ;
#12178=CYLINDRICAL_SURFACE ( 'NONE', #1980, 60.50000000000000711 ) ;
#12179=VERTEX_POINT ( 'NONE', #14095 ) ;
#12180=AXIS2_PLACEMENT_3D ( 'NONE', #13402, #14771, #5277 ) ;
#12181=DIRECTION ( 'NONE',  ( 0.000000000000000000, 0.000000000000000000, 1.000000000000000000 ) ) ;
#12182=DIRECTION ( 'NONE',  ( 0.000000000000000000, 0.000000000000000000, 1.000000000000000000 ) ) ;
#12183=UNCERTAINTY_MEASURE_WITH_UNIT (LENGTH_MEASURE( 1.000000000000000082E-05 ), #14644, 'distance_accuracy_value', 'NONE');
#12184=FACE_OUTER_BOUND ( 'NONE', #10280, .T. ) ;
#12186=ORIENTED_EDGE ( 'NONE', *, *, #13127, .T. ) ;
#12188=DIRECTION ( 'NONE',  ( 1.000000000000000000, 0.000000000000000000, 0.000000000000000000 ) ) ;
#12189=ORIENTED_EDGE ( 'NONE', *, *, #3480, .F. ) ;
#12195=CARTESIAN_POINT ( 'NONE',  ( 23.50071946824040836, 45.96504489226015977, -13.00000000000000178 ) ) ;
#12197=VERTEX_POINT ( 'NONE', #11897 ) ;
#12198=CIRCLE ( 'NONE', #7080, 52.50000000000000711 ) ;
#12199=ORIENTED_EDGE ( 'NONE', *, *, #2303, .F. ) ;
#12201=CYLINDRICAL_SURFACE ( 'NONE', #3053, 63.00000000000000000 ) ;
#12202=CARTESIAN_POINT ( 'NONE',  ( 0.000000000000000000, 0.000000000000000000, 8.000000000000000000 ) ) ;
#12203=AXIS2_PLACEMENT_3D ( 'NONE', #10636, #9496, #324 ) ;
#12204=ADVANCED_FACE ( 'NONE', ( #2555 ), #7170, .F. ) ;
#12206=EDGE_CURVE ( 'NONE', #1924, #6323, #2267, .T. ) ;
#12207=EDGE_CURVE ( 'NONE', #1787, #13337, #8913, .T. ) ;
#12208=ORIENTED_EDGE ( 'NONE', *, *, #14050, .F. ) ;
#12209=CIRCLE ( 'NONE', #11721, 53.55662432702593634 ) ;
#12210=EDGE_LOOP ( 'NONE', ( #8011, #15017, #14071, #14782 ) ) ;
#12211=ORIENTED_EDGE ( 'NONE', *, *, #9033, .T. ) ;
#12213=DIRECTION ( 'NONE',  ( -0.000000000000000000, -0.000000000000000000, -1.000000000000000000 ) ) ;
#12215=AXIS2_PLACEMENT_3D ( 'NONE', #1715, #6320, #14705 ) ;
#12216=PLANE ( 'NONE',  #12159 ) ;
#12217=DIRECTION ( 'NONE',  ( -1.000000000000000000, 0.000000000000000000, 0.000000000000000000 ) ) ;
#12218=EDGE_LOOP ( 'NONE', ( #5094, #9260, #381, #4134, #130, #7261 ) ) ;
#12220=ORIENTED_EDGE ( 'NONE', *, *, #8246, .F. ) ;
#12222=ORIENTED_EDGE ( 'NONE', *, *, #2649, .F. ) ;
#12224=CIRCLE ( 'NONE', #4234, 0.5000000000000004441 ) ;
#12226=EDGE_CURVE ( 'NONE', #132, #9892, #9286, .T. ) ;
#12227=DIRECTION ( 'NONE',  ( 1.000000000000000000, 0.000000000000000000, 0.000000000000000000 ) ) ;
#12229=DIRECTION ( 'NONE',  ( 1.000000000000000000, 0.000000000000000000, 0.000000000000000000 ) ) ;
#12230=DIRECTION ( 'NONE',  ( 1.000000000000000000, 0.000000000000000000, 0.000000000000000000 ) ) ;
#12231=CARTESIAN_POINT ( 'NONE',  ( -2.649999999999994138, 38.00000000000000000, -28.00000000000000000 ) ) ;
#12233=ORIENTED_EDGE ( 'NONE', *, *, #1707, .F. ) ;
#12235=AXIS2_PLACEMENT_3D ( 'NONE', #6059, #12996, #7124 ) ;
#12237=DIRECTION ( 'NONE',  ( 1.000000000000000000, 0.000000000000000000, 0.000000000000000000 ) ) ;
#12238=AXIS2_PLACEMENT_3D ( 'NONE', #4318, #4389, #12134 ) ;
#12240=CARTESIAN_POINT ( 'NONE',  ( 51.19406879332056093, 13.71740939043382745, -8.000000000000000000 ) ) ;
#12242=SURFACE_STYLE_FILL_AREA ( #13296 ) ;
#12245=CIRCLE ( 'NONE', #12968, 63.00000000000000000 ) ;
#12246=FACE_BOUND ( 'NONE', #5029, .T. ) ;
#12247=EDGE_CURVE ( 'NONE', #1887, #9608, #2748, .T. ) ;
#12250=CIRCLE ( 'NONE', #11764, 3.000000000000002665 ) ;
#12251=DIRECTION ( 'NONE',  ( 1.000000000000000000, 0.000000000000000000, -0.000000000000000000 ) ) ;
#12252=AXIS2_PLACEMENT_3D ( 'NONE', #7497, #14501, #4033 ) ;
#12253=ORIENTED_EDGE ( 'NONE', *, *, #4587, .F. ) ;
#12254=CYLINDRICAL_SURFACE ( 'NONE', #1323, 3.000000000000002665 ) ;
#12256=DIRECTION ( 'NONE',  ( 0.000000000000000000, 0.000000000000000000, 1.000000000000000000 ) ) ;
#12257=CARTESIAN_POINT ( 'NONE',  ( 65.64523757230274725, 68.01302780753375998, 8.000000000000000000 ) ) ;
#12258=DIRECTION ( 'NONE',  ( 0.000000000000000000, 0.000000000000000000, 1.000000000000000000 ) ) ;
#12259=EDGE_CURVE ( 'NONE', #13104, #4116, #4305, .T. ) ;
#12260=ORIENTED_EDGE ( 'NONE', *, *, #10659, .T. ) ;
#12262=COLOUR_RGB ( '', 0.09019608, 0.27058824, 0.51372549) ;
#12263=VERTEX_POINT ( 'NONE', #14474 ) ;
#12264=CARTESIAN_POINT ( 'NONE',  ( 91.27544013909738396, -39.61975340586587890, 8.000000000000000000 ) ) ;
#12265=DIRECTION ( 'NONE',  ( 1.000000000000000000, 0.000000000000000000, 0.000000000000000000 ) ) ;
#12266=CIRCLE ( 'NONE', #10560, 3.000000000000002665 ) ;
#12267=LINE ( 'NONE', #5425, #10737 ) ;
#12268=EDGE_CURVE ( 'NONE', #11078, #8551, #8548, .T. ) ;
#12269=EDGE_LOOP ( 'NONE', ( #11350, #5388, #8640, #11682, #2630 ) ) ;
#12271=VECTOR ( 'NONE', #11156, 1000.000000000000000 ) ;
#12273=DIRECTION ( 'NONE',  ( 1.000000000000000000, 0.000000000000000000, 0.000000000000000000 ) ) ;
#12275=ORIENTED_EDGE ( 'NONE', *, *, #13726, .T. ) ;
#12276=CARTESIAN_POINT ( 'NONE',  ( 32.06294366074496338, -42.50536573064421475, -13.00000000000000178 ) ) ;
#12277=DIRECTION ( 'NONE',  ( 0.5000000000000009992, -6.123233995736778362E-17, 0.8660254037844380415 ) ) ;
#12279=ORIENTED_EDGE ( 'NONE', *, *, #6824, .F. ) ;
#12280=ORIENTED_EDGE ( 'NONE', *, *, #6005, .F. ) ;
#12281=ORIENTED_EDGE ( 'NONE', *, *, #11221, .F. ) ;
#12282=AXIS2_PLACEMENT_3D ( 'NONE', #4754, #3541, #7853 ) ;
#12283=DIRECTION ( 'NONE',  ( 0.000000000000000000, 0.000000000000000000, 1.000000000000000000 ) ) ;
#12286=EDGE_LOOP ( 'NONE', ( #13824, #9871, #14949, #7252, #2037 ) ) ;
#12288=ORIENTED_EDGE ( 'NONE', *, *, #3711, .F. ) ;
#12290=CARTESIAN_POINT ( 'NONE',  ( -52.83493649053890806, 0.000000000000000000, -11.74999999999999822 ) ) ;
#12291=EDGE_CURVE ( 'NONE', #5635, #11081, #4463, .T. ) ;
#12292=DIRECTION ( 'NONE',  ( -0.000000000000000000, -0.000000000000000000, 1.000000000000000000 ) ) ;
#12293=EDGE_CURVE ( 'NONE', #9491, #7296, #10057, .T. ) ;
#12296=DIRECTION ( 'NONE',  ( 0.000000000000000000, 0.000000000000000000, 1.000000000000000000 ) ) ;
#12298=DIRECTION ( 'NONE',  ( 1.000000000000000000, 0.000000000000000000, 0.000000000000000000 ) ) ;
#12299=AXIS2_PLACEMENT_3D ( 'NONE', #9788, #14439, #1830 ) ;
#12300=ORIENTED_EDGE ( 'NONE', *, *, #14805, .F. ) ;
#12301=EDGE_CURVE ( 'NONE', #7513, #13798, #1549, .T. ) ;
#12302=ORIENTED_EDGE ( 'NONE', *, *, #6328, .F. ) ;
#12308=DIRECTION ( 'NONE',  ( 0.000000000000000000, 0.000000000000000000, 1.000000000000000000 ) ) ;
#12309=EDGE_CURVE ( 'NONE', #5327, #4514, #8326, .T. ) ;
#12311=EDGE_LOOP ( 'NONE', ( #3828, #14813, #14876, #188, #4259, #6133 ) ) ;
#12312=CARTESIAN_POINT ( 'NONE',  ( -71.53347797788819662, -69.16568774265570596, -8.000000000000000000 ) ) ;
#12316=VERTEX_POINT ( 'NONE', #726 ) ;
#12318=CIRCLE ( 'NONE', #3594, 50.00000000000000000 ) ;
#12320=DIRECTION ( 'NONE',  ( 0.000000000000000000, 0.000000000000000000, -1.000000000000000000 ) ) ;
#12321=ORIENTED_EDGE ( 'NONE', *, *, #9613, .F. ) ;
#12323=CARTESIAN_POINT ( 'NONE',  ( 37.12029293941379393, 89.61631465359479876, -13.00000000000000178 ) ) ;
#12324=CARTESIAN_POINT ( 'NONE',  ( 51.19406879332056093, 13.71740939043382745, -13.00000000000000178 ) ) ;
#12325=CARTESIAN_POINT ( 'NONE',  ( -7.383907457637922889, -52.72775723226778410, -13.00000000000000178 ) ) ;
#12326=CARTESIAN_POINT ( 'NONE',  ( -22.33583958711380646, -30.74264578624812927, -28.00000000000000000 ) ) ;
#12327=DIRECTION ( 'NONE',  ( 1.000000000000000000, 0.000000000000000000, 0.000000000000000000 ) ) ;
#12328=DIRECTION ( 'NONE',  ( 0.000000000000000000, 0.000000000000000000, 1.000000000000000000 ) ) ;
#12329=ADVANCED_FACE ( 'NONE', ( #4076 ), #7546, .T. ) ;
#12330=EDGE_LOOP ( 'NONE', ( #15023, #7298, #280, #13796, #14097, #3614, #5257, #6050, #5181, #5897 ) ) ;
#12331=EDGE_CURVE ( 'NONE', #12974, #2645, #7353, .T. ) ;
#12332=DIRECTION ( 'NONE',  ( -0.000000000000000000, -0.000000000000000000, -1.000000000000000000 ) ) ;
#12333=DIRECTION ( 'NONE',  ( 1.000000000000000000, 0.000000000000000000, 0.000000000000000000 ) ) ;
#12336=VERTEX_POINT ( 'NONE', #6549 ) ;
#12338=EDGE_CURVE ( 'NONE', #14269, #11532, #3240, .T. ) ;
#12339=CYLINDRICAL_SURFACE ( 'NONE', #10221, 0.5000000000000043299 ) ;
#12340=ORIENTED_EDGE ( 'NONE', *, *, #1398, .T. ) ;
#12342=DIRECTION ( 'NONE',  ( 1.000000000000000000, 0.000000000000000000, 0.000000000000000000 ) ) ;
#12344=CARTESIAN_POINT ( 'NONE',  ( -9.706953719245875689, -57.06275842387046993, -13.00000000000000178 ) ) ;
#12346=EDGE_LOOP ( 'NONE', ( #8275, #2004, #12923, #4223, #14098, #9907, #4926, #12233, #4024, #3730, #12925 ) ) ;
#12349=DIRECTION ( 'NONE',  ( 0.000000000000000000, 0.000000000000000000, -1.000000000000000000 ) ) ;
#12352=CIRCLE ( 'NONE', #15019, 59.50000000000000000 ) ;
#12355=DIRECTION ( 'NONE',  ( 1.000000000000000000, 0.000000000000000000, 0.000000000000000000 ) ) ;
#12356=CARTESIAN_POINT ( 'NONE',  ( 49.57224306869053976, -6.526309611002402811, -8.000000000000000000 ) ) ;
#12357=AXIS2_PLACEMENT_3D ( 'NONE', #9397, #9328, #4563 ) ;
#12358=ORIENTED_EDGE ( 'NONE', *, *, #12594, .F. ) ;
#12359=CARTESIAN_POINT ( 'NONE',  ( -32.26435573746199736, 42.04772703543562073, 8.000000000000000000 ) ) ;
#12364=EDGE_CURVE ( 'NONE', #9738, #9553, #6046, .T. ) ;
#12365=AXIS2_PLACEMENT_3D ( 'NONE', #2603, #7221, #3900 ) ;
#12368=CIRCLE ( 'NONE', #5806, 100.0000000000000000 ) ;
#12369=EDGE_CURVE ( 'NONE', #1906, #3649, #8565, .T. ) ;
#12370=AXIS2_PLACEMENT_3D ( 'NONE', #14925, #11730, #13782 ) ;
#12371=EDGE_CURVE ( 'NONE', #4717, #14193, #14387, .T. ) ;
#12372=AXIS2_PLACEMENT_3D ( 'NONE', #6586, #12375, #13363 ) ;
#12375=DIRECTION ( 'NONE',  ( -0.000000000000000000, -0.000000000000000000, -1.000000000000000000 ) ) ;
#12376=AXIS2_PLACEMENT_3D ( 'NONE', #5625, #13599, #14824 ) ;
#12377=LINE ( 'NONE', #2964, #9185 ) ;
#12378=ORIENTED_EDGE ( 'NONE', *, *, #5636, .F. ) ;
#12379=AXIS2_PLACEMENT_3D ( 'NONE', #3324, #6789, #10144 ) ;
#12381=AXIS2_PLACEMENT_3D ( 'NONE', #1368, #7189, #5979 ) ;
#12382=CARTESIAN_POINT ( 'NONE',  ( -12.86891638962156215, 56.43380494353993271, -10.50000000000000000 ) ) ;
#12383=DIRECTION ( 'NONE',  ( 0.000000000000000000, 0.000000000000000000, 1.000000000000000000 ) ) ;
#12386=EDGE_CURVE ( 'NONE', #7029, #7912, #11989, .T. ) ;
#12387=ADVANCED_FACE ( 'NONE', ( #11518 ), #9364, .F. ) ;
#12389=AXIS2_PLACEMENT_3D ( 'NONE', #5683, #2274, #13816 ) ;
#12390=FACE_BOUND ( 'NONE', #1498, .T. ) ;
#12392=DIRECTION ( 'NONE',  ( -0.000000000000000000, -0.000000000000000000, -1.000000000000000000 ) ) ;
#12393=AXIS2_PLACEMENT_3D ( 'NONE', #10891, #9661, #1566 ) ;
#12394=ORIENTED_EDGE ( 'NONE', *, *, #6983, .F. ) ;
#12395=CARTESIAN_POINT ( 'NONE',  ( 0.000000000000000000, 0.000000000000000000, -10.50000000000000000 ) ) ;
#12397=CARTESIAN_POINT ( 'NONE',  ( 37.02125851216354846, -90.10640870805738700, -10.50000000000000000 ) ) ;
#12398=LINE ( 'NONE', #11264, #710 ) ;
#12401=AXIS2_PLACEMENT_3D ( 'NONE', #678, #600, #11148 ) ;
#12402=ORIENTED_EDGE ( 'NONE', *, *, #11458, .F. ) ;
#12404=CIRCLE ( 'NONE', #1217, 59.50000000000000000 ) ;
#12405=DIRECTION ( 'NONE',  ( -1.000000000000000000, 0.000000000000000000, 0.000000000000000000 ) ) ;
#12406=CIRCLE ( 'NONE', #11928, 3.000000000000002665 ) ;
#12409=ORIENTED_EDGE ( 'NONE', *, *, #5416, .F. ) ;
#12410=LINE ( 'NONE', #2005, #10947 ) ;
#12411=ORIENTED_EDGE ( 'NONE', *, *, #6543, .F. ) ;
#12413=DIRECTION ( 'NONE',  ( 0.000000000000000000, 0.000000000000000000, 1.000000000000000000 ) ) ;
#12414=CYLINDRICAL_SURFACE ( 'NONE', #4426, 0.5000000000000004441 ) ;
#12416=EDGE_CURVE ( 'NONE', #13772, #3549, #2022, .T. ) ;
#12417=CYLINDRICAL_SURFACE ( 'NONE', #7748, 3.000000000000002665 ) ;
#12418=CIRCLE ( 'NONE', #5858, 63.00000000000000000 ) ;
#12421=VERTEX_POINT ( 'NONE', #1037 ) ;
#12422=VERTEX_POINT ( 'NONE', #15001 ) ;
#12425=ADVANCED_FACE ( 'NONE', ( #4453 ), #10270, .T. ) ;
#12427=CARTESIAN_POINT ( 'NONE',  ( 37.21932736666271779, -89.12622059913267947, -10.50000000000000000 ) ) ;
#12428=CARTESIAN_POINT ( 'NONE',  ( 33.48561063518626923, -47.21331623427104063, -10.50000000000000000 ) ) ;
#12429=VERTEX_POINT ( 'NONE', #10286 ) ;
#12430=AXIS2_PLACEMENT_3D ( 'NONE', #14609, #14523, #10034 ) ;
#12431=VERTEX_POINT ( 'NONE', #14930 ) ;
#12432=EDGE_CURVE ( 'NONE', #7912, #6631, #13927, .T. ) ;
#12433=ORIENTED_EDGE ( 'NONE', *, *, #7488, .F. ) ;
#12434=EDGE_CURVE ( 'NONE', #11559, #12743, #11250, .T. ) ;
#12436=AXIS2_PLACEMENT_3D ( 'NONE', #3317, #8228, #5734 ) ;
#12437=CARTESIAN_POINT ( 'NONE',  ( -3.492805317593278058, 46.55633131742322917, -10.50000000000000000 ) ) ;
#12440=ORIENTED_EDGE ( 'NONE', *, *, #6099, .T. ) ;
#12441=CARTESIAN_POINT ( 'NONE',  ( 23.51438936481372366, 47.21331623427104063, 8.000000000000000000 ) ) ;
#12443=ORIENTED_EDGE ( 'NONE', *, *, #6274, .F. ) ;
#12444=EDGE_CURVE ( 'NONE', #2878, #11690, #957, .T. ) ;
#12445=CARTESIAN_POINT ( 'NONE',  ( 1.674280531759317014, -94.51066581171355097, -13.00000000000000178 ) ) ;
#12446=AXIS2_PLACEMENT_3D ( 'NONE', #8317, #5132, #351 ) ;
#12447=ORIENTED_EDGE ( 'NONE', *, *, #441, .T. ) ;
#12448=CIRCLE ( 'NONE', #10498, 0.5000000000000004441 ) ;
#12449=ORIENTED_EDGE ( 'NONE', *, *, #10073, .T. ) ;
#12451=AXIS2_PLACEMENT_3D ( 'NONE', #7367, #6221, #14357 ) ;
#12453=CARTESIAN_POINT ( 'NONE',  ( 6.917888187663118416, 52.54657765281190507, -10.50000000000000000 ) ) ;
#12455=CARTESIAN_POINT ( 'NONE',  ( 0.000000000000000000, 0.000000000000000000, 10.50000000000000000 ) ) ;
#12457=DIRECTION ( 'NONE',  ( 0.000000000000000000, 0.000000000000000000, 1.000000000000000000 ) ) ;
#12458=VECTOR ( 'NONE', #10902, 1000.000000000000000 ) ;
#12459=ORIENTED_EDGE ( 'NONE', *, *, #10787, .T. ) ;
#12460=CYLINDRICAL_SURFACE ( 'NONE', #509, 57.00000000000000000 ) ;
#12462=DIRECTION ( 'NONE',  ( 1.000000000000000000, -1.749300984178292964E-15, 0.000000000000000000 ) ) ;
#12463=CYLINDRICAL_SURFACE ( 'NONE', #10684, 3.000000000000002665 ) ;
#12464=CIRCLE ( 'NONE', #10516, 3.000000000000002665 ) ;
#12465=ORIENTED_EDGE ( 'NONE', *, *, #10283, .F. ) ;
#12466=DIRECTION ( 'NONE',  ( 0.000000000000000000, 0.000000000000000000, -1.000000000000000000 ) ) ;
#12467=ORIENTED_EDGE ( 'NONE', *, *, #11019, .F. ) ;
#12468=CARTESIAN_POINT ( 'NONE',  ( 26.49999999999971578, 45.89934640057541060, 10.49999999999999822 ) ) ;
#12470=CARTESIAN_POINT ( 'NONE',  ( 0.000000000000000000, 0.000000000000000000, 8.000000000000000000 ) ) ;
#12472=DIRECTION ( 'NONE',  ( 1.000000000000000000, 0.000000000000000000, 0.000000000000000000 ) ) ;
#12473=CARTESIAN_POINT ( 'NONE',  ( 0.000000000000000000, 0.000000000000000000, 8.000000000000000000 ) ) ;
#12474=VECTOR ( 'NONE', #439, 1000.000000000000000 ) ;
#12476=AXIS2_PLACEMENT_3D ( 'NONE', #7009, #5741, #14944 ) ;
#12477=CARTESIAN_POINT ( 'NONE',  ( 22.33583958711425055, -30.74264578624780597, -28.00000000000000000 ) ) ;
#12478=EDGE_CURVE ( 'NONE', #11670, #14615, #5664, .T. ) ;
#12480=EDGE_CURVE ( 'NONE', #9297, #669, #7593, .T. ) ;
#12481=EDGE_CURVE ( 'NONE', #12042, #12813, #1071, .T. ) ;
#12483=ORIENTED_EDGE ( 'NONE', *, *, #3109, .F. ) ;
#12485=CARTESIAN_POINT ( 'NONE',  ( 42.04772703543530099, 32.26435573746242369, 8.000000000000000000 ) ) ;
#12486=AXIS2_PLACEMENT_3D ( 'NONE', #13932, #12708, #1104 ) ;
#12487=AXIS2_PLACEMENT_3D ( 'NONE', #14552, #2711, #2858 ) ;
#12488=FACE_OUTER_BOUND ( 'NONE', #9088, .T. ) ;
#12489=AXIS2_PLACEMENT_3D ( 'NONE', #10260, #10404, #4646 ) ;
#12490=CIRCLE ( 'NONE', #14670, 63.00000000000000000 ) ;
#12491=CARTESIAN_POINT ( 'NONE',  ( -31.05588327715806329, 44.79355920668842828, -8.000000000000000000 ) ) ;
#12492=VERTEX_POINT ( 'NONE', #2316 ) ;
#12493=DIRECTION ( 'NONE',  ( 0.000000000000000000, 0.000000000000000000, 1.000000000000000000 ) ) ;
#12495=DIRECTION ( 'NONE',  ( 0.000000000000000000, 0.000000000000000000, 1.000000000000000000 ) ) ;
#12496=LINE ( 'NONE', #4225, #8043 ) ;
#12497=ORIENTED_EDGE ( 'NONE', *, *, #9520, .F. ) ;
#12499=DIRECTION ( 'NONE',  ( 1.000000000000000000, 1.765157221169382931E-15, 0.000000000000000000 ) ) ;
#12501=AXIS2_PLACEMENT_3D ( 'NONE', #1499, #8466, #11757 ) ;
#12503=ORIENTED_EDGE ( 'NONE', *, *, #11021, .T. ) ;
#12507=CARTESIAN_POINT ( 'NONE',  ( 0.000000000000000000, 0.000000000000000000, -11.74999999999999822 ) ) ;
#12509=AXIS2_PLACEMENT_3D ( 'NONE', #916, #4481, #2187 ) ;
#12510=EDGE_LOOP ( 'NONE', ( #3598, #8730, #10599, #11369, #7222, #6211 ) ) ;
#12511=ORIENTED_EDGE ( 'NONE', *, *, #11867, .F. ) ;
#12512=DIRECTION ( 'NONE',  ( 0.000000000000000000, 0.000000000000000000, -1.000000000000000000 ) ) ;
#12515=DIRECTION ( 'NONE',  ( -0.000000000000000000, -0.000000000000000000, 1.000000000000000000 ) ) ;
#12516=AXIS2_PLACEMENT_3D ( 'NONE', #2174, #13961, #3473 ) ;
#12517=CIRCLE ( 'NONE', #7898, 63.00000000000000000 ) ;
#12519=CARTESIAN_POINT ( 'NONE',  ( 12.94095225512608494, -48.29629131445340562, -8.000000000000000000 ) ) ;
#12520=CARTESIAN_POINT ( 'NONE',  ( -9.706953719245875689, -57.06275842387046993, 8.000000000000000000 ) ) ;
#12521=EDGE_LOOP ( 'NONE', ( #3561, #12820, #10388, #8041 ) ) ;
#12523=EDGE_CURVE ( 'NONE', #13856, #2085, #13663, .T. ) ;
#12524=EDGE_CURVE ( 'NONE', #13552, #11211, #334, .T. ) ;
#12529=CIRCLE ( 'NONE', #3314, 50.00000000000000000 ) ;
#12531=DIRECTION ( 'NONE',  ( 0.000000000000000000, 0.000000000000000000, 1.000000000000000000 ) ) ;
#12533=DIRECTION ( 'NONE',  ( 0.000000000000000000, 0.000000000000000000, -1.000000000000000000 ) ) ;
#12534=DIRECTION ( 'NONE',  ( -0.000000000000000000, -0.000000000000000000, 1.000000000000000000 ) ) ;
#12537=AXIS2_PLACEMENT_3D ( 'NONE', #9812, #2989, #713 ) ;
#12541=DIRECTION ( 'NONE',  ( -0.000000000000000000, -0.000000000000000000, -1.000000000000000000 ) ) ;
#12542=CARTESIAN_POINT ( 'NONE',  ( 36.70371619500516402, 89.33979373934434420, -13.00000000000000178 ) ) ;
#12543=ORIENTED_EDGE ( 'NONE', *, *, #9624, .T. ) ;
#12545=VERTEX_POINT ( 'NONE', #14076 ) ;
#12546=DIRECTION ( 'NONE',  ( -1.000000000000000000, 9.329605248950895679E-16, 0.000000000000000000 ) ) ;
#12547=FACE_OUTER_BOUND ( 'NONE', #13874, .T. ) ;
#12548=CARTESIAN_POINT ( 'NONE',  ( 49.00442420935993226, -30.80502811811213704, -8.000000000000000000 ) ) ;
#12549=DIRECTION ( 'NONE',  ( 1.000000000000000000, 0.000000000000000000, 0.000000000000000000 ) ) ;
#12551=CYLINDRICAL_SURFACE ( 'NONE', #3407, 63.00000000000000000 ) ;
#12554=EDGE_LOOP ( 'NONE', ( #10296, #795, #6448, #4616 ) ) ;
#12555=DIRECTION ( 'NONE',  ( 1.000000000000000000, 0.000000000000000000, 0.000000000000000000 ) ) ;
#12558=PLANE ( 'NONE',  #8309 ) ;
#12559=CARTESIAN_POINT ( 'NONE',  ( -4.121772567811602173, -51.45950017607692217, -13.00000000000000178 ) ) ;
#12560=ORIENTED_EDGE ( 'NONE', *, *, #7585, .T. ) ;
#12561=EDGE_CURVE ( 'NONE', #297, #8589, #11500, .T. ) ;
#12562=DIRECTION ( 'NONE',  ( 1.000000000000000000, 0.000000000000000000, 0.000000000000000000 ) ) ;
#12565=DIRECTION ( 'NONE',  ( 1.000000000000000000, 0.000000000000000000, 0.000000000000000000 ) ) ;
#12567=CIRCLE ( 'NONE', #11029, 100.0000000000000000 ) ;
#12568=DIRECTION ( 'NONE',  ( 1.000000000000000000, 0.000000000000000000, 0.000000000000000000 ) ) ;
#12569=DIRECTION ( 'NONE',  ( -0.000000000000000000, -0.000000000000000000, -1.000000000000000000 ) ) ;
#12570=ORIENTED_EDGE ( 'NONE', *, *, #13823, .F. ) ;
#12572=DIRECTION ( 'NONE',  ( 1.000000000000000000, 0.000000000000000000, 0.000000000000000000 ) ) ;
#12575=DIRECTION ( 'NONE',  ( 0.000000000000000000, 0.000000000000000000, -1.000000000000000000 ) ) ;
#12576=VERTEX_POINT ( 'NONE', #5112 ) ;
#12577=ORIENTED_EDGE ( 'NONE', *, *, #2480, .T. ) ;
#12578=ADVANCED_FACE ( 'NONE', ( #14154 ), #12040, .T. ) ;
#12579=ORIENTED_EDGE ( 'NONE', *, *, #3943, .F. ) ;
#12584=DIRECTION ( 'NONE',  ( 0.000000000000000000, 0.000000000000000000, 1.000000000000000000 ) ) ;
#12585=CARTESIAN_POINT ( 'NONE',  ( -49.54657765281192638, 6.917888187662934563, 8.000000000000000000 ) ) ;
#12586=ORIENTED_EDGE ( 'NONE', *, *, #3575, .F. ) ;
#12587=DIRECTION ( 'NONE',  ( 0.000000000000000000, 0.000000000000000000, -1.000000000000000000 ) ) ;
#12589=VERTEX_POINT ( 'NONE', #3608 ) ;
#12590=ORIENTED_EDGE ( 'NONE', *, *, #2605, .F. ) ;
#12591=PLANE ( 'NONE',  #8140 ) ;
#12592=ORIENTED_EDGE ( 'NONE', *, *, #11259, .F. ) ;
#12594=EDGE_CURVE ( 'NONE', #6415, #212, #1627, .T. ) ;
#12595=VECTOR ( 'NONE', #7501, 1000.000000000000000 ) ;
#12597=EDGE_CURVE ( 'NONE', #14933, #13551, #8097, .T. ) ;
#12598=ADVANCED_FACE ( 'NONE', ( #8222 ), #9585, .F. ) ;
#12599=CARTESIAN_POINT ( 'NONE',  ( -3.492805317593278058, 46.55633131742322917, -10.50000000000000000 ) ) ;
#12604=CARTESIAN_POINT ( 'NONE',  ( -24.98583958711379793, -30.74264578624812927, -28.00000000000000000 ) ) ;
#12605=AXIS2_PLACEMENT_3D ( 'NONE', #3106, #13504, #603 ) ;
#12606=EDGE_CURVE ( 'NONE', #2333, #14343, #4237, .T. ) ;
#12607=CARTESIAN_POINT ( 'NONE',  ( -13.35619814848797837, 51.53979475227131246, -10.50000000000000000 ) ) ;
#12608=AXIS2_PLACEMENT_3D ( 'NONE', #11560, #6965, #2348 ) ;
#12610=AXIS2_PLACEMENT_3D ( 'NONE', #10785, #13069, #4873 ) ;
#12611=ORIENTED_EDGE ( 'NONE', *, *, #5967, .T. ) ;
#12612=FACE_OUTER_BOUND ( 'NONE', #10309, .T. ) ;
#12613=ORIENTED_EDGE ( 'NONE', *, *, #3984, .F. ) ;
#12614=FACE_OUTER_BOUND ( 'NONE', #7862, .T. ) ;
#12615=LINE ( 'NONE', #1089, #14077 ) ;
#12616=EDGE_CURVE ( 'NONE', #4787, #11326, #11998, .T. ) ;
#12618=EDGE_CURVE ( 'NONE', #9852, #4454, #5189, .T. ) ;
#12619=CARTESIAN_POINT ( 'NONE',  ( -7.383907457637922889, -52.72775723226778410, 10.49999999999999822 ) ) ;
#12620=CARTESIAN_POINT ( 'NONE',  ( -50.84834283437000835, -14.07862063237876704, -13.00000000000000178 ) ) ;
#12621=CARTESIAN_POINT ( 'NONE',  ( -37.12029293941441210, -89.61631465359452875, -13.00000000000000178 ) ) ;
#12622=CIRCLE ( 'NONE', #10910, 0.5000000000000004441 ) ;
#12623=FACE_OUTER_BOUND ( 'NONE', #13567, .T. ) ;
#12624=CIRCLE ( 'NONE', #12867, 60.49999999999999289 ) ;
#12626=CARTESIAN_POINT ( 'NONE',  ( -13.71740939043329277, 51.19406879332069593, -13.00000000000000178 ) ) ;
#12627=CARTESIAN_POINT ( 'NONE',  ( 34.62083247296202160, 87.95718916809205723, -8.000000000000000000 ) ) ;
#12628=AXIS2_PLACEMENT_3D ( 'NONE', #1069, #9248, #11694 ) ;
#12629=DIRECTION ( 'NONE',  ( -1.000000000000000000, 0.000000000000000000, 0.000000000000000000 ) ) ;
#12630=CIRCLE ( 'NONE', #5589, 0.5000000000000004441 ) ;
#12631=DIRECTION ( 'NONE',  ( 0.000000000000000000, 0.000000000000000000, -1.000000000000000000 ) ) ;
#12632=AXIS2_PLACEMENT_3D ( 'NONE', #9889, #489, #12188 ) ;
#12633=VERTEX_POINT ( 'NONE', #8450 ) ;
#12634=CARTESIAN_POINT ( 'NONE',  ( 68.58935777509475429, -68.58935777509547904, -13.00000000000000178 ) ) ;
#12637=PLANE ( 'NONE',  #5393 ) ;
#12638=AXIS2_PLACEMENT_3D ( 'NONE', #12908, #10549, #153 ) ;
#12639=CIRCLE ( 'NONE', #8273, 59.50000000000000000 ) ;
#12640=CARTESIAN_POINT ( 'NONE',  ( 29.51438936481373077, 47.21331623427104063, -8.000000000000000000 ) ) ;
#12643=CIRCLE ( 'NONE', #9231, 3.000000000000002665 ) ;
#12644=ORIENTED_EDGE ( 'NONE', *, *, #8463, .F. ) ;
#12645=VERTEX_POINT ( 'NONE', #7156 ) ;
#12646=CIRCLE ( 'NONE', #6081, 60.50000000000000000 ) ;
#12647=ORIENTED_EDGE ( 'NONE', *, *, #10561, .T. ) ;
#12649=EDGE_CURVE ( 'NONE', #10590, #3770, #343, .T. ) ;
#12650=DIRECTION ( 'NONE',  ( 0.000000000000000000, 0.000000000000000000, 1.000000000000000000 ) ) ;
#12652=DIRECTION ( 'NONE',  ( 0.000000000000000000, 0.000000000000000000, 1.000000000000000000 ) ) ;
#12655=ORIENTED_EDGE ( 'NONE', *, *, #11662, .T. ) ;
#12657=VECTOR ( 'NONE', #8910, 1000.000000000000000 ) ;
#12662=ORIENTED_EDGE ( 'NONE', *, *, #10242, .T. ) ;
#12663=DIRECTION ( 'NONE',  ( -1.000000000000000000, 0.000000000000000000, 0.000000000000000000 ) ) ;
#12664=ORIENTED_EDGE ( 'NONE', *, *, #1565, .T. ) ;
#12666=ORIENTED_EDGE ( 'NONE', *, *, #11216, .F. ) ;
#12667=EDGE_CURVE ( 'NONE', #11211, #5988, #12464, .T. ) ;
#12668=EDGE_CURVE ( 'NONE', #2406, #1338, #8338, .T. ) ;
#12669=CARTESIAN_POINT ( 'NONE',  ( -68.58935777509570642, -68.58935777509452691, -8.000000000000000000 ) ) ;
#12671=AXIS2_PLACEMENT_3D ( 'NONE', #13242, #7224, #1548 ) ;
#12673=ORIENTED_EDGE ( 'NONE', *, *, #12434, .T. ) ;
#12675=ORIENTED_EDGE ( 'NONE', *, *, #3818, .F. ) ;
#12676=CIRCLE ( 'NONE', #6114, 59.50000000000000000 ) ;
#12677=ORIENTED_EDGE ( 'NONE', *, *, #5409, .T. ) ;
#12678=DIRECTION ( 'NONE',  ( 0.000000000000000000, 0.000000000000000000, 1.000000000000000000 ) ) ;
#12680=AXIS2_PLACEMENT_3D ( 'NONE', #12473, #8963, #707 ) ;
#12682=CARTESIAN_POINT ( 'NONE',  ( -49.00442420935969778, 30.80502811811250297, -13.00000000000000178 ) ) ;
#12683=PLANE ( 'NONE',  #7245 ) ;
#12684=ORIENTED_EDGE ( 'NONE', *, *, #4678, .F. ) ;
#12685=CARTESIAN_POINT ( 'NONE',  ( 32.26435573746228158, -42.04772703543541468, 8.000000000000000000 ) ) ;
#12686=CIRCLE ( 'NONE', #5411, 63.00000000000000000 ) ;
#12688=ADVANCED_FACE ( 'NONE', ( #10957 ), #3071, .T. ) ;
#12689=ORIENTED_EDGE ( 'NONE', *, *, #1034, .T. ) ;
#12690=FACE_OUTER_BOUND ( 'NONE', #2972, .T. ) ;
#12691=AXIS2_PLACEMENT_3D ( 'NONE', #4470, #2470, #5743 ) ;
#12693=DIRECTION ( 'NONE',  ( 1.000000000000000000, 0.000000000000000000, 0.000000000000000000 ) ) ;
#12695=DIRECTION ( 'NONE',  ( 0.000000000000000000, 0.000000000000000000, 1.000000000000000000 ) ) ;
#12698=LINE ( 'NONE', #10934, #12595 ) ;
#12699=DIRECTION ( 'NONE',  ( -0.000000000000000000, -0.000000000000000000, 1.000000000000000000 ) ) ;
#12701=ORIENTED_EDGE ( 'NONE', *, *, #14201, .T. ) ;
#12702=FACE_OUTER_BOUND ( 'NONE', #3506, .T. ) ;
#12705=EDGE_CURVE ( 'NONE', #4759, #8664, #8669, .T. ) ;
#12706=FACE_OUTER_BOUND ( 'NONE', #6150, .T. ) ;
#12707=ORIENTED_EDGE ( 'NONE', *, *, #7358, .T. ) ;
#12708=DIRECTION ( 'NONE',  ( -0.000000000000000000, -0.000000000000000000, 1.000000000000000000 ) ) ;
#12709=EDGE_LOOP ( 'NONE', ( #13609, #8878, #2389, #3222 ) ) ;
#12711=CIRCLE ( 'NONE', #4955, 3.000000000000002665 ) ;
#12712=CIRCLE ( 'NONE', #1116, 100.0000000000000000 ) ;
#12713=CARTESIAN_POINT ( 'NONE',  ( -39.30189486418265687, -33.47282819776598473, -8.000000000000000000 ) ) ;
#12714=CIRCLE ( 'NONE', #3251, 50.00000000000000000 ) ;
#12715=ORIENTED_EDGE ( 'NONE', *, *, #8008, .T. ) ;
#12717=DIRECTION ( 'NONE',  ( 0.000000000000000000, 0.000000000000000000, 1.000000000000000000 ) ) ;
#12718=EDGE_CURVE ( 'NONE', #7912, #9770, #14896, .T. ) ;
#12719=CARTESIAN_POINT ( 'NONE',  ( -92.55687898036933348, -36.52608637591544039, 8.000000000000000000 ) ) ;
#12720=DIRECTION ( 'NONE',  ( -1.000000000000000000, 0.000000000000000000, 0.000000000000000000 ) ) ;
#12721=EDGE_LOOP ( 'NONE', ( #3574, #3194, #9610, #5494, #12033, #15009, #6881 ) ) ;
#12722=CIRCLE ( 'NONE', #11271, 3.000000000000002665 ) ;
#12724=FACE_OUTER_BOUND ( 'NONE', #8409, .T. ) ;
#12726=VECTOR ( 'NONE', #5588, 1000.000000000000000 ) ;
#12727=EDGE_CURVE ( 'NONE', #1124, #11178, #3010, .T. ) ;
#12729=VERTEX_POINT ( 'NONE', #13244 ) ;
#12730=ORIENTED_EDGE ( 'NONE', *, *, #3711, .T. ) ;
#12731=CIRCLE ( 'NONE', #3267, 56.99999999999999289 ) ;
#12732=ORIENTED_EDGE ( 'NONE', *, *, #13458, .T. ) ;
#12734=AXIS2_PLACEMENT_3D ( 'NONE', #8621, #10754, #13267 ) ;
#12735=CIRCLE ( 'NONE', #5926, 63.00000000000000000 ) ;
#12739=CARTESIAN_POINT ( 'NONE',  ( 46.63108361037843252, 56.43380494353993271, 10.49999999999999822 ) ) ;
#12741=CYLINDRICAL_SURFACE ( 'NONE', #7163, 56.99999999999999289 ) ;
#12743=VERTEX_POINT ( 'NONE', #2985 ) ;
#12744=ORIENTED_EDGE ( 'NONE', *, *, #8299, .F. ) ;
#12746=CARTESIAN_POINT ( 'NONE',  ( -30.43807145043581741, 39.66766701456192834, -8.000000000000000000 ) ) ;
#12747=CIRCLE ( 'NONE', #11042, 52.50000000000000711 ) ;
#12750=DIRECTION ( 'NONE',  ( 0.000000000000000000, 0.000000000000000000, 1.000000000000000000 ) ) ;
#12751=ADVANCED_FACE ( 'NONE', ( #4128 ), #1994, .F. ) ;
#12752=ORIENTED_EDGE ( 'NONE', *, *, #9890, .F. ) ;
#12756=LINE ( 'NONE', #1210, #7062 ) ;
#12757=EDGE_CURVE ( 'NONE', #8704, #8856, #13677, .T. ) ;
#12759=DIRECTION ( 'NONE',  ( -1.000000000000000000, 1.065814103640150279E-14, 0.000000000000000000 ) ) ;
#12760=DIRECTION ( 'NONE',  ( 0.000000000000000000, 0.000000000000000000, 1.000000000000000000 ) ) ;
#12761=ORIENTED_EDGE ( 'NONE', *, *, #7656, .F. ) ;
#12763=VERTEX_POINT ( 'NONE', #11039 ) ;
#12764=EDGE_CURVE ( 'NONE', #11742, #14537, #1913, .T. ) ;
#12766=ORIENTED_EDGE ( 'NONE', *, *, #11502, .F. ) ;
#12768=EDGE_CURVE ( 'NONE', #4523, #8947, #14161, .T. ) ;
#12769=FACE_OUTER_BOUND ( 'NONE', #601, .T. ) ;
#12773=DIRECTION ( 'NONE',  ( -0.000000000000000000, -0.000000000000000000, -1.000000000000000000 ) ) ;
#12774=CARTESIAN_POINT ( 'NONE',  ( 32.26435573746228158, -42.04772703543541468, -10.50000000000000000 ) ) ;
#12775=DIRECTION ( 'NONE',  ( 0.000000000000000000, 0.000000000000000000, -1.000000000000000000 ) ) ;
#12777=AXIS2_PLACEMENT_3D ( 'NONE', #7913, #9196, #3360 ) ;
#12778=DIRECTION ( 'NONE',  ( 1.000000000000000000, 1.749300984178292964E-15, 0.000000000000000000 ) ) ;
#12780=DIRECTION ( 'NONE',  ( -1.000000000000000000, 0.000000000000000000, 0.000000000000000000 ) ) ;
#12781=VERTEX_POINT ( 'NONE', #13385 ) ;
#12783=CARTESIAN_POINT ( 'NONE',  ( 0.000000000000000000, 0.000000000000000000, -13.00000000000000178 ) ) ;
#12784=DIRECTION ( 'NONE',  ( 0.000000000000000000, 0.000000000000000000, -1.000000000000000000 ) ) ;
#12785=LINE ( 'NONE', #3529, #5920 ) ;
#12786=ORIENTED_EDGE ( 'NONE', *, *, #8008, .F. ) ;
#12788=VERTEX_POINT ( 'NONE', #7609 ) ;
#12790=PLANE ( 'NONE',  #1514 ) ;
#12791=ADVANCED_FACE ( 'NONE', ( #4210 ), #9962, .F. ) ;
#12792=CARTESIAN_POINT ( 'NONE',  ( 26.00011991137315803, 45.91029614918951296, -13.00000000000000178 ) ) ;
#12793=EDGE_CURVE ( 'NONE', #9152, #11371, #12714, .T. ) ;
#12794=CARTESIAN_POINT ( 'NONE',  ( 0.000000000000000000, 0.000000000000000000, -13.00000000000000178 ) ) ;
#12795=EDGE_CURVE ( 'NONE', #10819, #12492, #7607, .T. ) ;
#12796=VERTEX_POINT ( 'NONE', #14613 ) ;
#12797=CARTESIAN_POINT ( 'NONE',  ( -32.26435573746199736, 42.04772703543562073, 8.000000000000000000 ) ) ;
#12798=DIRECTION ( 'NONE',  ( 0.000000000000000000, 0.000000000000000000, 1.000000000000000000 ) ) ;
#12799=CARTESIAN_POINT ( 'NONE',  ( 0.000000000000000000, 0.000000000000000000, -8.000000000000000000 ) ) ;
#12800=VERTEX_POINT ( 'NONE', #2906 ) ;
#12804=FACE_OUTER_BOUND ( 'NONE', #6956, .T. ) ;
#12805=DIRECTION ( 'NONE',  ( 0.000000000000000000, 0.000000000000000000, 1.000000000000000000 ) ) ;
#12806=EDGE_CURVE ( 'NONE', #490, #11004, #6875, .T. ) ;
#12807=DIRECTION ( 'NONE',  ( -1.000000000000000000, 0.000000000000000000, 0.000000000000000000 ) ) ;
#12809=DIRECTION ( 'NONE',  ( -0.000000000000000000, -0.000000000000000000, 1.000000000000000000 ) ) ;
#12810=EDGE_LOOP ( 'NONE', ( #9769, #4368, #5510, #1284 ) ) ;
#12812=ORIENTED_EDGE ( 'NONE', *, *, #11567, .T. ) ;
#12813=VERTEX_POINT ( 'NONE', #6301 ) ;
#12814=DIRECTION ( 'NONE',  ( -1.000000000000000000, 0.000000000000000000, 0.000000000000000000 ) ) ;
#12815=DIRECTION ( 'NONE',  ( 1.000000000000000000, 0.000000000000000000, 0.000000000000000000 ) ) ;
#12816=ORIENTED_EDGE ( 'NONE', *, *, #8016, .T. ) ;
#12817=ORIENTED_EDGE ( 'NONE', *, *, #12846, .T. ) ;
#12818=DIRECTION ( 'NONE',  ( -1.000000000000000000, -9.854395544204382819E-14, 0.000000000000000000 ) ) ;
#12819=CIRCLE ( 'NONE', #6251, 3.000000000000002665 ) ;
#12820=ORIENTED_EDGE ( 'NONE', *, *, #12301, .F. ) ;
#12821=CARTESIAN_POINT ( 'NONE',  ( 52.72775723226780542, -7.383907457637739036, -10.50000000000000000 ) ) ;
#12822=DIRECTION ( 'NONE',  ( 0.000000000000000000, 0.000000000000000000, 1.000000000000000000 ) ) ;
#12823=CARTESIAN_POINT ( 'NONE',  ( -37.21932736666205699, 89.12622059913296368, -13.00000000000000178 ) ) ;
#12824=DIRECTION ( 'NONE',  ( -0.000000000000000000, -0.000000000000000000, 1.000000000000000000 ) ) ;
#12825=CARTESIAN_POINT ( 'NONE',  ( 56.43380494353997534, 12.86891638962136319, 10.49999999999999822 ) ) ;
#12826=CARTESIAN_POINT ( 'NONE',  ( -91.27544013909712817, 39.61975340586647576, -13.00000000000000178 ) ) ;
#12829=ORIENTED_EDGE ( 'NONE', *, *, #2162, .F. ) ;
#12831=CYLINDRICAL_SURFACE ( 'NONE', #1667, 2.649999999999992806 ) ;
#12834=CIRCLE ( 'NONE', #10645, 100.0000000000000000 ) ;
#12835=CARTESIAN_POINT ( 'NONE',  ( 27.01438936481372721, 47.21331623427104063, -10.50000000000000000 ) ) ;
#12841=DIRECTION ( 'NONE',  ( 1.000000000000000000, 0.000000000000000000, 0.000000000000000000 ) ) ;
#12846=EDGE_CURVE ( 'NONE', #14306, #5756, #5902, .T. ) ;
#12847=DIRECTION ( 'NONE',  ( 0.000000000000000000, 0.000000000000000000, 1.000000000000000000 ) ) ;
#12849=DIRECTION ( 'NONE',  ( -0.000000000000000000, -0.000000000000000000, 1.000000000000000000 ) ) ;
#12851=FACE_OUTER_BOUND ( 'NONE', #7739, .T. ) ;
#12852=EDGE_LOOP ( 'NONE', ( #3844, #2268, #3899, #2199, #2930, #3428, #11851, #13952, #9255, #4484 ) ) ;
#12853=CIRCLE ( 'NONE', #14802, 56.99999999999999289 ) ;
#12854=DIRECTION ( 'NONE',  ( 1.000000000000000000, 0.000000000000000000, 0.000000000000000000 ) ) ;
#12855=VERTEX_POINT ( 'NONE', #2496 ) ;
#12856=VECTOR ( 'NONE', #3958, 1000.000000000000000 ) ;
#12857=DIRECTION ( 'NONE',  ( 1.000000000000000000, 0.000000000000000000, 0.000000000000000000 ) ) ;
#12859=DIRECTION ( 'NONE',  ( 0.000000000000000000, 0.000000000000000000, 1.000000000000000000 ) ) ;
#12860=DIRECTION ( 'NONE',  ( 1.000000000000000000, 0.000000000000000000, 0.000000000000000000 ) ) ;
#12861=AXIS2_PLACEMENT_3D ( 'NONE', #10406, #5703, #2215 ) ;
#12863=CARTESIAN_POINT ( 'NONE',  ( 0.000000000000000000, 0.000000000000000000, 8.000000000000000000 ) ) ;
#12864=CIRCLE ( 'NONE', #3422, 3.000000000000002665 ) ;
#12865=DIRECTION ( 'NONE',  ( 1.000000000000000000, 0.000000000000000000, 0.000000000000000000 ) ) ;
#12866=CIRCLE ( 'NONE', #4393, 50.00000000000000000 ) ;
#12867=AXIS2_PLACEMENT_3D ( 'NONE', #4489, #14965, #3340 ) ;
#12868=DIRECTION ( 'NONE',  ( 1.000000000000000000, 0.000000000000000000, 0.000000000000000000 ) ) ;
#12869=EDGE_LOOP ( 'NONE', ( #9170, #8914, #6572, #6957 ) ) ;
#12871=VERTEX_POINT ( 'NONE', #5558 ) ;
#12872=AXIS2_PLACEMENT_3D ( 'NONE', #1391, #236, #5852 ) ;
#12874=AXIS2_PLACEMENT_3D ( 'NONE', #2343, #12678, #9102 ) ;
#12875=EDGE_CURVE ( 'NONE', #11131, #2090, #213, .T. ) ;
#12877=AXIS2_PLACEMENT_3D ( 'NONE', #9777, #3391, #14866 ) ;
#12879=CIRCLE ( 'NONE', #11428, 0.5000000000000004441 ) ;
#12882=DIRECTION ( 'NONE',  ( 1.000000000000000000, 0.000000000000000000, 0.000000000000000000 ) ) ;
#12884=DIRECTION ( 'NONE',  ( -0.000000000000000000, -0.000000000000000000, -1.000000000000000000 ) ) ;
#12885=ORIENTED_EDGE ( 'NONE', *, *, #7670, .F. ) ;
#12886=ORIENTED_EDGE ( 'NONE', *, *, #5380, .T. ) ;
#12887=EDGE_LOOP ( 'NONE', ( #925, #14639, #7561, #1141, #10234, #2168 ) ) ;
#12888=CARTESIAN_POINT ( 'NONE',  ( -50.69406879332065330, -13.71740939043347041, -10.50000000000000000 ) ) ;
#12890=CIRCLE ( 'NONE', #14834, 0.5000000000000004441 ) ;
#12891=VERTEX_POINT ( 'NONE', #67 ) ;
#12895=VERTEX_POINT ( 'NONE', #4710 ) ;
#12899=CARTESIAN_POINT ( 'NONE',  ( -49.00442420935969778, 30.80502811811250297, -13.00000000000000178 ) ) ;
#12901=DIRECTION ( 'NONE',  ( 0.000000000000000000, 0.000000000000000000, 1.000000000000000000 ) ) ;
#12902=DIRECTION ( 'NONE',  ( -1.000000000000000000, 0.000000000000000000, 0.000000000000000000 ) ) ;
#12905=CARTESIAN_POINT ( 'NONE',  ( 33.49014761921571193, 11.74264578624841171, -25.50000000000000355 ) ) ;
#12906=CIRCLE ( 'NONE', #1265, 53.55662432702593634 ) ;
#12908=CARTESIAN_POINT ( 'NONE',  ( -2.449293598294708880E-16, 38.00000000000000000, -28.00000000000000000 ) ) ;
#12910=CIRCLE ( 'NONE', #1756, 56.99999999999999289 ) ;
#12912=DIRECTION ( 'NONE',  ( 1.000000000000000000, 0.000000000000000000, 0.000000000000000000 ) ) ;
#12914=LINE ( 'NONE', #2505, #9067 ) ;
#12915=AXIS2_PLACEMENT_3D ( 'NONE', #14009, #7993, #29 ) ;
#12918=CARTESIAN_POINT ( 'NONE',  ( 49.00442420935993226, -30.80502811811213704, -13.00000000000000178 ) ) ;
#12919=DIRECTION ( 'NONE',  ( -1.000000000000000000, 0.000000000000000000, 0.000000000000000000 ) ) ;
#12920=CARTESIAN_POINT ( 'NONE',  ( -22.33583958711380646, -30.74264578624812927, -28.00000000000000000 ) ) ;
#12922=AXIS2_PLACEMENT_3D ( 'NONE', #14840, #1101, #2371 ) ;
#12923=ORIENTED_EDGE ( 'NONE', *, *, #12293, .T. ) ;
#12924=DIRECTION ( 'NONE',  ( -1.000000000000000000, 0.000000000000000000, 0.000000000000000000 ) ) ;
#12925=ORIENTED_EDGE ( 'NONE', *, *, #1396, .F. ) ;
#12932=ORIENTED_EDGE ( 'NONE', *, *, #800, .F. ) ;
#12933=EDGE_CURVE ( 'NONE', #1331, #1743, #6637, .T. ) ;
#12935=EDGE_LOOP ( 'NONE', ( #8216, #5568 ) ) ;
#12938=CARTESIAN_POINT ( 'NONE',  ( 33.49014761921571903, 11.74264578624841171, -28.00000000000000000 ) ) ;
#12939=ADVANCED_FACE ( 'NONE', ( #12139 ), #3800, .F. ) ;
#12940=CARTESIAN_POINT ( 'NONE',  ( -3.492805317593278058, 46.55633131742322917, -10.50000000000000000 ) ) ;
#12941=EDGE_CURVE ( 'NONE', #3450, #9063, #12069, .T. ) ;
#12942=CARTESIAN_POINT ( 'NONE',  ( -2.449293598294700991E-16, 97.00000000000000000, -13.00000000000000178 ) ) ;
#12945=CIRCLE ( 'NONE', #14889, 56.99999999999999289 ) ;
#12946=CARTESIAN_POINT ( 'NONE',  ( -26.49999999999971578, -45.89934640057541060, 10.49999999999999822 ) ) ;
#12948=LINE ( 'NONE', #2541, #9549 ) ;
#12949=DIRECTION ( 'NONE',  ( -0.000000000000000000, -0.000000000000000000, -1.000000000000000000 ) ) ;
#12950=AXIS2_PLACEMENT_3D ( 'NONE', #1222, #9262, #14975 ) ;
#12951=ORIENTED_EDGE ( 'NONE', *, *, #4068, .F. ) ;
#12953=EDGE_LOOP ( 'NONE', ( #3110, #12644, #196, #2860, #3215 ) ) ;
#12954=EDGE_CURVE ( 'NONE', #8947, #1277, #14094, .T. ) ;
#12958=AXIS2_PLACEMENT_3D ( 'NONE', #2301, #6986, #13850 ) ;
#12962=ORIENTED_EDGE ( 'NONE', *, *, #11727, .F. ) ;
#12963=VERTEX_POINT ( 'NONE', #2870 ) ;
#12965=CARTESIAN_POINT ( 'NONE',  ( 69.20695371924547601, 57.06275842387054098, -13.00000000000000178 ) ) ;
#12966=DIRECTION ( 'NONE',  ( 0.000000000000000000, 0.000000000000000000, -1.000000000000000000 ) ) ;
#12967=ORIENTED_EDGE ( 'NONE', *, *, #7656, .T. ) ;
#12968=AXIS2_PLACEMENT_3D ( 'NONE', #13854, #11508, #3449 ) ;
#12969=ORIENTED_EDGE ( 'NONE', *, *, #13980, .F. ) ;
#12970=CARTESIAN_POINT ( 'NONE',  ( 57.06275842387049835, -9.706953719245678514, -10.50000000000000000 ) ) ;
#12971=VECTOR ( 'NONE', #2775, 1000.000000000000000 ) ;
#12973=CIRCLE ( 'NONE', #6406, 3.000000000000002665 ) ;
#12974=VERTEX_POINT ( 'NONE', #1591 ) ;
#12975=CARTESIAN_POINT ( 'NONE',  ( 33.47282819776613394, -39.30189486418255740, 8.000000000000000000 ) ) ;
#12976=CARTESIAN_POINT ( 'NONE',  ( 89.12622059913255157, 37.21932736666302333, 10.49999999999999822 ) ) ;
#12977=CARTESIAN_POINT ( 'NONE',  ( -45.83364790889027773, 29.49928053175948506, 8.000000000000000000 ) ) ;
#12979=ORIENTED_EDGE ( 'NONE', *, *, #2586, .T. ) ;
#12983=EDGE_CURVE ( 'NONE', #1155, #2510, #4640, .T. ) ;
#12984=ORIENTED_EDGE ( 'NONE', *, *, #2258, .T. ) ;
#12985=AXIS2_PLACEMENT_3D ( 'NONE', #4224, #2998, #12273 ) ;
#12986=AXIS2_PLACEMENT_3D ( 'NONE', #11269, #6693, #3218 ) ;
#12987=CARTESIAN_POINT ( 'NONE',  ( -68.58935777509427112, 68.58935777509594800, -13.00000000000000178 ) ) ;
#12988=CIRCLE ( 'NONE', #4507, 60.50000000000000711 ) ;
#12989=EDGE_CURVE ( 'NONE', #6551, #13229, #4936, .T. ) ;
#12994=EDGE_CURVE ( 'NONE', #6180, #10678, #9706, .T. ) ;
#12995=AXIS2_PLACEMENT_3D ( 'NONE', #2733, #1521, #7349 ) ;
#12996=DIRECTION ( 'NONE',  ( 0.000000000000000000, 0.000000000000000000, -1.000000000000000000 ) ) ;
#12998=FACE_OUTER_BOUND ( 'NONE', #4694, .T. ) ;
#12999=FACE_OUTER_BOUND ( 'NONE', #13457, .T. ) ;
#13000=DIRECTION ( 'NONE',  ( 0.000000000000000000, 0.000000000000000000, -1.000000000000000000 ) ) ;
#13001=DIRECTION ( 'NONE',  ( 0.000000000000000000, 0.000000000000000000, 1.000000000000000000 ) ) ;
#13002=ADVANCED_FACE ( 'NONE', ( #13130 ), #14414, .T. ) ;
#13003=VERTEX_POINT ( 'NONE', #12002 ) ;
#13006=EDGE_LOOP ( 'NONE', ( #3557, #5864, #9161, #7741, #4535, #6641 ) ) ;
#13008=DIRECTION ( 'NONE',  ( 0.000000000000000000, 0.000000000000000000, 1.000000000000000000 ) ) ;
#13009=DIRECTION ( 'NONE',  ( 0.000000000000000000, 0.000000000000000000, -1.000000000000000000 ) ) ;
#13011=VERTEX_POINT ( 'NONE', #6204 ) ;
#13012=CIRCLE ( 'NONE', #165, 0.5000000000000004441 ) ;
#13013=CARTESIAN_POINT ( 'NONE',  ( 32.06294366074496338, -42.50536573064421475, -10.50000000000000000 ) ) ;
#13014=ORIENTED_EDGE ( 'NONE', *, *, #14273, .T. ) ;
#13015=CARTESIAN_POINT ( 'NONE',  ( 69.16568774265594755, -71.53347797788796925, -8.000000000000000000 ) ) ;
#13016=CARTESIAN_POINT ( 'NONE',  ( 0.000000000000000000, 0.000000000000000000, 8.000000000000000000 ) ) ;
#13017=DIRECTION ( 'NONE',  ( 1.000000000000000000, -3.498601968356585929E-15, 0.000000000000000000 ) ) ;
#13018=CARTESIAN_POINT ( 'NONE',  ( 0.000000000000000000, 0.000000000000000000, 8.000000000000000000 ) ) ;
#13019=CIRCLE ( 'NONE', #6450, 0.5000000000000004441 ) ;
#13021=VERTEX_POINT ( 'NONE', #6341 ) ;
#13022=AXIS2_PLACEMENT_3D ( 'NONE', #11170, #462, #9866 ) ;
#13023=DIRECTION ( 'NONE',  ( 1.000000000000000000, 0.000000000000000000, -0.000000000000000000 ) ) ;
#13027=EDGE_CURVE ( 'NONE', #1277, #9852, #2446, .T. ) ;
#13028=ORIENTED_EDGE ( 'NONE', *, *, #1289, .F. ) ;
#13029=ORIENTED_EDGE ( 'NONE', *, *, #10429, .F. ) ;
#13030=DIRECTION ( 'NONE',  ( 0.000000000000000000, 0.000000000000000000, 1.000000000000000000 ) ) ;
#13033=CARTESIAN_POINT ( 'NONE',  ( 29.49928053175901610, 45.83364790889059037, -8.000000000000000000 ) ) ;
#13034=CARTESIAN_POINT ( 'NONE',  ( -68.58935777509427112, 68.58935777509594800, 10.49999999999999822 ) ) ;
#13037=ORIENTED_EDGE ( 'NONE', *, *, #404, .F. ) ;
#13039=CARTESIAN_POINT ( 'NONE',  ( -33.48561063518626923, 47.21331623427104063, -13.00000000000000178 ) ) ;
#13040=PLANE ( 'NONE',  #11354 ) ;
#13042=EDGE_CURVE ( 'NONE', #5870, #12645, #2695, .T. ) ;
#13044=ORIENTED_EDGE ( 'NONE', *, *, #11143, .T. ) ;
#13045=AXIS2_PLACEMENT_3D ( 'NONE', #3256, #3330, #1060 ) ;
#13047=CARTESIAN_POINT ( 'NONE',  ( -30.43807145043584583, 39.66766701456190702, 8.000000000000000000 ) ) ;
#13048=ORIENTED_EDGE ( 'NONE', *, *, #6810, .T. ) ;
#13049=CARTESIAN_POINT ( 'NONE',  ( -38.26834323650965786, -92.38795325112840828, 8.000000000000000000 ) ) ;
#13050=CARTESIAN_POINT ( 'NONE',  ( -1.674280531759317459, 94.51066581171355097, -8.000000000000000000 ) ) ;
#13051=FACE_OUTER_BOUND ( 'NONE', #14942, .T. ) ;
#13052=ORIENTED_EDGE ( 'NONE', *, *, #5067, .T. ) ;
#13054=CIRCLE ( 'NONE', #9883, 50.00000000000000000 ) ;
#13055=DIRECTION ( 'NONE',  ( 1.000000000000000000, 0.000000000000000000, 0.000000000000000000 ) ) ;
#13056=ORIENTED_EDGE ( 'NONE', *, *, #1435, .F. ) ;
#13057=DIRECTION ( 'NONE',  ( 0.000000000000000000, 0.000000000000000000, 1.000000000000000000 ) ) ;
#13059=VERTEX_POINT ( 'NONE', #5154 ) ;
#13061=EDGE_CURVE ( 'NONE', #2546, #8947, #4093, .T. ) ;
#13062=DIRECTION ( 'NONE',  ( 0.000000000000000000, 0.000000000000000000, 1.000000000000000000 ) ) ;
#13064=ORIENTED_EDGE ( 'NONE', *, *, #6612, .T. ) ;
#13065=DIRECTION ( 'NONE',  ( 0.000000000000000000, 0.000000000000000000, 1.000000000000000000 ) ) ;
#13066=EDGE_CURVE ( 'NONE', #7929, #11386, #10446, .T. ) ;
#13068=CARTESIAN_POINT ( 'NONE',  ( 40.12029293941316155, -89.61631465359504034, -8.000000000000000000 ) ) ;
#13069=DIRECTION ( 'NONE',  ( -0.000000000000000000, -0.000000000000000000, -1.000000000000000000 ) ) ;
#13070=CARTESIAN_POINT ( 'NONE',  ( 15.88467684210547226, -49.11971303961683333, 8.000000000000000000 ) ) ;
#13071=ORIENTED_EDGE ( 'NONE', *, *, #2233, .T. ) ;
#13072=ADVANCED_FACE ( 'NONE', ( #13499 ), #3252, .T. ) ;
#13073=CARTESIAN_POINT ( 'NONE',  ( -45.89934640057513349, 26.50000000000019540, 8.000000000000000000 ) ) ;
#13075=FACE_OUTER_BOUND ( 'NONE', #8311, .T. ) ;
#13076=CIRCLE ( 'NONE', #7969, 0.5000000000000004441 ) ;
#13077=CARTESIAN_POINT ( 'NONE',  ( -37.02125851216292318, 90.10640870805768543, -10.50000000000000000 ) ) ;
#13078=DIRECTION ( 'NONE',  ( -1.000000000000000000, 0.000000000000000000, 0.000000000000000000 ) ) ;
#13079=ADVANCED_FACE ( 'NONE', ( #830 ), #4397, .T. ) ;
#13082=ORIENTED_EDGE ( 'NONE', *, *, #4723, .F. ) ;
#13083=DIRECTION ( 'NONE',  ( 1.000000000000000000, 0.000000000000000000, 0.000000000000000000 ) ) ;
#13085=EDGE_LOOP ( 'NONE', ( #2865, #11609, #7036, #11191, #14560, #11448, #3546, #13265, #10458 ) ) ;
#13087=FACE_OUTER_BOUND ( 'NONE', #7480, .T. ) ;
#13090=CARTESIAN_POINT ( 'NONE',  ( -48.19406879332065330, -13.71740939043347041, -8.000000000000000000 ) ) ;
#13091=DIRECTION ( 'NONE',  ( 1.000000000000000000, 0.000000000000000000, 0.000000000000000000 ) ) ;
#13092=VERTEX_POINT ( 'NONE', #14793 ) ;
#13093=DIRECTION ( 'NONE',  ( -1.000000000000000000, 6.927231897346039366E-14, 0.000000000000000000 ) ) ;
#13094=DIRECTION ( 'NONE',  ( 1.000000000000000000, 0.000000000000000000, 0.000000000000000000 ) ) ;
#13095=DIRECTION ( 'NONE',  ( -1.000000000000000000, 0.000000000000000000, 0.000000000000000000 ) ) ;
#13099=VECTOR ( 'NONE', #12308, 1000.000000000000000 ) ;
#13100=ORIENTED_EDGE ( 'NONE', *, *, #10567, .F. ) ;
#13102=ORIENTED_EDGE ( 'NONE', *, *, #9961, .T. ) ;
#13104=VERTEX_POINT ( 'NONE', #7873 ) ;
#13105=VECTOR ( 'NONE', #6683, 1000.000000000000000 ) ;
#13106=DIRECTION ( 'NONE',  ( -0.000000000000000000, -0.000000000000000000, -1.000000000000000000 ) ) ;
#13109=AXIS2_PLACEMENT_3D ( 'NONE', #6278, #535, #9561 ) ;
#13110=ORIENTED_EDGE ( 'NONE', *, *, #13690, .F. ) ;
#13111=EDGE_LOOP ( 'NONE', ( #14478, #3685, #9800, #8547, #5485, #14751, #12543, #5995, #11380, #11360 ) ) ;
#13113=CARTESIAN_POINT ( 'NONE',  ( -12.86891638962156215, 56.43380494353993271, -10.50000000000000000 ) ) ;
#13114=DIRECTION ( 'NONE',  ( -1.000000000000000000, 0.000000000000000000, 0.000000000000000000 ) ) ;
#13117=AXIS2_PLACEMENT_3D ( 'NONE', #10860, #2595, #13149 ) ;
#13118=VECTOR ( 'NONE', #7186, 1000.000000000000000 ) ;
#13119=VERTEX_POINT ( 'NONE', #3103 ) ;
#13120=CARTESIAN_POINT ( 'NONE',  ( 9.706953719245472456, 57.06275842387054098, -13.00000000000000178 ) ) ;
#13121=CIRCLE ( 'NONE', #8500, 53.55662432702593634 ) ;
#13122=VERTEX_POINT ( 'NONE', #13565 ) ;
#13123=AXIS2_PLACEMENT_3D ( 'NONE', #6127, #11076, #5454 ) ;
#13124=DIRECTION ( 'NONE',  ( 0.000000000000000000, 0.000000000000000000, 1.000000000000000000 ) ) ;
#13125=EDGE_CURVE ( 'NONE', #4787, #14448, #1010, .T. ) ;
#13127=EDGE_CURVE ( 'NONE', #6408, #5997, #4878, .T. ) ;
#13128=EDGE_CURVE ( 'NONE', #3028, #7285, #3030, .T. ) ;
#13129=ORIENTED_EDGE ( 'NONE', *, *, #4818, .T. ) ;
#13130=FACE_OUTER_BOUND ( 'NONE', #5361, .T. ) ;
#13131=CIRCLE ( 'NONE', #14103, 59.50000000000000000 ) ;
#13133=VERTEX_POINT ( 'NONE', #12441 ) ;
#13134=CIRCLE ( 'NONE', #33, 3.000000000000002665 ) ;
#13135=DIRECTION ( 'NONE',  ( -0.000000000000000000, -0.000000000000000000, 1.000000000000000000 ) ) ;
#13136=CIRCLE ( 'NONE', #3684, 3.000000000000002665 ) ;
#13137=VERTEX_POINT ( 'NONE', #11147 ) ;
#13138=ORIENTED_EDGE ( 'NONE', *, *, #2793, .F. ) ;
#13140=VECTOR ( 'NONE', #5493, 1000.000000000000000 ) ;
#13141=VERTEX_POINT ( 'NONE', #5527 ) ;
#13143=CIRCLE ( 'NONE', #6579, 3.000000000000002665 ) ;
#13144=DIRECTION ( 'NONE',  ( 0.000000000000000000, 0.000000000000000000, 1.000000000000000000 ) ) ;
#13145=FACE_OUTER_BOUND ( 'NONE', #14717, .T. ) ;
#13147=DIRECTION ( 'NONE',  ( 1.000000000000000000, 0.000000000000000000, 0.000000000000000000 ) ) ;
#13148=ORIENTED_EDGE ( 'NONE', *, *, #14281, .F. ) ;
#13149=DIRECTION ( 'NONE',  ( -1.000000000000000000, 0.000000000000000000, 0.000000000000000000 ) ) ;
#13151=ORIENTED_EDGE ( 'NONE', *, *, #7025, .T. ) ;
#13152=EDGE_CURVE ( 'NONE', #9152, #5654, #2035, .T. ) ;
#13154=CARTESIAN_POINT ( 'NONE',  ( -68.58935777509427112, 68.58935777509594800, 8.000000000000000000 ) ) ;
#13155=CIRCLE ( 'NONE', #7569, 60.50000000000000000 ) ;
#13157=CYLINDRICAL_SURFACE ( 'NONE', #13673, 3.000000000000002665 ) ;
#13159=CARTESIAN_POINT ( 'NONE',  ( -19.68583958711381143, -30.74264578624812927, -28.00000000000000000 ) ) ;
#13160=VERTEX_POINT ( 'NONE', #12519 ) ;
#13161=CIRCLE ( 'NONE', #6339, 60.50000000000000000 ) ;
#13162=DIRECTION ( 'NONE',  ( -1.000000000000000000, 0.000000000000000000, 0.000000000000000000 ) ) ;
#13163=DIRECTION ( 'NONE',  ( -0.000000000000000000, -0.000000000000000000, -1.000000000000000000 ) ) ;
#13166=CARTESIAN_POINT ( 'NONE',  ( 68.58935777509475429, -68.58935777509547904, 10.49999999999999822 ) ) ;
#13167=CARTESIAN_POINT ( 'NONE',  ( -26.49999999999971578, -45.89934640057541060, 8.000000000000000000 ) ) ;
#13168=EDGE_CURVE ( 'NONE', #10287, #11546, #264, .T. ) ;
#13169=ORIENTED_EDGE ( 'NONE', *, *, #10429, .T. ) ;
#13170=ORIENTED_EDGE ( 'NONE', *, *, #5632, .T. ) ;
#13171=ADVANCED_FACE ( 'NONE', ( #13651, #4250, #7652, #11229, #2109, #7798, #8786 ), #12216, .F. ) ;
#13172=CARTESIAN_POINT ( 'NONE',  ( -32.26435573746199736, 42.04772703543562073, -8.000000000000000000 ) ) ;
#13173=CARTESIAN_POINT ( 'NONE',  ( -86.67575032682103142, -37.71449950291016506, -13.00000000000000178 ) ) ;
#13175=DIRECTION ( 'NONE',  ( -1.000000000000000000, 0.000000000000000000, 0.000000000000000000 ) ) ;
#13178=VERTEX_POINT ( 'NONE', #6651 ) ;
#13180=CARTESIAN_POINT ( 'NONE',  ( -19.68583958711381143, -30.74264578624812927, -25.50000000000000355 ) ) ;
#13181=EDGE_LOOP ( 'NONE', ( #8320, #13138, #12885, #14299, #4768, #742 ) ) ;
#13183=AXIS2_PLACEMENT_3D ( 'NONE', #4043, #6363, #11018 ) ;
#13184=DIRECTION ( 'NONE',  ( 0.000000000000000000, 0.000000000000000000, 1.000000000000000000 ) ) ;
#13185=DIRECTION ( 'NONE',  ( 1.000000000000000000, 0.000000000000000000, 0.000000000000000000 ) ) ;
#13188=ORIENTED_EDGE ( 'NONE', *, *, #11021, .F. ) ;
#13191=DIRECTION ( 'NONE',  ( 0.000000000000000000, 0.000000000000000000, 1.000000000000000000 ) ) ;
#13192=DIRECTION ( 'NONE',  ( -0.000000000000000000, -0.000000000000000000, 1.000000000000000000 ) ) ;
#13194=LINE ( 'NONE', #3790, #8080 ) ;
#13195=ORIENTED_EDGE ( 'NONE', *, *, #700, .T. ) ;
#13196=ORIENTED_EDGE ( 'NONE', *, *, #4028, .T. ) ;
#13201=CIRCLE ( 'NONE', #3502, 3.000000000000002665 ) ;
#13203=AXIS2_PLACEMENT_3D ( 'NONE', #1775, #4290, #14374 ) ;
#13205=CYLINDRICAL_SURFACE ( 'NONE', #3172, 56.99999999999999289 ) ;
#13206=ORIENTED_EDGE ( 'NONE', *, *, #5474, .F. ) ;
#13209=ORIENTED_EDGE ( 'NONE', *, *, #13306, .F. ) ;
#13210=DIRECTION ( 'NONE',  ( 0.000000000000000000, 0.000000000000000000, 1.000000000000000000 ) ) ;
#13211=AXIS2_PLACEMENT_3D ( 'NONE', #4840, #14257, #7250 ) ;
#13217=DIRECTION ( 'NONE',  ( 0.000000000000000000, 0.000000000000000000, -1.000000000000000000 ) ) ;
#13218=ADVANCED_FACE ( 'NONE', ( #7315 ), #3841, .T. ) ;
#13220=FACE_OUTER_BOUND ( 'NONE', #5713, .T. ) ;
#13221=AXIS2_PLACEMENT_3D ( 'NONE', #14746, #12466, #3278 ) ;
#13222=DIRECTION ( 'NONE',  ( 1.000000000000000000, 0.000000000000000000, 0.000000000000000000 ) ) ;
#13223=DIRECTION ( 'NONE',  ( 1.000000000000000000, 0.000000000000000000, 0.000000000000000000 ) ) ;
#13224=CARTESIAN_POINT ( 'NONE',  ( -70.71067811865385977, 70.71067811865565034, -8.000000000000000000 ) ) ;
#13226=FACE_OUTER_BOUND ( 'NONE', #12521, .T. ) ;
#13227=VERTEX_POINT ( 'NONE', #13253 ) ;
#13228=DIRECTION ( 'NONE',  ( 0.000000000000000000, 0.000000000000000000, 1.000000000000000000 ) ) ;
#13229=VERTEX_POINT ( 'NONE', #10820 ) ;
#13230=EDGE_CURVE ( 'NONE', #2908, #3918, #998, .T. ) ;
#13231=DIRECTION ( 'NONE',  ( -1.000000000000000000, 0.000000000000000000, 0.000000000000000000 ) ) ;
#13233=ORIENTED_EDGE ( 'NONE', *, *, #8305, .F. ) ;
#13235=EDGE_CURVE ( 'NONE', #9892, #3062, #12879, .T. ) ;
#13236=AXIS2_PLACEMENT_3D ( 'NONE', #2723, #6124, #8415 ) ;
#13239=CARTESIAN_POINT ( 'NONE',  ( 2.449293598294700991E-16, -97.00000000000000000, -10.50000000000000000 ) ) ;
#13242=CARTESIAN_POINT ( 'NONE',  ( 0.000000000000000000, 0.000000000000000000, -8.000000000000000000 ) ) ;
#13243=CARTESIAN_POINT ( 'NONE',  ( -32.26435573746199736, 42.04772703543562073, 10.49999999999999822 ) ) ;
#13244=CARTESIAN_POINT ( 'NONE',  ( 48.29629131445336299, 12.94095225512623060, -8.000000000000000000 ) ) ;
#13245=CARTESIAN_POINT ( 'NONE',  ( -30.80502811811232888, -49.00442420935981147, -10.50000000000000000 ) ) ;
#13247=DIRECTION ( 'NONE',  ( -0.000000000000000000, -0.000000000000000000, 1.000000000000000000 ) ) ;
#13250=DIRECTION ( 'NONE',  ( 0.000000000000000000, 0.000000000000000000, -1.000000000000000000 ) ) ;
#13251=AXIS2_PLACEMENT_3D ( 'NONE', #13172, #14157, #3766 ) ;
#13252=ORIENTED_EDGE ( 'NONE', *, *, #3041, .T. ) ;
#13253=CARTESIAN_POINT ( 'NONE',  ( -68.49330278050074128, 68.09867107463051639, 10.49999999999999822 ) ) ;
#13254=EDGE_CURVE ( 'NONE', #5756, #836, #7043, .T. ) ;
#13257=CARTESIAN_POINT ( 'NONE',  ( 29.51438936481373077, 47.21331623427104063, -13.00000000000000178 ) ) ;
#13258=CARTESIAN_POINT ( 'NONE',  ( -45.91029614918924295, 26.00011991137363765, -10.50000000000000000 ) ) ;
#13259=EDGE_CURVE ( 'NONE', #4441, #1935, #8737, .T. ) ;
#13260=DIRECTION ( 'NONE',  ( 1.000000000000000000, 0.000000000000000000, 0.000000000000000000 ) ) ;
#13264=CIRCLE ( 'NONE', #12777, 52.50000000000000711 ) ;
#13265=ORIENTED_EDGE ( 'NONE', *, *, #6151, .T. ) ;
#13267=DIRECTION ( 'NONE',  ( 1.000000000000000000, 0.000000000000000000, 0.000000000000000000 ) ) ;
#13268=LINE ( 'NONE', #7328, #606 ) ;
#13269=DIRECTION ( 'NONE',  ( -1.000000000000000000, 0.000000000000000000, 0.000000000000000000 ) ) ;
#13271=ORIENTED_EDGE ( 'NONE', *, *, #10747, .T. ) ;
#13272=PLANE ( 'NONE',  #9558 ) ;
#13273=ORIENTED_EDGE ( 'NONE', *, *, #13397, .F. ) ;
#13274=EDGE_CURVE ( 'NONE', #7460, #7416, #4154, .T. ) ;
#13275=CARTESIAN_POINT ( 'NONE',  ( 23.51438936481372366, 47.21331623427104063, -8.000000000000000000 ) ) ;
#13277=DIRECTION ( 'NONE',  ( 1.000000000000000000, 0.000000000000000000, 0.000000000000000000 ) ) ;
#13278=CARTESIAN_POINT ( 'NONE',  ( -50.00000000000000000, 0.000000000000000000, 13.00000000000000178 ) ) ;
#13279=VERTEX_POINT ( 'NONE', #5125 ) ;
#13280=FACE_OUTER_BOUND ( 'NONE', #13895, .T. ) ;
#13281=ORIENTED_EDGE ( 'NONE', *, *, #3887, .T. ) ;
#13282=EDGE_LOOP ( 'NONE', ( #7950, #5366, #14287, #12984 ) ) ;
#13283=DIRECTION ( 'NONE',  ( 0.000000000000000000, 0.000000000000000000, -1.000000000000000000 ) ) ;
#13285=CARTESIAN_POINT ( 'NONE',  ( -43.30127018922183169, 25.00000000000018474, 8.000000000000000000 ) ) ;
#13286=DIRECTION ( 'NONE',  ( 0.000000000000000000, 0.000000000000000000, -1.000000000000000000 ) ) ;
#13288=DIRECTION ( 'NONE',  ( 1.000000000000000000, 0.000000000000000000, 0.000000000000000000 ) ) ;
#13292=DIRECTION ( 'NONE',  ( 0.000000000000000000, 0.000000000000000000, 1.000000000000000000 ) ) ;
#13293=DIRECTION ( 'NONE',  ( 0.000000000000000000, 0.000000000000000000, -1.000000000000000000 ) ) ;
#13294=CARTESIAN_POINT ( 'NONE',  ( -22.33583958711380646, -30.74264578624812927, -28.00000000000000000 ) ) ;
#13295=VERTEX_POINT ( 'NONE', #13180 ) ;
#13296=FILL_AREA_STYLE ('',( #2975 ) ) ;
#13297=ORIENTED_EDGE ( 'NONE', *, *, #9314, .F. ) ;
#13299=ORIENTED_EDGE ( 'NONE', *, *, #12806, .F. ) ;
#13300=DIRECTION ( 'NONE',  ( -1.000000000000000000, 0.000000000000000000, 0.000000000000000000 ) ) ;
#13301=ORIENTED_EDGE ( 'NONE', *, *, #4262, .F. ) ;
#13302=CARTESIAN_POINT ( 'NONE',  ( 12.86891638962116247, -56.43380494354001087, -10.50000000000000000 ) ) ;
#13303=DIRECTION ( 'NONE',  ( -0.000000000000000000, -0.000000000000000000, -1.000000000000000000 ) ) ;
#13304=DIRECTION ( 'NONE',  ( 1.000000000000000000, 0.000000000000000000, 0.000000000000000000 ) ) ;
#13306=EDGE_CURVE ( 'NONE', #1631, #8562, #8019, .T. ) ;
#13307=CARTESIAN_POINT ( 'NONE',  ( 0.000000000000000000, 0.000000000000000000, 8.000000000000000000 ) ) ;
#13309=EDGE_CURVE ( 'NONE', #6495, #9289, #13136, .T. ) ;
#13310=DIRECTION ( 'NONE',  ( 1.000000000000000000, 0.000000000000000000, 0.000000000000000000 ) ) ;
#13311=ORIENTED_EDGE ( 'NONE', *, *, #6107, .F. ) ;
#13312=DIRECTION ( 'NONE',  ( 0.000000000000000000, 0.000000000000000000, 1.000000000000000000 ) ) ;
#13313=CARTESIAN_POINT ( 'NONE',  ( 14.07862063237891981, -50.84834283436993729, -13.00000000000000178 ) ) ;
#13315=ORIENTED_EDGE ( 'NONE', *, *, #7634, .F. ) ;
#13319=CARTESIAN_POINT ( 'NONE',  ( -94.51066581171356518, -1.674280531758327140, 8.000000000000000000 ) ) ;
#13320=DIRECTION ( 'NONE',  ( 1.000000000000000000, 0.000000000000000000, 0.000000000000000000 ) ) ;
#13321=CARTESIAN_POINT ( 'NONE',  ( -69.16568774265545017, 71.53347797788843820, -8.000000000000000000 ) ) ;
#13322=DIRECTION ( 'NONE',  ( 0.000000000000000000, 0.000000000000000000, 1.000000000000000000 ) ) ;
#13324=ORIENTED_EDGE ( 'NONE', *, *, #5016, .F. ) ;
#13325=ORIENTED_EDGE ( 'NONE', *, *, #7198, .F. ) ;
#13326=CIRCLE ( 'NONE', #8708, 3.000000000000002665 ) ;
#13328=CARTESIAN_POINT ( 'NONE',  ( 2.449293598294700991E-16, -97.00000000000000000, 10.49999999999999822 ) ) ;
#13329=VECTOR ( 'NONE', #2575, 1000.000000000000000 ) ;
#13330=CARTESIAN_POINT ( 'NONE',  ( 57.06275842387049835, -9.706953719245678514, -13.00000000000000178 ) ) ;
#13332=VECTOR ( 'NONE', #3115, 1000.000000000000000 ) ;
#13335=ADVANCED_FACE ( 'NONE', ( #5349 ), #6472, .F. ) ;
#13336=ORIENTED_EDGE ( 'NONE', *, *, #14648, .T. ) ;
#13337=VERTEX_POINT ( 'NONE', #5011 ) ;
#13339=CIRCLE ( 'NONE', #8718, 2.649999999999992806 ) ;
#13340=CIRCLE ( 'NONE', #2188, 60.50000000000000000 ) ;
#13341=DIRECTION ( 'NONE',  ( 1.000000000000000000, 0.000000000000000000, 0.000000000000000000 ) ) ;
#13342=VECTOR ( 'NONE', #1469, 1000.000000000000000 ) ;
#13345=VERTEX_POINT ( 'NONE', #11277 ) ;
#13346=CARTESIAN_POINT ( 'NONE',  ( 9.714003807514266953, 53.63365512954683112, -13.00000000000000178 ) ) ;
#13347=CARTESIAN_POINT ( 'NONE',  ( 51.19406879332056093, 13.71740939043382745, 8.000000000000000000 ) ) ;
#13349=CARTESIAN_POINT ( 'NONE',  ( -42.04772703543551415, -32.26435573746212526, 8.000000000000000000 ) ) ;
#13351=AXIS2_PLACEMENT_3D ( 'NONE', #4791, #13065, #2813 ) ;
#13352=EDGE_CURVE ( 'NONE', #11311, #12963, #1972, .T. ) ;
#13353=ORIENTED_EDGE ( 'NONE', *, *, #539, .T. ) ;
#13354=VECTOR ( 'NONE', #3512, 1000.000000000000000 ) ;
#13355=CIRCLE ( 'NONE', #263, 100.0000000000000000 ) ;
#13357=ORIENTED_EDGE ( 'NONE', *, *, #6088, .T. ) ;
#13358=CARTESIAN_POINT ( 'NONE',  ( 45.89934640057532533, -26.49999999999987566, -10.50000000000000000 ) ) ;
#13359=FACE_OUTER_BOUND ( 'NONE', #13834, .T. ) ;
#13360=EDGE_CURVE ( 'NONE', #12781, #4070, #12410, .T. ) ;
#13361=CARTESIAN_POINT ( 'NONE',  ( 0.000000000000000000, 0.000000000000000000, -8.000000000000000000 ) ) ;
#13362=CARTESIAN_POINT ( 'NONE',  ( 89.61631465359491244, 37.12029293941346708, -13.00000000000000178 ) ) ;
#13363=DIRECTION ( 'NONE',  ( 1.000000000000000000, -4.440892098500626162E-15, 0.000000000000000000 ) ) ;
#13364=AXIS2_PLACEMENT_3D ( 'NONE', #14023, #11749, #11677 ) ;
#13365=DIRECTION ( 'NONE',  ( 0.000000000000000000, 0.000000000000000000, 1.000000000000000000 ) ) ;
#13366=AXIS2_PLACEMENT_3D ( 'NONE', #6850, #11513, #5784 ) ;
#13367=ORIENTED_EDGE ( 'NONE', *, *, #11829, .F. ) ;
#13368=DIRECTION ( 'NONE',  ( -0.000000000000000000, -0.000000000000000000, -1.000000000000000000 ) ) ;
#13371=CARTESIAN_POINT ( 'NONE',  ( -2.449293598294708880E-16, 38.00000000000000000, -25.50000000000000355 ) ) ;
#13372=CARTESIAN_POINT ( 'NONE',  ( 32.06294366074496338, -42.50536573064421475, 10.49999999999999822 ) ) ;
#13373=CIRCLE ( 'NONE', #12401, 53.55662432702593634 ) ;
#13376=DIRECTION ( 'NONE',  ( 0.000000000000000000, 0.000000000000000000, -1.000000000000000000 ) ) ;
#13377=ORIENTED_EDGE ( 'NONE', *, *, #14050, .T. ) ;
#13378=CARTESIAN_POINT ( 'NONE',  ( -89.61631465359519666, -37.12029293941281338, 8.000000000000000000 ) ) ;
#13379=ORIENTED_EDGE ( 'NONE', *, *, #13397, .T. ) ;
#13382=CYLINDRICAL_SURFACE ( 'NONE', #7329, 59.50000000000000000 ) ;
#13384=CYLINDRICAL_SURFACE ( 'NONE', #5346, 2.649999999999992806 ) ;
#13385=CARTESIAN_POINT ( 'NONE',  ( 68.68541276968825571, -69.08004447556089644, -10.50000000000000000 ) ) ;
#13386=ORIENTED_EDGE ( 'NONE', *, *, #13066, .T. ) ;
#13388=ORIENTED_EDGE ( 'NONE', *, *, #10332, .F. ) ;
#13389=AXIS2_PLACEMENT_3D ( 'NONE', #7845, #2088, #3153 ) ;
#13391=CARTESIAN_POINT ( 'NONE',  ( -32.26435573746199736, 42.04772703543562073, -13.00000000000000178 ) ) ;
#13393=EDGE_CURVE ( 'NONE', #13059, #5144, #9244, .T. ) ;
#13394=CIRCLE ( 'NONE', #6838, 3.000000000000002665 ) ;
#13395=ORIENTED_EDGE ( 'NONE', *, *, #1154, .F. ) ;
#13397=EDGE_CURVE ( 'NONE', #2518, #7149, #6568, .T. ) ;
#13399=ORIENTED_EDGE ( 'NONE', *, *, #12875, .T. ) ;
#13400=VECTOR ( 'NONE', #12717, 1000.000000000000000 ) ;
#13401=CARTESIAN_POINT ( 'NONE',  ( 26.49999999999971578, 45.89934640057541060, -13.00000000000000178 ) ) ;
#13402=CARTESIAN_POINT ( 'NONE',  ( -45.89934640057513349, 26.50000000000019540, -8.000000000000000000 ) ) ;
#13404=DIRECTION ( 'NONE',  ( 0.000000000000000000, 0.000000000000000000, -1.000000000000000000 ) ) ;
#13408=VERTEX_POINT ( 'NONE', #2150 ) ;
#13409=CIRCLE ( 'NONE', #1297, 63.00000000000000000 ) ;
#13410=DIRECTION ( 'NONE',  ( -0.000000000000000000, -0.000000000000000000, 1.000000000000000000 ) ) ;
#13411=DIRECTION ( 'NONE',  ( 0.000000000000000000, 0.000000000000000000, 1.000000000000000000 ) ) ;
#13413=CARTESIAN_POINT ( 'NONE',  ( 30.80502811811196295, 49.00442420936003174, 8.000000000000000000 ) ) ;
#13417=EDGE_CURVE ( 'NONE', #11178, #4704, #14106, .T. ) ;
#13418=VERTEX_POINT ( 'NONE', #14845 ) ;
#13419=CIRCLE ( 'NONE', #328, 59.50000000000000000 ) ;
#13420=FACE_OUTER_BOUND ( 'NONE', #2251, .T. ) ;
#13421=DIRECTION ( 'NONE',  ( -1.000000000000000000, 0.000000000000000000, 0.000000000000000000 ) ) ;
#13422=CARTESIAN_POINT ( 'NONE',  ( -31.05588327715806329, 44.79355920668842828, -13.00000000000000178 ) ) ;
#13423=EDGE_LOOP ( 'NONE', ( #6959, #8701, #10134, #13315 ) ) ;
#13424=AXIS2_PLACEMENT_3D ( 'NONE', #4374, #5436, #11128 ) ;
#13425=DIRECTION ( 'NONE',  ( 1.000000000000000000, 0.000000000000000000, 0.000000000000000000 ) ) ;
#13428=CARTESIAN_POINT ( 'NONE',  ( 0.000000000000000000, 0.000000000000000000, 8.000000000000000000 ) ) ;
#13431=CIRCLE ( 'NONE', #14904, 0.5000000000000004441 ) ;
#13434=AXIS2_PLACEMENT_3D ( 'NONE', #6532, #12177, #7687 ) ;
#13435=DIRECTION ( 'NONE',  ( 1.000000000000000000, 0.000000000000000000, 0.000000000000000000 ) ) ;
#13436=ADVANCED_FACE ( 'NONE', ( #9054 ), #12339, .F. ) ;
#13439=CARTESIAN_POINT ( 'NONE',  ( 45.89934640057532533, -26.49999999999987566, -8.000000000000000000 ) ) ;
#13440=CARTESIAN_POINT ( 'NONE',  ( 0.000000000000000000, 0.000000000000000000, 8.000000000000000000 ) ) ;
#13442=ORIENTED_EDGE ( 'NONE', *, *, #11687, .F. ) ;
#13444=AXIS2_PLACEMENT_3D ( 'NONE', #3687, #9434, #5733 ) ;
#13446=AXIS2_PLACEMENT_3D ( 'NONE', #6416, #11071, #13341 ) ;
#13447=EDGE_CURVE ( 'NONE', #3890, #8922, #4167, .T. ) ;
#13450=ORIENTED_EDGE ( 'NONE', *, *, #10791, .F. ) ;
#13451=DIRECTION ( 'NONE',  ( 1.000000000000000000, 0.000000000000000000, 0.000000000000000000 ) ) ;
#13453=DIRECTION ( 'NONE',  ( -1.000000000000000000, 0.000000000000000000, 0.000000000000000000 ) ) ;
#13454=ORIENTED_EDGE ( 'NONE', *, *, #1248, .T. ) ;
#13456=CYLINDRICAL_SURFACE ( 'NONE', #6538, 0.5000000000000004441 ) ;
#13457=EDGE_LOOP ( 'NONE', ( #12744, #10171, #14239, #10849, #12142, #14882 ) ) ;
#13458=EDGE_CURVE ( 'NONE', #2743, #8664, #12406, .T. ) ;
#13459=ORIENTED_EDGE ( 'NONE', *, *, #11143, .F. ) ;
#13460=DIRECTION ( 'NONE',  ( 1.000000000000000000, 0.000000000000000000, 0.000000000000000000 ) ) ;
#13462=DIRECTION ( 'NONE',  ( 0.000000000000000000, 0.000000000000000000, 1.000000000000000000 ) ) ;
#13464=DIRECTION ( 'NONE',  ( 0.000000000000000000, 0.000000000000000000, 1.000000000000000000 ) ) ;
#13465=CARTESIAN_POINT ( 'NONE',  ( -39.04772703543551415, -32.26435573746212526, 8.000000000000000000 ) ) ;
#13466=AXIS2_PLACEMENT_3D ( 'NONE', #10258, #6906, #5548 ) ;
#13467=ORIENTED_EDGE ( 'NONE', *, *, #3411, .F. ) ;
#13472=ORIENTED_EDGE ( 'NONE', *, *, #14506, .T. ) ;
#13473=AXIS2_PLACEMENT_3D ( 'NONE', #8540, #2783, #6250 ) ;
#13476=CYLINDRICAL_SURFACE ( 'NONE', #5222, 0.5000000000000004441 ) ;
#13478=DIRECTION ( 'NONE',  ( 0.000000000000000000, 0.000000000000000000, 1.000000000000000000 ) ) ;
#13479=DIRECTION ( 'NONE',  ( 0.000000000000000000, 0.000000000000000000, -1.000000000000000000 ) ) ;
#13481=ORIENTED_EDGE ( 'NONE', *, *, #12291, .F. ) ;
#13482=ORIENTED_EDGE ( 'NONE', *, *, #1008, .F. ) ;
#13483=ADVANCED_FACE ( 'NONE', ( #100 ), #5720, .T. ) ;
#13484=AXIS2_PLACEMENT_3D ( 'NONE', #12946, #8226, #8529 ) ;
#13485=CARTESIAN_POINT ( 'NONE',  ( 30.80502811811196295, 49.00442420936003174, -13.00000000000000178 ) ) ;
#13488=CARTESIAN_POINT ( 'NONE',  ( -30.80502811811232888, -49.00442420935981147, 8.000000000000000000 ) ) ;
#13490=VERTEX_POINT ( 'NONE', #6007 ) ;
#13491=ORIENTED_EDGE ( 'NONE', *, *, #7882, .T. ) ;
#13492=AXIS2_PLACEMENT_3D ( 'NONE', #6950, #4614, #1054 ) ;
#13494=DIRECTION ( 'NONE',  ( 1.000000000000000000, 0.000000000000000000, 0.000000000000000000 ) ) ;
#13496=PLANE ( 'NONE',  #7362 ) ;
#13497=EDGE_CURVE ( 'NONE', #6488, #9994, #2704, .T. ) ;
#13498=CARTESIAN_POINT ( 'NONE',  ( -68.08935777509570642, -68.58935777509452691, -10.50000000000000000 ) ) ;
#13499=FACE_OUTER_BOUND ( 'NONE', #1956, .T. ) ;
#13502=ADVANCED_FACE ( 'NONE', ( #11804 ), #6925, .F. ) ;
#13503=ADVANCED_FACE ( 'NONE', ( #2448 ), #7067, .T. ) ;
#13504=DIRECTION ( 'NONE',  ( 0.000000000000000000, 0.000000000000000000, -1.000000000000000000 ) ) ;
#13505=ORIENTED_EDGE ( 'NONE', *, *, #2771, .F. ) ;
#13506=ORIENTED_EDGE ( 'NONE', *, *, #11366, .T. ) ;
#13507=CARTESIAN_POINT ( 'NONE',  ( 20.00000000000000000, 2.449293598294706513E-15, -25.50000000000000355 ) ) ;
#13508=DIRECTION ( 'NONE',  ( -0.000000000000000000, -0.000000000000000000, -1.000000000000000000 ) ) ;
#13509=CARTESIAN_POINT ( 'NONE',  ( -49.11971303961688307, -15.88467684210530528, 8.000000000000000000 ) ) ;
#13511=DIRECTION ( 'NONE',  ( 1.000000000000000000, 0.000000000000000000, 0.000000000000000000 ) ) ;
#13515=DIRECTION ( 'NONE',  ( -1.000000000000000000, 0.000000000000000000, 0.000000000000000000 ) ) ;
#13516=CARTESIAN_POINT ( 'NONE',  ( 0.000000000000000000, 0.000000000000000000, 8.000000000000000000 ) ) ;
#13518=ORIENTED_EDGE ( 'NONE', *, *, #2780, .F. ) ;
#13520=ORIENTED_EDGE ( 'NONE', *, *, #5699, .F. ) ;
#13522=ADVANCED_FACE ( 'NONE', ( #10578 ), #10354, .F. ) ;
#13523=VERTEX_POINT ( 'NONE', #176 ) ;
#13524=FACE_OUTER_BOUND ( 'NONE', #11431, .T. ) ;
#13525=ORIENTED_EDGE ( 'NONE', *, *, #5082, .T. ) ;
#13526=CARTESIAN_POINT ( 'NONE',  ( -2.449293598294700991E-16, 97.00000000000000000, 10.49999999999999822 ) ) ;
#13527=CARTESIAN_POINT ( 'NONE',  ( 90.10640870805727332, 37.02125851216391794, 10.49999999999999822 ) ) ;
#13528=CARTESIAN_POINT ( 'NONE',  ( -9.706953719245875689, -57.06275842387046993, 8.000000000000000000 ) ) ;
#13529=ADVANCED_FACE ( 'NONE', ( #14070 ), #10641, .F. ) ;
#13530=FACE_OUTER_BOUND ( 'NONE', #6849, .T. ) ;
#13532=ORIENTED_EDGE ( 'NONE', *, *, #4139, .T. ) ;
#13534=ORIENTED_EDGE ( 'NONE', *, *, #10723, .T. ) ;
#13535=CARTESIAN_POINT ( 'NONE',  ( 90.11631465359491244, 37.12029293941346708, -13.00000000000000178 ) ) ;
#13537=EDGE_CURVE ( 'NONE', #1631, #2976, #5131, .T. ) ;
#13538=EDGE_CURVE ( 'NONE', #12429, #12179, #1741, .T. ) ;
#13539=DIRECTION ( 'NONE',  ( 0.000000000000000000, 0.000000000000000000, 1.000000000000000000 ) ) ;
#13540=DIRECTION ( 'NONE',  ( -1.000000000000000000, 0.000000000000000000, 0.000000000000000000 ) ) ;
#13541=ORIENTED_EDGE ( 'NONE', *, *, #8566, .F. ) ;
#13543=ORIENTED_EDGE ( 'NONE', *, *, #8446, .T. ) ;
#13544=CYLINDRICAL_SURFACE ( 'NONE', #3527, 0.5000000000000038858 ) ;
#13545=CARTESIAN_POINT ( 'NONE',  ( -51.19406879332065330, -13.71740939043347041, -8.000000000000000000 ) ) ;
#13548=CARTESIAN_POINT ( 'NONE',  ( 0.000000000000000000, 0.000000000000000000, -10.50000000000000000 ) ) ;
#13551=VERTEX_POINT ( 'NONE', #10500 ) ;
#13552=VERTEX_POINT ( 'NONE', #12713 ) ;
#13554=DIRECTION ( 'NONE',  ( 1.000000000000000000, 0.000000000000000000, 0.000000000000000000 ) ) ;
#13555=DIRECTION ( 'NONE',  ( 0.000000000000000000, 0.000000000000000000, -1.000000000000000000 ) ) ;
#13557=AXIS2_PLACEMENT_3D ( 'NONE', #314, #13001, #2593 ) ;
#13559=ORIENTED_EDGE ( 'NONE', *, *, #5389, .T. ) ;
#13561=FACE_OUTER_BOUND ( 'NONE', #12709, .T. ) ;
#13565=CARTESIAN_POINT ( 'NONE',  ( 15.88467684210547226, -49.11971303961683333, -8.000000000000000000 ) ) ;
#13567=EDGE_LOOP ( 'NONE', ( #4243, #9099, #4278, #7447, #1354, #5823 ) ) ;
#13568=VERTEX_POINT ( 'NONE', #9205 ) ;
#13569=CIRCLE ( 'NONE', #10417, 52.50000000000000711 ) ;
#13570=VERTEX_POINT ( 'NONE', #4745 ) ;
#13572=VECTOR ( 'NONE', #557, 1000.000000000000000 ) ;
#13575=EDGE_CURVE ( 'NONE', #12855, #6102, #12646, .T. ) ;
#13576=CIRCLE ( 'NONE', #14553, 0.5000000000000073275 ) ;
#13580=DIRECTION ( 'NONE',  ( -0.000000000000000000, -0.000000000000000000, 1.000000000000000000 ) ) ;
#13581=FACE_OUTER_BOUND ( 'NONE', #4841, .T. ) ;
#13582=CARTESIAN_POINT ( 'NONE',  ( -68.49330278050074128, 68.09867107463051639, -13.00000000000000178 ) ) ;
#13583=CIRCLE ( 'NONE', #6774, 3.000000000000002665 ) ;
#13584=DIRECTION ( 'NONE',  ( 1.000000000000000000, 0.000000000000000000, 0.000000000000000000 ) ) ;
#13585=ORIENTED_EDGE ( 'NONE', *, *, #12846, .F. ) ;
#13586=CIRCLE ( 'NONE', #10435, 100.0000000000000000 ) ;
#13587=CYLINDRICAL_SURFACE ( 'NONE', #6063, 3.000000000000002665 ) ;
#13588=ORIENTED_EDGE ( 'NONE', *, *, #7358, .F. ) ;
#13589=STYLED_ITEM ( 'NONE', ( #8261 ), #7823 ) ;
#13590=DIRECTION ( 'NONE',  ( -1.000000000000000000, 0.000000000000000000, 0.000000000000000000 ) ) ;
#13591=CARTESIAN_POINT ( 'NONE',  ( -26.01305530232562546, -46.81487971942612347, -10.50000000000000000 ) ) ;
#13592=EDGE_LOOP ( 'NONE', ( #7843, #12459 ) ) ;
#13594=AXIS2_PLACEMENT_3D ( 'NONE', #7668, #7588, #12237 ) ;
#13595=EDGE_LOOP ( 'NONE', ( #728, #7743, #11184, #12673, #11762, #3773, #2580, #8636, #6206, #2298 ) ) ;
#13596=AXIS2_PLACEMENT_3D ( 'NONE', #8413, #9538, #2640 ) ;
#13597=CARTESIAN_POINT ( 'NONE',  ( 89.61631465359491244, 37.12029293941346708, -8.000000000000000000 ) ) ;
#13598=ORIENTED_EDGE ( 'NONE', *, *, #2179, .T. ) ;
#13599=DIRECTION ( 'NONE',  ( 0.000000000000000000, 0.000000000000000000, 1.000000000000000000 ) ) ;
#13604=DIRECTION ( 'NONE',  ( 0.000000000000000000, 0.000000000000000000, 1.000000000000000000 ) ) ;
#13605=ADVANCED_FACE ( 'NONE', ( #5608 ), #13662, .T. ) ;
#13607=CARTESIAN_POINT ( 'NONE',  ( 44.79355920668810853, 31.05588327715852159, -8.000000000000000000 ) ) ;
#13609=ORIENTED_EDGE ( 'NONE', *, *, #7560, .F. ) ;
#13610=LINE ( 'NONE', #10188, #10099 ) ;
#13616=DIRECTION ( 'NONE',  ( 0.000000000000000000, 0.000000000000000000, -1.000000000000000000 ) ) ;
#13617=ORIENTED_EDGE ( 'NONE', *, *, #9127, .F. ) ;
#13618=DIRECTION ( 'NONE',  ( 0.000000000000000000, 0.000000000000000000, -1.000000000000000000 ) ) ;
#13619=ORIENTED_EDGE ( 'NONE', *, *, #13447, .T. ) ;
#13620=AXIS2_PLACEMENT_3D ( 'NONE', #13167, #2762, #11112 ) ;
#13621=DIRECTION ( 'NONE',  ( 0.000000000000000000, 0.000000000000000000, 1.000000000000000000 ) ) ;
#13622=DIRECTION ( 'NONE',  ( 1.000000000000000000, 0.000000000000000000, 0.000000000000000000 ) ) ;
#13623=EDGE_LOOP ( 'NONE', ( #13736, #1596, #3489, #10936, #11464 ) ) ;
#13624=EDGE_CURVE ( 'NONE', #10362, #13021, #14591, .T. ) ;
#13626=EDGE_CURVE ( 'NONE', #12871, #2381, #9971, .T. ) ;
#13628=CARTESIAN_POINT ( 'NONE',  ( 89.61631465359491244, 37.12029293941346708, -10.50000000000000000 ) ) ;
#13631=ORIENTED_EDGE ( 'NONE', *, *, #8649, .F. ) ;
#13632=ORIENTED_EDGE ( 'NONE', *, *, #2965, .F. ) ;
#13633=DIRECTION ( 'NONE',  ( 0.000000000000000000, 0.000000000000000000, 1.000000000000000000 ) ) ;
#13634=CARTESIAN_POINT ( 'NONE',  ( 26.01438936481372721, 47.21331623427104063, -13.00000000000000178 ) ) ;
#13635=CIRCLE ( 'NONE', #7324, 59.50000000000000000 ) ;
#13638=EDGE_CURVE ( 'NONE', #3039, #6857, #5375, .T. ) ;
#13641=ORIENTED_EDGE ( 'NONE', *, *, #3291, .F. ) ;
#13642=DIRECTION ( 'NONE',  ( 0.000000000000000000, 0.000000000000000000, 1.000000000000000000 ) ) ;
#13645=CARTESIAN_POINT ( 'NONE',  ( -50.00000000000000000, 0.000000000000000000, 8.000000000000000000 ) ) ;
#13646=EDGE_CURVE ( 'NONE', #11976, #11994, #10708, .T. ) ;
#13647=CYLINDRICAL_SURFACE ( 'NONE', #77, 0.5000000000000073275 ) ;
#13649=DIRECTION ( 'NONE',  ( -1.000000000000000000, 0.000000000000000000, 0.000000000000000000 ) ) ;
#13651=FACE_BOUND ( 'NONE', #9746, .T. ) ;
#13653=VERTEX_POINT ( 'NONE', #3188 ) ;
#13654=FACE_OUTER_BOUND ( 'NONE', #2006, .T. ) ;
#13655=AXIS2_PLACEMENT_3D ( 'NONE', #426, #14246, #4828 ) ;
#13656=ORIENTED_EDGE ( 'NONE', *, *, #13821, .T. ) ;
#13657=CIRCLE ( 'NONE', #9038, 3.000000000000002665 ) ;
#13658=ORIENTED_EDGE ( 'NONE', *, *, #6905, .F. ) ;
#13659=DIRECTION ( 'NONE',  ( -1.000000000000000000, 0.000000000000000000, 0.000000000000000000 ) ) ;
#13660=ORIENTED_EDGE ( 'NONE', *, *, #3072, .F. ) ;
#13662=CYLINDRICAL_SURFACE ( 'NONE', #11450, 63.00000000000000000 ) ;
#13663=CIRCLE ( 'NONE', #9529, 59.50000000000000000 ) ;
#13664=CYLINDRICAL_SURFACE ( 'NONE', #7643, 0.5000000000000004441 ) ;
#13667=CARTESIAN_POINT ( 'NONE',  ( 0.000000000000000000, 0.000000000000000000, -8.000000000000000000 ) ) ;
#13668=CIRCLE ( 'NONE', #13183, 50.00000000000000000 ) ;
#13670=FACE_OUTER_BOUND ( 'NONE', #4582, .T. ) ;
#13671=VERTEX_POINT ( 'NONE', #5758 ) ;
#13672=EDGE_CURVE ( 'NONE', #10698, #14931, #10961, .T. ) ;
#13673=AXIS2_PLACEMENT_3D ( 'NONE', #2750, #9499, #4889 ) ;
#13675=DIRECTION ( 'NONE',  ( -0.000000000000000000, -0.000000000000000000, -1.000000000000000000 ) ) ;
#13676=EDGE_CURVE ( 'NONE', #4514, #469, #12418, .T. ) ;
#13677=CIRCLE ( 'NONE', #3504, 57.00000000000000000 ) ;
#13679=PLANE ( 'NONE',  #13221 ) ;
#13681=CARTESIAN_POINT ( 'NONE',  ( 49.11971303961677648, 15.88467684210564990, 8.000000000000000000 ) ) ;
#13682=FACE_OUTER_BOUND ( 'NONE', #11488, .T. ) ;
#13683=CYLINDRICAL_SURFACE ( 'NONE', #14565, 0.5000000000000004441 ) ;
#13686=AXIS2_PLACEMENT_3D ( 'NONE', #3237, #11444, #1043 ) ;
#13688=DIRECTION ( 'NONE',  ( 1.000000000000000000, 0.000000000000000000, 0.000000000000000000 ) ) ;
#13690=EDGE_CURVE ( 'NONE', #8255, #2714, #4658, .T. ) ;
#13691=ORIENTED_EDGE ( 'NONE', *, *, #5862, .T. ) ;
#13692=CARTESIAN_POINT ( 'NONE',  ( -12.86891638962156215, 56.43380494353993271, 8.000000000000000000 ) ) ;
#13693=VERTEX_POINT ( 'NONE', #14807 ) ;
#13694=EDGE_CURVE ( 'NONE', #14215, #3803, #12756, .T. ) ;
#13695=CARTESIAN_POINT ( 'NONE',  ( -31.95997502295763582, 41.65105036529000415, -10.50000000000000000 ) ) ;
#13697=CIRCLE ( 'NONE', #1815, 0.5000000000000022204 ) ;
#13698=DIRECTION ( 'NONE',  ( 1.000000000000000000, 0.000000000000000000, 0.000000000000000000 ) ) ;
#13700=VECTOR ( 'NONE', #1634, 1000.000000000000000 ) ;
#13701=AXIS2_PLACEMENT_3D ( 'NONE', #1344, #6023, #5955 ) ;
#13702=CARTESIAN_POINT ( 'NONE',  ( 0.000000000000000000, 0.000000000000000000, -10.50000000000000000 ) ) ;
#13703=ORIENTED_EDGE ( 'NONE', *, *, #5699, .T. ) ;
#13705=EDGE_LOOP ( 'NONE', ( #1045, #1947, #9641, #12932, #12592, #8288 ) ) ;
#13707=DIRECTION ( 'NONE',  ( 0.000000000000000000, 0.000000000000000000, 1.000000000000000000 ) ) ;
#13708=ORIENTED_EDGE ( 'NONE', *, *, #14836, .F. ) ;
#13709=( GEOMETRIC_REPRESENTATION_CONTEXT ( 3 ) GLOBAL_UNCERTAINTY_ASSIGNED_CONTEXT ( ( #14737 ) ) GLOBAL_UNIT_ASSIGNED_CONTEXT ( ( #3058, #1902, #14674 ) ) REPRESENTATION_CONTEXT ( 'NONE', 'WORKASPACE' ) );
#13710=CARTESIAN_POINT ( 'NONE',  ( -68.58935777509570642, -68.58935777509452691, -13.00000000000000178 ) ) ;
#13712=ORIENTED_EDGE ( 'NONE', *, *, #1572, .T. ) ;
#13713=CIRCLE ( 'NONE', #11413, 50.00000000000000000 ) ;
#13715=CIRCLE ( 'NONE', #10314, 3.000000000000002665 ) ;
#13716=VERTEX_POINT ( 'NONE', #9019 ) ;
#13717=ORIENTED_EDGE ( 'NONE', *, *, #7014, .F. ) ;
#13719=CARTESIAN_POINT ( 'NONE',  ( -12.86891638962156215, 56.43380494353993271, -13.00000000000000178 ) ) ;
#13723=ORIENTED_EDGE ( 'NONE', *, *, #13125, .T. ) ;
#13725=CIRCLE ( 'NONE', #7154, 3.000000000000002665 ) ;
#13726=EDGE_CURVE ( 'NONE', #2878, #14215, #14348, .T. ) ;
#13727=ORIENTED_EDGE ( 'NONE', *, *, #2021, .T. ) ;
#13728=ORIENTED_EDGE ( 'NONE', *, *, #6369, .T. ) ;
#13730=DIRECTION ( 'NONE',  ( 0.000000000000000000, 0.000000000000000000, -1.000000000000000000 ) ) ;
#13734=AXIS2_PLACEMENT_3D ( 'NONE', #4002, #353, #2557 ) ;
#13736=ORIENTED_EDGE ( 'NONE', *, *, #12795, .T. ) ;
#13737=CARTESIAN_POINT ( 'NONE',  ( -9.706953719245875689, -57.06275842387046993, -13.00000000000000178 ) ) ;
#13741=ORIENTED_EDGE ( 'NONE', *, *, #13254, .F. ) ;
#13742=EDGE_CURVE ( 'NONE', #3199, #4159, #12906, .T. ) ;
#13743=EDGE_CURVE ( 'NONE', #4485, #3890, #2230, .T. ) ;
#13744=ORIENTED_EDGE ( 'NONE', *, *, #4587, .T. ) ;
#13746=CIRCLE ( 'NONE', #649, 0.5000000000000004441 ) ;
#13747=EDGE_LOOP ( 'NONE', ( #9503, #12199, #3154, #402, #9526, #7758 ) ) ;
#13748=LINE ( 'NONE', #60, #8265 ) ;
#13749=DIRECTION ( 'NONE',  ( 1.000000000000000000, 0.000000000000000000, 0.000000000000000000 ) ) ;
#13752=DIRECTION ( 'NONE',  ( 1.000000000000000000, 0.000000000000000000, -0.000000000000000000 ) ) ;
#13754=AXIS2_PLACEMENT_3D ( 'NONE', #11605, #11540, #9158 ) ;
#13755=CIRCLE ( 'NONE', #8160, 3.000000000000002665 ) ;
#13756=DIRECTION ( 'NONE',  ( 0.000000000000000000, 0.000000000000000000, 1.000000000000000000 ) ) ;
#13759=DIRECTION ( 'NONE',  ( 1.000000000000000000, 0.000000000000000000, 0.000000000000000000 ) ) ;
#13760=ORIENTED_EDGE ( 'NONE', *, *, #4455, .T. ) ;
#13761=CARTESIAN_POINT ( 'NONE',  ( 39.66766701456161570, 30.43807145043622597, -8.000000000000000000 ) ) ;
#13762=VERTEX_POINT ( 'NONE', #3412 ) ;
#13763=DIRECTION ( 'NONE',  ( 0.000000000000000000, 0.000000000000000000, -1.000000000000000000 ) ) ;
#13766=CARTESIAN_POINT ( 'NONE',  ( -23.50071946824040836, -45.96504489226015977, -8.000000000000000000 ) ) ;
#13767=DIRECTION ( 'NONE',  ( -1.000000000000000000, 0.000000000000000000, 0.000000000000000000 ) ) ;
#13769=FACE_OUTER_BOUND ( 'NONE', #4556, .T. ) ;
#13771=DIRECTION ( 'NONE',  ( -0.000000000000000000, -0.000000000000000000, -1.000000000000000000 ) ) ;
#13772=VERTEX_POINT ( 'NONE', #12976 ) ;
#13773=DIRECTION ( 'NONE',  ( -0.000000000000000000, -0.000000000000000000, 1.000000000000000000 ) ) ;
#13775=CIRCLE ( 'NONE', #4792, 0.5000000000000043299 ) ;
#13776=DIRECTION ( 'NONE',  ( 0.000000000000000000, 0.000000000000000000, 1.000000000000000000 ) ) ;
#13777=DIRECTION ( 'NONE',  ( -0.000000000000000000, -0.000000000000000000, 1.000000000000000000 ) ) ;
#13780=ORIENTED_EDGE ( 'NONE', *, *, #8510, .T. ) ;
#13781=EDGE_CURVE ( 'NONE', #5385, #7405, #9012, .T. ) ;
#13782=DIRECTION ( 'NONE',  ( 1.000000000000000000, 0.000000000000000000, 0.000000000000000000 ) ) ;
#13783=ADVANCED_FACE ( 'NONE', ( #1365 ), #14038, .F. ) ;
#13784=CYLINDRICAL_SURFACE ( 'NONE', #12915, 0.5000000000000004441 ) ;
#13786=AXIS2_PLACEMENT_3D ( 'NONE', #7177, #14102, #5814 ) ;
#13788=DIRECTION ( 'NONE',  ( -1.000000000000000000, 0.000000000000000000, 0.000000000000000000 ) ) ;
#13789=ORIENTED_EDGE ( 'NONE', *, *, #5315, .T. ) ;
#13792=EDGE_CURVE ( 'NONE', #2920, #5532, #7557, .T. ) ;
#13793=DIRECTION ( 'NONE',  ( 1.000000000000000000, 0.000000000000000000, 0.000000000000000000 ) ) ;
#13794=DIRECTION ( 'NONE',  ( -0.000000000000000000, -0.000000000000000000, -1.000000000000000000 ) ) ;
#13795=DIRECTION ( 'NONE',  ( -0.000000000000000000, -0.000000000000000000, -1.000000000000000000 ) ) ;
#13796=ORIENTED_EDGE ( 'NONE', *, *, #8508, .T. ) ;
#13798=VERTEX_POINT ( 'NONE', #3568 ) ;
#13801=DIRECTION ( 'NONE',  ( -0.000000000000000000, -0.000000000000000000, -1.000000000000000000 ) ) ;
#13802=DIRECTION ( 'NONE',  ( -0.000000000000000000, -0.000000000000000000, 1.000000000000000000 ) ) ;
#13804=CARTESIAN_POINT ( 'NONE',  ( -36.14014761921588104, 11.74264578624790190, -28.00000000000000000 ) ) ;
#13805=EDGE_CURVE ( 'NONE', #12336, #14898, #10890, .T. ) ;
#13808=AXIS2_PLACEMENT_3D ( 'NONE', #769, #4191, #13511 ) ;
#13809=DIRECTION ( 'NONE',  ( 0.000000000000000000, 0.000000000000000000, 1.000000000000000000 ) ) ;
#13810=ADVANCED_FACE ( 'NONE', ( #9391 ), #8610, .F. ) ;
#13815=ORIENTED_EDGE ( 'NONE', *, *, #4343, .T. ) ;
#13816=DIRECTION ( 'NONE',  ( 1.000000000000000000, 0.000000000000000000, 0.000000000000000000 ) ) ;
#13817=VECTOR ( 'NONE', #9765, 1000.000000000000000 ) ;
#13818=DIRECTION ( 'NONE',  ( 1.000000000000000000, 1.826024711554534012E-15, 0.000000000000000000 ) ) ;
#13819=LINE ( 'NONE', #12823, #5472 ) ;
#13821=EDGE_CURVE ( 'NONE', #2546, #2335, #4181, .T. ) ;
#13822=DIRECTION ( 'NONE',  ( 0.000000000000000000, 0.000000000000000000, 1.000000000000000000 ) ) ;
#13823=EDGE_CURVE ( 'NONE', #4604, #9310, #13143, .T. ) ;
#13824=ORIENTED_EDGE ( 'NONE', *, *, #14225, .T. ) ;
#13829=CARTESIAN_POINT ( 'NONE',  ( -51.45950017607691507, 4.121772567811807342, 8.000000000000000000 ) ) ;
#13830=CIRCLE ( 'NONE', #977, 50.00000000000000000 ) ;
#13831=ORIENTED_EDGE ( 'NONE', *, *, #4347, .T. ) ;
#13832=CARTESIAN_POINT ( 'NONE',  ( -57.06275842387042729, 9.706953719246069312, -13.00000000000000178 ) ) ;
#13833=EDGE_CURVE ( 'NONE', #12431, #1277, #11840, .T. ) ;
#13834=EDGE_LOOP ( 'NONE', ( #8785, #4776, #6218, #4986, #3344, #396, #7181, #12677, #14218 ) ) ;
#13837=AXIS2_PLACEMENT_3D ( 'NONE', #7203, #14129, #6213 ) ;
#13838=CYLINDRICAL_SURFACE ( 'NONE', #10788, 63.00000000000000000 ) ;
#13839=CIRCLE ( 'NONE', #4857, 59.50000000000000000 ) ;
#13840=CARTESIAN_POINT ( 'NONE',  ( -9.706953719245875689, -57.06275842387046993, -10.50000000000000000 ) ) ;
#13842=AXIS2_PLACEMENT_3D ( 'NONE', #11856, #9004, #12230 ) ;
#13844=ADVANCED_FACE ( 'NONE', ( #7542 ), #9741, .T. ) ;
#13847=ORIENTED_EDGE ( 'NONE', *, *, #6799, .F. ) ;
#13848=AXIS2_PLACEMENT_3D ( 'NONE', #7211, #3820, #3962 ) ;
#13849=CARTESIAN_POINT ( 'NONE',  ( 7.252293700257532727, 53.06332297728244640, -10.50000000000000000 ) ) ;
#13850=DIRECTION ( 'NONE',  ( 1.000000000000000000, 0.000000000000000000, 0.000000000000000000 ) ) ;
#13851=CIRCLE ( 'NONE', #9229, 63.00000000000000000 ) ;
#13854=CARTESIAN_POINT ( 'NONE',  ( 49.00442420935993226, -30.80502811811213704, 8.000000000000000000 ) ) ;
#13855=AXIS2_PLACEMENT_3D ( 'NONE', #6314, #7619, #1785 ) ;
#13856=VERTEX_POINT ( 'NONE', #4778 ) ;
#13860=DIRECTION ( 'NONE',  ( 1.000000000000000000, 0.000000000000000000, -0.000000000000000000 ) ) ;
#13861=AXIS2_PLACEMENT_3D ( 'NONE', #4094, #8703, #11077 ) ;
#13862=DIRECTION ( 'NONE',  ( 0.000000000000000000, 0.000000000000000000, 1.000000000000000000 ) ) ;
#13863=DIRECTION ( 'NONE',  ( -1.000000000000000000, 0.000000000000000000, 0.000000000000000000 ) ) ;
#13864=VERTEX_POINT ( 'NONE', #13258 ) ;
#13865=VECTOR ( 'NONE', #6946, 1000.000000000000000 ) ;
#13867=AXIS2_PLACEMENT_3D ( 'NONE', #11621, #7887, #1146 ) ;
#13870=CARTESIAN_POINT ( 'NONE',  ( 45.88839665196118744, -26.99988008862642630, -13.00000000000000178 ) ) ;
#13872=FACE_OUTER_BOUND ( 'NONE', #7987, .T. ) ;
#13874=EDGE_LOOP ( 'NONE', ( #8770, #1187, #5036, #11598, #3384, #5116, #3443, #3228, #6858, #6020 ) ) ;
#13876=AXIS2_PLACEMENT_3D ( 'NONE', #167, #6917, #11794 ) ;
#13877=VERTEX_POINT ( 'NONE', #13975 ) ;
#13878=EDGE_LOOP ( 'NONE', ( #11165, #158, #6187, #14188, #4086 ) ) ;
#13879=AXIS2_PLACEMENT_3D ( 'NONE', #7771, #14849, #11281 ) ;
#13881=ADVANCED_FACE ( 'NONE', ( #1287 ), #5901, .F. ) ;
#13882=DIRECTION ( 'NONE',  ( 1.000000000000000000, 0.000000000000000000, 0.000000000000000000 ) ) ;
#13883=CARTESIAN_POINT ( 'NONE',  ( 68.09867107462983427, 68.49330278050145182, -10.50000000000000000 ) ) ;
#13884=DIRECTION ( 'NONE',  ( -1.000000000000000000, -6.833935844856531060E-14, 0.000000000000000000 ) ) ;
#13886=FACE_OUTER_BOUND ( 'NONE', #12346, .T. ) ;
#13887=ORIENTED_EDGE ( 'NONE', *, *, #937, .T. ) ;
#13888=ADVANCED_FACE ( 'NONE', ( #5432 ), #12414, .F. ) ;
#13889=EDGE_LOOP ( 'NONE', ( #267, #9329, #10366, #8618, #14290, #958, #891, #1983, #6757 ) ) ;
#13892=CIRCLE ( 'NONE', #14128, 59.50000000000000000 ) ;
#13894=EDGE_LOOP ( 'NONE', ( #3651, #8928 ) ) ;
#13895=EDGE_LOOP ( 'NONE', ( #4983, #5300, #6453, #8863, #8559, #13100 ) ) ;
#13896=LINE ( 'NONE', #1143, #2324 ) ;
#13898=CIRCLE ( 'NONE', #2248, 59.50000000000000000 ) ;
#13899=DIRECTION ( 'NONE',  ( 0.000000000000000000, 0.000000000000000000, 1.000000000000000000 ) ) ;
#13901=AXIS2_PLACEMENT_3D ( 'NONE', #7605, #13462, #1992 ) ;
#13902=DIRECTION ( 'NONE',  ( 1.000000000000000000, 0.000000000000000000, 0.000000000000000000 ) ) ;
#13906=DIRECTION ( 'NONE',  ( 0.000000000000000000, 0.000000000000000000, 1.000000000000000000 ) ) ;
#13908=CIRCLE ( 'NONE', #7335, 56.99999999999999289 ) ;
#13909=CARTESIAN_POINT ( 'NONE',  ( 70.20695371924547601, 57.06275842387054098, 10.49999999999999822 ) ) ;
#13910=AXIS2_PLACEMENT_3D ( 'NONE', #4803, #5857, #2441 ) ;
#13911=ORIENTED_EDGE ( 'NONE', *, *, #13061, .F. ) ;
#13912=CARTESIAN_POINT ( 'NONE',  ( -33.48561063518626923, 47.21331623427104063, -13.00000000000000178 ) ) ;
#13913=ORIENTED_EDGE ( 'NONE', *, *, #7260, .T. ) ;
#13915=AXIS2_PLACEMENT_3D ( 'NONE', #8539, #8615, #13185 ) ;
#13917=EDGE_CURVE ( 'NONE', #1935, #3975, #2008, .T. ) ;
#13918=DIRECTION ( 'NONE',  ( 0.000000000000000000, 0.000000000000000000, 1.000000000000000000 ) ) ;
#13919=EDGE_CURVE ( 'NONE', #14223, #4677, #14601, .T. ) ;
#13922=LINE ( 'NONE', #3513, #12856 ) ;
#13925=EDGE_CURVE ( 'NONE', #14497, #7611, #9983, .T. ) ;
#13926=DIRECTION ( 'NONE',  ( 1.000000000000000000, 0.000000000000000000, 0.000000000000000000 ) ) ;
#13927=CIRCLE ( 'NONE', #3732, 52.50000000000000711 ) ;
#13928=ORIENTED_EDGE ( 'NONE', *, *, #3523, .F. ) ;
#13929=DIRECTION ( 'NONE',  ( 1.000000000000000000, 0.000000000000000000, 0.000000000000000000 ) ) ;
#13930=DIRECTION ( 'NONE',  ( 0.000000000000000000, 0.000000000000000000, 1.000000000000000000 ) ) ;
#13931=FACE_OUTER_BOUND ( 'NONE', #7086, .T. ) ;
#13932=CARTESIAN_POINT ( 'NONE',  ( 0.000000000000000000, 0.000000000000000000, -13.00000000000000178 ) ) ;
#13933=EDGE_CURVE ( 'NONE', #6415, #11737, #8291, .T. ) ;
#13934=ORIENTED_EDGE ( 'NONE', *, *, #15003, .F. ) ;
#13936=AXIS2_PLACEMENT_3D ( 'NONE', #12437, #6648, #3099 ) ;
#13937=DIRECTION ( 'NONE',  ( 1.000000000000000000, 0.000000000000000000, 0.000000000000000000 ) ) ;
#13938=AXIS2_PLACEMENT_3D ( 'NONE', #11810, #11734, #13091 ) ;
#13939=ORIENTED_EDGE ( 'NONE', *, *, #5049, .F. ) ;
#13941=DIRECTION ( 'NONE',  ( 0.000000000000000000, 0.000000000000000000, -1.000000000000000000 ) ) ;
#13942=CARTESIAN_POINT ( 'NONE',  ( 31.05588327715836527, -44.79355920668822932, -13.00000000000000178 ) ) ;
#13943=DIRECTION ( 'NONE',  ( -0.000000000000000000, -0.000000000000000000, -1.000000000000000000 ) ) ;
#13944=EDGE_LOOP ( 'NONE', ( #2458, #7558, #10353, #10906, #1105 ) ) ;
#13946=CIRCLE ( 'NONE', #4256, 3.000000000000002665 ) ;
#13947=CARTESIAN_POINT ( 'NONE',  ( 92.38795325112877777, 38.26834323650874126, 8.000000000000000000 ) ) ;
#13948=CARTESIAN_POINT ( 'NONE',  ( -44.89637028918152595, 0.000000000000000000, -25.50000000000000355 ) ) ;
#13950=CARTESIAN_POINT ( 'NONE',  ( 41.59008834022645829, 32.46576781417968505, -13.00000000000000178 ) ) ;
#13952=ORIENTED_EDGE ( 'NONE', *, *, #8373, .T. ) ;
#13954=ORIENTED_EDGE ( 'NONE', *, *, #9405, .F. ) ;
#13955=AXIS2_PLACEMENT_3D ( 'NONE', #6104, #5127, #9740 ) ;
#13956=CARTESIAN_POINT ( 'NONE',  ( 51.19406879332056093, 13.71740939043382745, -13.00000000000000178 ) ) ;
#13957=AXIS2_PLACEMENT_3D ( 'NONE', #9340, #1090, #4793 ) ;
#13960=EDGE_CURVE ( 'NONE', #13160, #1886, #5624, .T. ) ;
#13961=DIRECTION ( 'NONE',  ( -0.000000000000000000, -0.000000000000000000, 1.000000000000000000 ) ) ;
#13962=EDGE_CURVE ( 'NONE', #6859, #12263, #2715, .T. ) ;
#13964=ORIENTED_EDGE ( 'NONE', *, *, #10747, .F. ) ;
#13966=DIRECTION ( 'NONE',  ( 1.000000000000000000, 0.000000000000000000, 0.000000000000000000 ) ) ;
#13967=AXIS2_PLACEMENT_3D ( 'NONE', #12028, #6223, #10865 ) ;
#13968=ORIENTED_EDGE ( 'NONE', *, *, #10753, .T. ) ;
#13969=ORIENTED_EDGE ( 'NONE', *, *, #7548, .F. ) ;
#13970=CARTESIAN_POINT ( 'NONE',  ( -86.67575032682103142, -37.71449950291016506, 8.000000000000000000 ) ) ;
#13971=EDGE_LOOP ( 'NONE', ( #12091, #11674, #780, #11805 ) ) ;
#13972=ORIENTED_EDGE ( 'NONE', *, *, #642, .T. ) ;
#13973=CIRCLE ( 'NONE', #6674, 59.49999999999999289 ) ;
#13975=CARTESIAN_POINT ( 'NONE',  ( 20.00000000000000000, 2.449293598294706513E-15, -28.00000000000000000 ) ) ;
#13978=DIRECTION ( 'NONE',  ( 0.000000000000000000, 0.000000000000000000, 1.000000000000000000 ) ) ;
#13979=ADVANCED_FACE ( 'NONE', ( #8985 ), #886, .F. ) ;
#13980=EDGE_CURVE ( 'NONE', #877, #11546, #9497, .T. ) ;
#13982=CARTESIAN_POINT ( 'NONE',  ( -19.68583958711381854, -30.74264578624812927, -28.00000000000000000 ) ) ;
#13984=DIRECTION ( 'NONE',  ( 1.000000000000000000, 0.000000000000000000, 0.000000000000000000 ) ) ;
#13986=CYLINDRICAL_SURFACE ( 'NONE', #3056, 63.00000000000000000 ) ;
#13987=ORIENTED_EDGE ( 'NONE', *, *, #441, .F. ) ;
#13989=DIRECTION ( 'NONE',  ( 1.000000000000000000, 0.000000000000000000, 0.000000000000000000 ) ) ;
#13993=CIRCLE ( 'NONE', #3322, 3.000000000000002665 ) ;
#13994=DIRECTION ( 'NONE',  ( 0.000000000000000000, 0.000000000000000000, 1.000000000000000000 ) ) ;
#13995=CARTESIAN_POINT ( 'NONE',  ( -22.33583958711380646, -30.74264578624812927, -25.50000000000000355 ) ) ;
#13997=EDGE_CURVE ( 'NONE', #6857, #9553, #12496, .T. ) ;
#13999=LINE ( 'NONE', #10415, #10522 ) ;
#14001=CARTESIAN_POINT ( 'NONE',  ( 0.000000000000000000, 0.000000000000000000, -10.50000000000000000 ) ) ;
#14002=CARTESIAN_POINT ( 'NONE',  ( 97.00000000000000000, -3.384287605079545030E-13, -8.000000000000000000 ) ) ;
#14004=EDGE_CURVE ( 'NONE', #5446, #12855, #2959, .T. ) ;
#14005=DIRECTION ( 'NONE',  ( 1.000000000000000000, 0.000000000000000000, 0.000000000000000000 ) ) ;
#14009=CARTESIAN_POINT ( 'NONE',  ( -89.61631465359441506, 37.12029293941468211, -13.00000000000000178 ) ) ;
#14010=LINE ( 'NONE', #13942, #732 ) ;
#14011=DIRECTION ( 'NONE',  ( 0.000000000000000000, 0.000000000000000000, 1.000000000000000000 ) ) ;
#14012=EDGE_CURVE ( 'NONE', #14795, #6680, #1997, .T. ) ;
#14013=ORIENTED_EDGE ( 'NONE', *, *, #10283, .T. ) ;
#14014=EDGE_CURVE ( 'NONE', #7044, #1401, #8076, .T. ) ;
#14018=ORIENTED_EDGE ( 'NONE', *, *, #2376, .T. ) ;
#14020=ADVANCED_FACE ( 'NONE', ( #9424 ), #3679, .T. ) ;
#14021=VERTEX_POINT ( 'NONE', #1109 ) ;
#14022=DIRECTION ( 'NONE',  ( 1.000000000000000000, 0.000000000000000000, 0.000000000000000000 ) ) ;
#14023=CARTESIAN_POINT ( 'NONE',  ( 89.61631465359491244, 37.12029293941346708, 8.000000000000000000 ) ) ;
#14026=DIRECTION ( 'NONE',  ( 0.000000000000000000, 0.000000000000000000, 1.000000000000000000 ) ) ;
#14028=ORIENTED_EDGE ( 'NONE', *, *, #13259, .F. ) ;
#14030=DIRECTION ( 'NONE',  ( 1.000000000000000000, 0.000000000000000000, 0.000000000000000000 ) ) ;
#14031=DIRECTION ( 'NONE',  ( 0.000000000000000000, 0.000000000000000000, -1.000000000000000000 ) ) ;
#14032=DIRECTION ( 'NONE',  ( 0.000000000000000000, 0.000000000000000000, -1.000000000000000000 ) ) ;
#14035=DIRECTION ( 'NONE',  ( -1.000000000000000000, 0.000000000000000000, 0.000000000000000000 ) ) ;
#14036=EDGE_LOOP ( 'NONE', ( #14490, #11860, #9436, #10965, #5058 ) ) ;
#14037=CARTESIAN_POINT ( 'NONE',  ( 24.99999999999975131, 43.30127018922208038, -8.000000000000000000 ) ) ;
#14038=PLANE ( 'NONE',  #45 ) ;
#14039=CARTESIAN_POINT ( 'NONE',  ( 0.000000000000000000, 0.000000000000000000, -10.50000000000000000 ) ) ;
#14042=DIRECTION ( 'NONE',  ( 0.000000000000000000, 0.000000000000000000, -1.000000000000000000 ) ) ;
#14043=LINE ( 'NONE', #12826, #7493 ) ;
#14047=ADVANCED_FACE ( 'NONE', ( #14074 ), #12790, .T. ) ;
#14048=ORIENTED_EDGE ( 'NONE', *, *, #14856, .T. ) ;
#14050=EDGE_CURVE ( 'NONE', #3450, #4822, #11950, .T. ) ;
#14052=ORIENTED_EDGE ( 'NONE', *, *, #9676, .T. ) ;
#14054=FACE_OUTER_BOUND ( 'NONE', #10317, .T. ) ;
#14057=DIRECTION ( 'NONE',  ( 0.000000000000000000, 0.000000000000000000, 1.000000000000000000 ) ) ;
#14060=DIRECTION ( 'NONE',  ( 0.000000000000000000, 0.000000000000000000, 1.000000000000000000 ) ) ;
#14062=VERTEX_POINT ( 'NONE', #4813 ) ;
#14063=AXIS2_PLACEMENT_3D ( 'NONE', #9778, #11011, #11162 ) ;
#14065=CARTESIAN_POINT ( 'NONE',  ( -89.89283556784485540, 37.53686968382331202, -10.50000000000000000 ) ) ;
#14066=DIRECTION ( 'NONE',  ( 0.000000000000000000, 0.000000000000000000, 1.000000000000000000 ) ) ;
#14067=ADVANCED_FACE ( 'NONE', ( #3370 ), #2239, .F. ) ;
#14068=DIRECTION ( 'NONE',  ( 0.000000000000000000, 0.000000000000000000, -1.000000000000000000 ) ) ;
#14070=FACE_OUTER_BOUND ( 'NONE', #9014, .T. ) ;
#14071=ORIENTED_EDGE ( 'NONE', *, *, #2642, .T. ) ;
#14073=DIRECTION ( 'NONE',  ( 1.000000000000000000, 0.000000000000000000, 0.000000000000000000 ) ) ;
#14074=FACE_OUTER_BOUND ( 'NONE', #6865, .T. ) ;
#14075=DIRECTION ( 'NONE',  ( -0.000000000000000000, -0.000000000000000000, -1.000000000000000000 ) ) ;
#14076=CARTESIAN_POINT ( 'NONE',  ( 6.526309611002943711, 49.57224306869047581, 8.000000000000000000 ) ) ;
#14077=VECTOR ( 'NONE', #13918, 1000.000000000000000 ) ;
#14078=ORIENTED_EDGE ( 'NONE', *, *, #9493, .T. ) ;
#14080=AXIS2_PLACEMENT_3D ( 'NONE', #6913, #4949, #6066 ) ;
#14081=LINE ( 'NONE', #13313, #8843 ) ;
#14082=AXIS2_PLACEMENT_3D ( 'NONE', #12240, #4275, #12165 ) ;
#14086=AXIS2_PLACEMENT_3D ( 'NONE', #10773, #4939, #446 ) ;
#14087=EDGE_CURVE ( 'NONE', #5893, #7269, #3216, .T. ) ;
#14088=ORIENTED_EDGE ( 'NONE', *, *, #8742, .F. ) ;
#14089=VECTOR ( 'NONE', #5243, 1000.000000000000000 ) ;
#14092=CIRCLE ( 'NONE', #11181, 3.000000000000002665 ) ;
#14093=DIRECTION ( 'NONE',  ( 1.000000000000000000, 0.000000000000000000, 0.000000000000000000 ) ) ;
#14094=CIRCLE ( 'NONE', #5362, 63.00000000000000000 ) ;
#14095=CARTESIAN_POINT ( 'NONE',  ( -37.53686968382306333, -89.89283556784496909, 10.49999999999999822 ) ) ;
#14096=CARTESIAN_POINT ( 'NONE',  ( -70.71067811865538033, -70.71067811865414399, 8.000000000000000000 ) ) ;
#14097=ORIENTED_EDGE ( 'NONE', *, *, #2825, .T. ) ;
#14098=ORIENTED_EDGE ( 'NONE', *, *, #14190, .F. ) ;
#14100=ADVANCED_FACE ( 'NONE', ( #4748 ), #13784, .F. ) ;
#14101=LINE ( 'NONE', #3706, #1332 ) ;
#14102=DIRECTION ( 'NONE',  ( 0.000000000000000000, 0.000000000000000000, -1.000000000000000000 ) ) ;
#14103=AXIS2_PLACEMENT_3D ( 'NONE', #5299, #5384, #12217 ) ;
#14106=CIRCLE ( 'NONE', #6807, 60.50000000000000711 ) ;
#14107=ORIENTED_EDGE ( 'NONE', *, *, #13417, .F. ) ;
#14108=DIRECTION ( 'NONE',  ( 0.000000000000000000, 0.000000000000000000, -1.000000000000000000 ) ) ;
#14110=ADVANCED_FACE ( 'NONE', ( #8219 ), #12637, .T. ) ;
#14111=CARTESIAN_POINT ( 'NONE',  ( -51.19406879332065330, -13.71740939043347041, -13.00000000000000178 ) ) ;
#14112=DIRECTION ( 'NONE',  ( 0.000000000000000000, 0.000000000000000000, 1.000000000000000000 ) ) ;
#14113=VECTOR ( 'NONE', #1311, 1000.000000000000000 ) ;
#14114=CARTESIAN_POINT ( 'NONE',  ( -68.58935777509427112, 68.58935777509594800, -8.000000000000000000 ) ) ;
#14115=CARTESIAN_POINT ( 'NONE',  ( 0.000000000000000000, 0.000000000000000000, -11.74999999999999822 ) ) ;
#14117=CARTESIAN_POINT ( 'NONE',  ( 9.706953719245472456, 57.06275842387054098, 8.000000000000000000 ) ) ;
#14118=AXIS2_PLACEMENT_3D ( 'NONE', #14626, #3227, #13622 ) ;
#14119=VERTEX_POINT ( 'NONE', #3830 ) ;
#14120=CARTESIAN_POINT ( 'NONE',  ( -38.79014761921587251, 11.74264578624790190, -28.00000000000000000 ) ) ;
#14121=ORIENTED_EDGE ( 'NONE', *, *, #7858, .T. ) ;
#14122=ORIENTED_EDGE ( 'NONE', *, *, #3879, .F. ) ;
#14124=ORIENTED_EDGE ( 'NONE', *, *, #9520, .T. ) ;
#14125=DIRECTION ( 'NONE',  ( 0.000000000000000000, 0.000000000000000000, 1.000000000000000000 ) ) ;
#14126=ORIENTED_EDGE ( 'NONE', *, *, #3757, .T. ) ;
#14127=CARTESIAN_POINT ( 'NONE',  ( 89.61631465359468507, -37.12029293941410657, -13.00000000000000178 ) ) ;
#14128=AXIS2_PLACEMENT_3D ( 'NONE', #8521, #13163, #12036 ) ;
#14129=DIRECTION ( 'NONE',  ( 0.000000000000000000, 0.000000000000000000, -1.000000000000000000 ) ) ;
#14131=CYLINDRICAL_SURFACE ( 'NONE', #7028, 56.99999999999999289 ) ;
#14132=CARTESIAN_POINT ( 'NONE',  ( 0.000000000000000000, 0.000000000000000000, -10.50000000000000000 ) ) ;
#14133=LINE ( 'NONE', #8572, #6031 ) ;
#14134=AXIS2_PLACEMENT_3D ( 'NONE', #9198, #8068, #13698 ) ;
#14135=EDGE_LOOP ( 'NONE', ( #4598, #10861, #8833, #14122, #8351, #9030 ) ) ;
#14136=EDGE_CURVE ( 'NONE', #2381, #4530, #11710, .T. ) ;
#14137=DIRECTION ( 'NONE',  ( -0.000000000000000000, -0.000000000000000000, 1.000000000000000000 ) ) ;
#14139=VECTOR ( 'NONE', #2671, 1000.000000000000000 ) ;
#14143=CIRCLE ( 'NONE', #2009, 0.5000000000000004441 ) ;
#14144=CARTESIAN_POINT ( 'NONE',  ( -20.00000000000000000, 0.000000000000000000, -28.00000000000000000 ) ) ;
#14147=VERTEX_POINT ( 'NONE', #11958 ) ;
#14148=DIRECTION ( 'NONE',  ( -1.000000000000000000, 0.000000000000000000, 0.000000000000000000 ) ) ;
#14150=CARTESIAN_POINT ( 'NONE',  ( 13.35619814848834075, -51.53979475227123430, 10.49999999999999822 ) ) ;
#14151=DIRECTION ( 'NONE',  ( 0.000000000000000000, 0.000000000000000000, 1.000000000000000000 ) ) ;
#14152=AXIS2_PLACEMENT_3D ( 'NONE', #4594, #5869, #3232 ) ;
#14154=FACE_OUTER_BOUND ( 'NONE', #51, .T. ) ;
#14156=ORIENTED_EDGE ( 'NONE', *, *, #8142, .T. ) ;
#14157=DIRECTION ( 'NONE',  ( 0.000000000000000000, 0.000000000000000000, -1.000000000000000000 ) ) ;
#14158=DIRECTION ( 'NONE',  ( 0.000000000000000000, 0.000000000000000000, -1.000000000000000000 ) ) ;
#14159=DIRECTION ( 'NONE',  ( 1.000000000000000000, 0.000000000000000000, 0.000000000000000000 ) ) ;
#14160=VECTOR ( 'NONE', #2522, 1000.000000000000000 ) ;
#14161=CIRCLE ( 'NONE', #10279, 3.000000000000002665 ) ;
#14165=FACE_OUTER_BOUND ( 'NONE', #2828, .T. ) ;
#14167=DIRECTION ( 'NONE',  ( 0.000000000000000000, 0.000000000000000000, 1.000000000000000000 ) ) ;
#14169=AXIS2_PLACEMENT_3D ( 'NONE', #9403, #10779, #3810 ) ;
#14170=AXIS2_PLACEMENT_3D ( 'NONE', #11815, #11739, #4901 ) ;
#14172=ORIENTED_EDGE ( 'NONE', *, *, #1164, .T. ) ;
#14175=ORIENTED_EDGE ( 'NONE', *, *, #9810, .T. ) ;
#14176=ADVANCED_FACE ( 'NONE', ( #11875 ), #10954, .F. ) ;
#14178=DIRECTION ( 'NONE',  ( 0.000000000000000000, 0.000000000000000000, 1.000000000000000000 ) ) ;
#14179=ADVANCED_FACE ( 'NONE', ( #9581 ), #8378, .T. ) ;
#14181=CARTESIAN_POINT ( 'NONE',  ( 69.08935777509475429, -68.58935777509547904, -13.00000000000000178 ) ) ;
#14182=ORIENTED_EDGE ( 'NONE', *, *, #651, .F. ) ;
#14183=CIRCLE ( 'NONE', #10055, 3.000000000000002665 ) ;
#14184=ORIENTED_EDGE ( 'NONE', *, *, #1629, .F. ) ;
#14185=DIRECTION ( 'NONE',  ( 0.000000000000000000, 0.000000000000000000, -1.000000000000000000 ) ) ;
#14186=CIRCLE ( 'NONE', #9330, 44.89637028918152595 ) ;
#14187=AXIS2_PLACEMENT_3D ( 'NONE', #12323, #14753, #6834 ) ;
#14188=ORIENTED_EDGE ( 'NONE', *, *, #10182, .T. ) ;
#14189=CYLINDRICAL_SURFACE ( 'NONE', #11673, 0.5000000000000004441 ) ;
#14190=EDGE_CURVE ( 'NONE', #14620, #9479, #3947, .T. ) ;
#14191=DIRECTION ( 'NONE',  ( 0.000000000000000000, 0.000000000000000000, 1.000000000000000000 ) ) ;
#14192=CARTESIAN_POINT ( 'NONE',  ( 0.000000000000000000, 0.000000000000000000, -10.50000000000000000 ) ) ;
#14193=VERTEX_POINT ( 'NONE', #9645 ) ;
#14196=CARTESIAN_POINT ( 'NONE',  ( -6.123233995736766085E-15, 100.0000000000000000, 8.000000000000000000 ) ) ;
#14197=ORIENTED_EDGE ( 'NONE', *, *, #12206, .T. ) ;
#14198=AXIS2_PLACEMENT_3D ( 'NONE', #8453, #14301, #13095 ) ;
#14199=DIRECTION ( 'NONE',  ( -0.000000000000000000, -0.000000000000000000, -1.000000000000000000 ) ) ;
#14200=AXIS2_PLACEMENT_3D ( 'NONE', #6437, #689, #14587 ) ;
#14201=EDGE_CURVE ( 'NONE', #5954, #8393, #6165, .T. ) ;
#14202=EDGE_CURVE ( 'NONE', #14329, #2988, #13892, .T. ) ;
#14204=ORIENTED_EDGE ( 'NONE', *, *, #12718, .F. ) ;
#14205=CIRCLE ( 'NONE', #1829, 0.5000000000000004441 ) ;
#14206=AXIS2_PLACEMENT_3D ( 'NONE', #6809, #8106, #13659 ) ;
#14210=CARTESIAN_POINT ( 'NONE',  ( 37.71449950291050612, -86.67575032682090352, 8.000000000000000000 ) ) ;
#14211=CARTESIAN_POINT ( 'NONE',  ( 97.00000000000000000, -3.384287605079545030E-13, -8.000000000000000000 ) ) ;
#14215=VERTEX_POINT ( 'NONE', #556 ) ;
#14216=AXIS2_PLACEMENT_3D ( 'NONE', #1851, #11268, #10042 ) ;
#14218=ORIENTED_EDGE ( 'NONE', *, *, #6193, .F. ) ;
#14219=DIRECTION ( 'NONE',  ( 1.000000000000000000, 0.000000000000000000, 0.000000000000000000 ) ) ;
#14221=CARTESIAN_POINT ( 'NONE',  ( 97.00000000000000000, -3.384287605079545030E-13, -13.00000000000000178 ) ) ;
#14223=VERTEX_POINT ( 'NONE', #10872 ) ;
#14224=VERTEX_POINT ( 'NONE', #5110 ) ;
#14225=EDGE_CURVE ( 'NONE', #7351, #1696, #13155, .T. ) ;
#14228=ORIENTED_EDGE ( 'NONE', *, *, #5414, .F. ) ;
#14229=LINE ( 'NONE', #555, #13342 ) ;
#14230=DIRECTION ( 'NONE',  ( 1.000000000000000000, 0.000000000000000000, 0.000000000000000000 ) ) ;
#14231=CARTESIAN_POINT ( 'NONE',  ( 0.000000000000000000, 0.000000000000000000, -10.50000000000000000 ) ) ;
#14232=DIRECTION ( 'NONE',  ( 1.000000000000000000, 0.000000000000000000, 0.000000000000000000 ) ) ;
#14234=VECTOR ( 'NONE', #6446, 1000.000000000000000 ) ;
#14238=EDGE_CURVE ( 'NONE', #12729, #4183, #1280, .T. ) ;
#14239=ORIENTED_EDGE ( 'NONE', *, *, #7960, .F. ) ;
#14241=EDGE_CURVE ( 'NONE', #13345, #6195, #2482, .T. ) ;
#14243=ORIENTED_EDGE ( 'NONE', *, *, #416, .F. ) ;
#14244=CARTESIAN_POINT ( 'NONE',  ( -24.99999999999973355, -43.30127018922208748, 8.000000000000000000 ) ) ;
#14246=DIRECTION ( 'NONE',  ( 0.000000000000000000, 0.000000000000000000, 1.000000000000000000 ) ) ;
#14248=EDGE_CURVE ( 'NONE', #218, #11004, #6830, .T. ) ;
#14250=VERTEX_POINT ( 'NONE', #3758 ) ;
#14251=ORIENTED_EDGE ( 'NONE', *, *, #8062, .F. ) ;
#14252=CYLINDRICAL_SURFACE ( 'NONE', #9563, 59.50000000000000000 ) ;
#14254=CARTESIAN_POINT ( 'NONE',  ( -41.54772703543551415, -32.26435573746212526, -10.50000000000000000 ) ) ;
#14257=DIRECTION ( 'NONE',  ( 0.000000000000000000, 0.000000000000000000, -1.000000000000000000 ) ) ;
#14260=EDGE_CURVE ( 'NONE', #2743, #6973, #6584, .T. ) ;
#14263=ORIENTED_EDGE ( 'NONE', *, *, #3505, .T. ) ;
#14265=CARTESIAN_POINT ( 'NONE',  ( 37.12029293941315444, -89.61631465359504034, 8.000000000000000000 ) ) ;
#14266=ORIENTED_EDGE ( 'NONE', *, *, #4179, .T. ) ;
#14267=CARTESIAN_POINT ( 'NONE',  ( 99.48933418828643482, -1.674280531759671620, -8.000000000000000000 ) ) ;
#14269=VERTEX_POINT ( 'NONE', #11260 ) ;
#14270=CARTESIAN_POINT ( 'NONE',  ( 0.2790467552932217044, -96.58511096861892042, 10.49999999999999822 ) ) ;
#14271=LINE ( 'NONE', #1379, #5682 ) ;
#14273=EDGE_CURVE ( 'NONE', #9052, #8417, #8303, .T. ) ;
#14274=EDGE_CURVE ( 'NONE', #10391, #7242, #2983, .T. ) ;
#14275=CARTESIAN_POINT ( 'NONE',  ( -1.674280531759324342, -99.48933418828643482, -13.00000000000000178 ) ) ;
#14278=CYLINDRICAL_SURFACE ( 'NONE', #7727, 63.00000000000000000 ) ;
#14279=ORIENTED_EDGE ( 'NONE', *, *, #11364, .T. ) ;
#14280=EDGE_LOOP ( 'NONE', ( #9578, #14018, #6226, #14366 ) ) ;
#14281=EDGE_CURVE ( 'NONE', #7029, #10986, #8741, .T. ) ;
#14282=LINE ( 'NONE', #5998, #7427 ) ;
#14283=AXIS2_PLACEMENT_3D ( 'NONE', #11, #2223, #11580 ) ;
#14285=DIRECTION ( 'NONE',  ( -0.000000000000000000, -0.000000000000000000, -1.000000000000000000 ) ) ;
#14286=DIRECTION ( 'NONE',  ( -1.000000000000000000, 6.399202155825555340E-14, 0.000000000000000000 ) ) ;
#14287=ORIENTED_EDGE ( 'NONE', *, *, #5827, .T. ) ;
#14288=CARTESIAN_POINT ( 'NONE',  ( 100.0000000000000000, 1.224646799147353217E-14, 13.00000000000000178 ) ) ;
#14290=ORIENTED_EDGE ( 'NONE', *, *, #14190, .T. ) ;
#14291=EDGE_CURVE ( 'NONE', #2928, #1483, #8777, .T. ) ;
#14293=FACE_OUTER_BOUND ( 'NONE', #11175, .T. ) ;
#14294=CARTESIAN_POINT ( 'NONE',  ( 1.674280531759324342, 99.48933418828643482, -13.00000000000000178 ) ) ;
#14299=ORIENTED_EDGE ( 'NONE', *, *, #2900, .F. ) ;
#14301=DIRECTION ( 'NONE',  ( 0.000000000000000000, 0.000000000000000000, -1.000000000000000000 ) ) ;
#14302=VECTOR ( 'NONE', #2951, 1000.000000000000000 ) ;
#14303=FACE_OUTER_BOUND ( 'NONE', #11479, .T. ) ;
#14305=CIRCLE ( 'NONE', #248, 56.99999999999999289 ) ;
#14306=VERTEX_POINT ( 'NONE', #1910 ) ;
#14307=DIRECTION ( 'NONE',  ( 0.000000000000000000, 0.000000000000000000, -1.000000000000000000 ) ) ;
#14309=CYLINDRICAL_SURFACE ( 'NONE', #8842, 3.000000000000002665 ) ;
#14315=AXIS2_PLACEMENT_3D ( 'NONE', #10563, #4728, #12549 ) ;
#14316=ORIENTED_EDGE ( 'NONE', *, *, #12268, .F. ) ;
#14319=CARTESIAN_POINT ( 'NONE',  ( 0.000000000000000000, 0.000000000000000000, -10.50000000000000000 ) ) ;
#14321=CARTESIAN_POINT ( 'NONE',  ( 52.83493649053890806, -6.470413585629217057E-15, -11.74999999999999822 ) ) ;
#14323=CIRCLE ( 'NONE', #8047, 3.000000000000002665 ) ;
#14324=CIRCLE ( 'NONE', #12874, 63.00000000000000000 ) ;
#14326=DIRECTION ( 'NONE',  ( 0.000000000000000000, 0.000000000000000000, 1.000000000000000000 ) ) ;
#14327=ADVANCED_FACE ( 'NONE', ( #867 ), #9041, .F. ) ;
#14328=CIRCLE ( 'NONE', #7780, 100.0000000000000000 ) ;
#14329=VERTEX_POINT ( 'NONE', #4352 ) ;
#14331=DIRECTION ( 'NONE',  ( 1.000000000000000000, 0.000000000000000000, 0.000000000000000000 ) ) ;
#14332=DIRECTION ( 'NONE',  ( 1.000000000000000000, 0.000000000000000000, 0.000000000000000000 ) ) ;
#14334=SURFACE_SIDE_STYLE ('',( #149 ) ) ;
#14336=CIRCLE ( 'NONE', #2700, 56.99999999999999289 ) ;
#14337=DIRECTION ( 'NONE',  ( 0.000000000000000000, 0.000000000000000000, 1.000000000000000000 ) ) ;
#14338=ORIENTED_EDGE ( 'NONE', *, *, #5009, .T. ) ;
#14341=DIRECTION ( 'NONE',  ( -0.000000000000000000, -0.000000000000000000, -1.000000000000000000 ) ) ;
#14342=AXIS2_PLACEMENT_3D ( 'NONE', #3600, #3451, #12854 ) ;
#14343=VERTEX_POINT ( 'NONE', #12397 ) ;
#14344=EDGE_LOOP ( 'NONE', ( #9146, #14555, #11780, #5529 ) ) ;
#14345=CARTESIAN_POINT ( 'NONE',  ( 49.00442420935993226, -30.80502811811213704, -13.00000000000000178 ) ) ;
#14346=CIRCLE ( 'NONE', #11460, 59.50000000000000711 ) ;
#14348=CIRCLE ( 'NONE', #11465, 3.000000000000002665 ) ;
#14350=CARTESIAN_POINT ( 'NONE',  ( -45.96504489225991819, 23.50071946824089153, 8.000000000000000000 ) ) ;
#14351=CARTESIAN_POINT ( 'NONE',  ( -99.48933418828642061, 1.674280531760365065, 8.000000000000000000 ) ) ;
#14352=CARTESIAN_POINT ( 'NONE',  ( -6.852625091552704717, -52.05085522212505111, -10.50000000000000000 ) ) ;
#14353=ORIENTED_EDGE ( 'NONE', *, *, #2825, .F. ) ;
#14354=CYLINDRICAL_SURFACE ( 'NONE', #3180, 3.000000000000002665 ) ;
#14356=DIRECTION ( 'NONE',  ( 0.000000000000000000, 0.000000000000000000, 1.000000000000000000 ) ) ;
#14357=DIRECTION ( 'NONE',  ( -1.000000000000000000, 1.765157221169382734E-15, 0.000000000000000000 ) ) ;
#14358=EDGE_CURVE ( 'NONE', #8214, #8032, #3457, .T. ) ;
#14362=CARTESIAN_POINT ( 'NONE',  ( 52.54657765281197612, -6.917888187662545540, -10.50000000000000000 ) ) ;
#14363=ORIENTED_EDGE ( 'NONE', *, *, #10575, .T. ) ;
#14365=EDGE_CURVE ( 'NONE', #10761, #5962, #1524, .T. ) ;
#14366=ORIENTED_EDGE ( 'NONE', *, *, #14713, .F. ) ;
#14367=DIRECTION ( 'NONE',  ( 1.000000000000000000, 0.000000000000000000, 0.000000000000000000 ) ) ;
#14368=EDGE_LOOP ( 'NONE', ( #8889, #2537, #14121, #8831 ) ) ;
#14369=CIRCLE ( 'NONE', #2969, 3.000000000000002665 ) ;
#14370=DIRECTION ( 'NONE',  ( 1.000000000000000000, 0.000000000000000000, 0.000000000000000000 ) ) ;
#14372=ADVANCED_FACE ( 'NONE', ( #6605 ), #5489, .F. ) ;
#14373=DIRECTION ( 'NONE',  ( -1.000000000000000000, 2.682261509073382730E-15, 0.000000000000000000 ) ) ;
#14374=DIRECTION ( 'NONE',  ( 1.000000000000000000, 0.000000000000000000, 0.000000000000000000 ) ) ;
#14375=CYLINDRICAL_SURFACE ( 'NONE', #5853, 2.649999999999993694 ) ;
#14377=EDGE_LOOP ( 'NONE', ( #7677, #11986, #716, #10360, #11850 ) ) ;
#14378=CARTESIAN_POINT ( 'NONE',  ( 0.000000000000000000, 0.000000000000000000, 10.50000000000000000 ) ) ;
#14379=FACE_OUTER_BOUND ( 'NONE', #731, .T. ) ;
#14380=AXIS2_PLACEMENT_3D ( 'NONE', #9972, #14763, #8903 ) ;
#14381=ADVANCED_FACE ( 'NONE', ( #10113 ), #13382, .T. ) ;
#14382=CARTESIAN_POINT ( 'NONE',  ( -38.26834323650768255, 92.38795325112920409, -8.000000000000000000 ) ) ;
#14383=CIRCLE ( 'NONE', #12203, 60.49999999999999289 ) ;
#14385=ORIENTED_EDGE ( 'NONE', *, *, #5535, .F. ) ;
#14387=CIRCLE ( 'NONE', #5428, 56.99999999999999289 ) ;
#14388=ORIENTED_EDGE ( 'NONE', *, *, #1665, .T. ) ;
#14392=DIRECTION ( 'NONE',  ( 1.000000000000000000, 0.000000000000000000, 0.000000000000000000 ) ) ;
#14395=CARTESIAN_POINT ( 'NONE',  ( 97.50000000000000000, -3.384287605079545030E-13, 10.49999999999999822 ) ) ;
#14396=ORIENTED_EDGE ( 'NONE', *, *, #12705, .F. ) ;
#14397=AXIS2_PLACEMENT_3D ( 'NONE', #13702, #7918, #7986 ) ;
#14399=CYLINDRICAL_SURFACE ( 'NONE', #3019, 63.00000000000000000 ) ;
#14400=AXIS2_PLACEMENT_3D ( 'NONE', #640, #13464, #12327 ) ;
#14401=DIRECTION ( 'NONE',  ( 0.000000000000000000, 0.000000000000000000, 1.000000000000000000 ) ) ;
#14402=ORIENTED_EDGE ( 'NONE', *, *, #1460, .T. ) ;
#14403=VERTEX_POINT ( 'NONE', #14829 ) ;
#14405=EDGE_LOOP ( 'NONE', ( #4088, #1173, #6926, #7801, #14156, #1552, #14363, #12275, #6105 ) ) ;
#14406=EDGE_CURVE ( 'NONE', #4070, #297, #805, .T. ) ;
#14407=AXIS2_PLACEMENT_3D ( 'NONE', #5813, #9091, #3625 ) ;
#14408=AXIS2_PLACEMENT_3D ( 'NONE', #5661, #11528, #1408 ) ;
#14409=AXIS2_PLACEMENT_3D ( 'NONE', #9541, #14191, #14332 ) ;
#14410=CARTESIAN_POINT ( 'NONE',  ( 68.58935777509475429, -68.58935777509547904, -13.00000000000000178 ) ) ;
#14412=LINE ( 'NONE', #10767, #6634 ) ;
#14413=ORIENTED_EDGE ( 'NONE', *, *, #11980, .T. ) ;
#14414=CYLINDRICAL_SURFACE ( 'NONE', #3183, 3.000000000000002665 ) ;
#14415=FACE_OUTER_BOUND ( 'NONE', #8980, .T. ) ;
#14416=VERTEX_POINT ( 'NONE', #6459 ) ;
#14417=CARTESIAN_POINT ( 'NONE',  ( 56.43380494353997534, 12.86891638962136319, 8.000000000000000000 ) ) ;
#14418=AXIS2_PLACEMENT_3D ( 'NONE', #6923, #10418, #4583 ) ;
#14419=CIRCLE ( 'NONE', #3514, 3.000000000000002665 ) ;
#14420=ORIENTED_EDGE ( 'NONE', *, *, #14844, .T. ) ;
#14421=AXIS2_PLACEMENT_3D ( 'NONE', #12774, #5847, #5769 ) ;
#14422=ORIENTED_EDGE ( 'NONE', *, *, #7072, .T. ) ;
#14424=ORIENTED_EDGE ( 'NONE', *, *, #3665, .T. ) ;
#14425=EDGE_CURVE ( 'NONE', #14021, #13716, #4431, .T. ) ;
#14426=ADVANCED_FACE ( 'NONE', ( #1772 ), #6378, .T. ) ;
#14427=CYLINDRICAL_SURFACE ( 'NONE', #4855, 3.000000000000002665 ) ;
#14431=DIRECTION ( 'NONE',  ( 0.000000000000000000, 0.000000000000000000, 1.000000000000000000 ) ) ;
#14433=CIRCLE ( 'NONE', #1343, 3.000000000000002665 ) ;
#14434=CIRCLE ( 'NONE', #14421, 0.5000000000000004441 ) ;
#14436=EDGE_LOOP ( 'NONE', ( #2678, #612, #102, #10306, #6691, #13631 ) ) ;
#14438=CARTESIAN_POINT ( 'NONE',  ( -50.71110588017612741, -13.58799986788221226, -10.50000000000000000 ) ) ;
#14439=DIRECTION ( 'NONE',  ( 0.000000000000000000, 0.000000000000000000, 1.000000000000000000 ) ) ;
#14441=CIRCLE ( 'NONE', #6918, 0.5000000000000004441 ) ;
#14442=ORIENTED_EDGE ( 'NONE', *, *, #131, .T. ) ;
#14443=DIRECTION ( 'NONE',  ( -0.000000000000000000, -0.000000000000000000, 1.000000000000000000 ) ) ;
#14444=ORIENTED_EDGE ( 'NONE', *, *, #1529, .F. ) ;
#14446=VERTEX_POINT ( 'NONE', #2293 ) ;
#14447=LINE ( 'NONE', #3974, #2912 ) ;
#14448=VERTEX_POINT ( 'NONE', #6914 ) ;
#14449=DIRECTION ( 'NONE',  ( -1.000000000000000000, 0.000000000000000000, 0.000000000000000000 ) ) ;
#14451=CARTESIAN_POINT ( 'NONE',  ( 0.000000000000000000, 0.000000000000000000, 8.000000000000000000 ) ) ;
#14453=CARTESIAN_POINT ( 'NONE',  ( -13.71740939043329277, 51.19406879332069593, 8.000000000000000000 ) ) ;
#14456=DIRECTION ( 'NONE',  ( -1.000000000000000000, 0.000000000000000000, 0.000000000000000000 ) ) ;
#14458=ORIENTED_EDGE ( 'NONE', *, *, #647, .T. ) ;
#14463=ADVANCED_FACE ( 'NONE', ( #13769 ), #3588, .F. ) ;
#14465=ORIENTED_EDGE ( 'NONE', *, *, #2626, .F. ) ;
#14466=CARTESIAN_POINT ( 'NONE',  ( -47.21331623427138879, -33.48561063518577896, -10.50000000000000000 ) ) ;
#14467=ORIENTED_EDGE ( 'NONE', *, *, #7580, .T. ) ;
#14468=AXIS2_PLACEMENT_3D ( 'NONE', #6421, #3027, #5453 ) ;
#14469=LINE ( 'NONE', #7464, #12971 ) ;
#14470=DIRECTION ( 'NONE',  ( 1.000000000000000000, 0.000000000000000000, -0.000000000000000000 ) ) ;
#14473=ADVANCED_FACE ( 'NONE', ( #8135 ), #5707, .T. ) ;
#14474=CARTESIAN_POINT ( 'NONE',  ( -44.79355920668832880, -31.05588327715819474, -8.000000000000000000 ) ) ;
#14476=CIRCLE ( 'NONE', #7916, 2.649999999999993694 ) ;
#14477=ORIENTED_EDGE ( 'NONE', *, *, #14758, .T. ) ;
#14478=ORIENTED_EDGE ( 'NONE', *, *, #7008, .T. ) ;
#14479=DIRECTION ( 'NONE',  ( 0.000000000000000000, 0.000000000000000000, -1.000000000000000000 ) ) ;
#14481=DIRECTION ( 'NONE',  ( -1.000000000000000000, 0.000000000000000000, 0.000000000000000000 ) ) ;
#14482=ORIENTED_EDGE ( 'NONE', *, *, #6481, .T. ) ;
#14484=ORIENTED_EDGE ( 'NONE', *, *, #13833, .T. ) ;
#14486=VERTEX_POINT ( 'NONE', #2430 ) ;
#14487=LINE ( 'NONE', #11141, #2294 ) ;
#14488=DIRECTION ( 'NONE',  ( 1.000000000000000000, 0.000000000000000000, 0.000000000000000000 ) ) ;
#14490=ORIENTED_EDGE ( 'NONE', *, *, #14789, .T. ) ;
#14492=DIRECTION ( 'NONE',  ( 1.000000000000000000, 0.000000000000000000, 0.000000000000000000 ) ) ;
#14494=LINE ( 'NONE', #7514, #5087 ) ;
#14496=ORIENTED_EDGE ( 'NONE', *, *, #4975, .T. ) ;
#14497=VERTEX_POINT ( 'NONE', #1013 ) ;
#14499=PLANE ( 'NONE',  #6052 ) ;
#14500=VECTOR ( 'NONE', #9313, 1000.000000000000000 ) ;
#14501=DIRECTION ( 'NONE',  ( -0.000000000000000000, -0.000000000000000000, -1.000000000000000000 ) ) ;
#14503=DIRECTION ( 'NONE',  ( -0.000000000000000000, -0.000000000000000000, -1.000000000000000000 ) ) ;
#14504=DIRECTION ( 'NONE',  ( -1.000000000000000000, 0.000000000000000000, 0.000000000000000000 ) ) ;
#14505=ORIENTED_EDGE ( 'NONE', *, *, #5748, .T. ) ;
#14506=EDGE_CURVE ( 'NONE', #2940, #219, #11961, .T. ) ;
#14507=CARTESIAN_POINT ( 'NONE',  ( 37.71449950291050612, -86.67575032682090352, -13.00000000000000178 ) ) ;
#14512=LINE ( 'NONE', #7440, #11327 ) ;
#14514=VERTEX_POINT ( 'NONE', #5628 ) ;
#14516=ORIENTED_EDGE ( 'NONE', *, *, #14716, .T. ) ;
#14518=VERTEX_POINT ( 'NONE', #164 ) ;
#14520=ORIENTED_EDGE ( 'NONE', *, *, #3292, .F. ) ;
#14521=FACE_OUTER_BOUND ( 'NONE', #11123, .T. ) ;
#14523=DIRECTION ( 'NONE',  ( 0.000000000000000000, 0.000000000000000000, 1.000000000000000000 ) ) ;
#14524=FACE_OUTER_BOUND ( 'NONE', #5917, .T. ) ;
#14527=AXIS2_PLACEMENT_3D ( 'NONE', #13440, #13365, #7891 ) ;
#14529=ORIENTED_EDGE ( 'NONE', *, *, #1246, .F. ) ;
#14531=DIRECTION ( 'NONE',  ( 1.000000000000000000, 0.000000000000000000, 0.000000000000000000 ) ) ;
#14532=FACE_OUTER_BOUND ( 'NONE', #11509, .T. ) ;
#14533=CARTESIAN_POINT ( 'NONE',  ( 89.61631465359491244, 37.12029293941346708, -13.00000000000000178 ) ) ;
#14536=AXIS2_PLACEMENT_3D ( 'NONE', #2432, #11715, #8136 ) ;
#14537=VERTEX_POINT ( 'NONE', #4650 ) ;
#14538=DIRECTION ( 'NONE',  ( 0.000000000000000000, 0.000000000000000000, 1.000000000000000000 ) ) ;
#14541=CARTESIAN_POINT ( 'NONE',  ( -52.54657765281192638, 6.917888187662934563, 10.49999999999999822 ) ) ;
#14542=DIRECTION ( 'NONE',  ( -0.000000000000000000, -0.000000000000000000, -1.000000000000000000 ) ) ;
#14547=CIRCLE ( 'NONE', #983, 0.5000000000000004441 ) ;
#14548=ORIENTED_EDGE ( 'NONE', *, *, #1951, .T. ) ;
#14551=CIRCLE ( 'NONE', #4605, 0.5000000000000004441 ) ;
#14552=CARTESIAN_POINT ( 'NONE',  ( 0.000000000000000000, 0.000000000000000000, 8.000000000000000000 ) ) ;
#14553=AXIS2_PLACEMENT_3D ( 'NONE', #4336, #7583, #690 ) ;
#14554=FACE_OUTER_BOUND ( 'NONE', #2872, .T. ) ;
#14555=ORIENTED_EDGE ( 'NONE', *, *, #5816, .T. ) ;
#14556=EDGE_CURVE ( 'NONE', #14416, #8471, #13922, .T. ) ;
#14560=ORIENTED_EDGE ( 'NONE', *, *, #5819, .T. ) ;
#14561=AXIS2_PLACEMENT_3D ( 'NONE', #9932, #10012, #7805 ) ;
#14562=ADVANCED_FACE ( 'NONE', ( #4950 ), #1674, .F. ) ;
#14563=CIRCLE ( 'NONE', #745, 59.50000000000000000 ) ;
#14564=DIRECTION ( 'NONE',  ( 0.000000000000000000, 0.000000000000000000, -1.000000000000000000 ) ) ;
#14565=AXIS2_PLACEMENT_3D ( 'NONE', #12324, #4286, #5555 ) ;
#14566=CONICAL_SURFACE ( 'NONE', #3903, 52.83493649053890806, 0.5235987755983000369 ) ;
#14567=DIRECTION ( 'NONE',  ( 0.000000000000000000, 0.000000000000000000, -1.000000000000000000 ) ) ;
#14568=LINE ( 'NONE', #13422, #9849 ) ;
#14570=EDGE_LOOP ( 'NONE', ( #7209, #6293 ) ) ;
#14571=DIRECTION ( 'NONE',  ( 1.000000000000000000, 0.000000000000000000, 0.000000000000000000 ) ) ;
#14572=CARTESIAN_POINT ( 'NONE',  ( -55.00000000000000000, 0.000000000000000000, -13.00000000000000178 ) ) ;
#14573=ORIENTED_EDGE ( 'NONE', *, *, #1477, .F. ) ;
#14574=AXIS2_PLACEMENT_3D ( 'NONE', #13073, #2821, #5093 ) ;
#14577=ORIENTED_EDGE ( 'NONE', *, *, #7217, .T. ) ;
#14578=AXIS2_PLACEMENT_3D ( 'NONE', #5706, #4794, #7974 ) ;
#14579=EDGE_CURVE ( 'NONE', #1620, #5520, #6531, .T. ) ;
#14580=AXIS2_PLACEMENT_3D ( 'NONE', #11972, #11053, #2919 ) ;
#14582=CARTESIAN_POINT ( 'NONE',  ( 68.09867107462983427, 68.49330278050145182, -13.00000000000000178 ) ) ;
#14584=CIRCLE ( 'NONE', #10689, 3.000000000000002665 ) ;
#14587=DIRECTION ( 'NONE',  ( 1.000000000000000000, 0.000000000000000000, 0.000000000000000000 ) ) ;
#14588=CYLINDRICAL_SURFACE ( 'NONE', #14063, 0.5000000000000022204 ) ;
#14589=AXIS2_PLACEMENT_3D ( 'NONE', #13362, #7582, #14786 ) ;
#14591=CIRCLE ( 'NONE', #2952, 50.00000000000000000 ) ;
#14592=ORIENTED_EDGE ( 'NONE', *, *, #5067, .F. ) ;
#14597=CARTESIAN_POINT ( 'NONE',  ( -6.526309611002575117, -49.57224306869051844, -8.000000000000000000 ) ) ;
#14598=ORIENTED_EDGE ( 'NONE', *, *, #12649, .T. ) ;
#14599=CARTESIAN_POINT ( 'NONE',  ( 42.64958156413651835, 32.39328945492032830, -10.50000000000000000 ) ) ;
#14601=CIRCLE ( 'NONE', #6333, 59.50000000000000711 ) ;
#14602=EDGE_LOOP ( 'NONE', ( #281, #1271, #9625, #4026 ) ) ;
#14603=PLANE ( 'NONE',  #9936 ) ;
#14604=EDGE_CURVE ( 'NONE', #8687, #8824, #2905, .T. ) ;
#14605=EDGE_LOOP ( 'NONE', ( #3350, #14854, #12675, #9228 ) ) ;
#14606=DIRECTION ( 'NONE',  ( 0.000000000000000000, 0.000000000000000000, 1.000000000000000000 ) ) ;
#14607=DIRECTION ( 'NONE',  ( 1.000000000000000000, 0.000000000000000000, -0.000000000000000000 ) ) ;
#14608=EDGE_CURVE ( 'NONE', #11469, #13059, #14804, .T. ) ;
#14609=CARTESIAN_POINT ( 'NONE',  ( -12.86891638962156215, 56.43380494353993271, 10.49999999999999822 ) ) ;
#14610=EDGE_CURVE ( 'NONE', #6323, #14678, #9439, .T. ) ;
#14611=AXIS2_PLACEMENT_3D ( 'NONE', #10021, #3121, #3052 ) ;
#14612=CARTESIAN_POINT ( 'NONE',  ( 57.06275842387049835, -9.706953719245678514, -10.50000000000000000 ) ) ;
#14613=CARTESIAN_POINT ( 'NONE',  ( -29.26435573746199381, 42.04772703543562073, -8.000000000000000000 ) ) ;
#14615=VERTEX_POINT ( 'NONE', #14351 ) ;
#14616=AXIS2_PLACEMENT_3D ( 'NONE', #6527, #14686, #5556 ) ;
#14618=CARTESIAN_POINT ( 'NONE',  ( 0.000000000000000000, 0.000000000000000000, 8.000000000000000000 ) ) ;
#14619=AXIS2_PLACEMENT_3D ( 'NONE', #2844, #10879, #9435 ) ;
#14620=VERTEX_POINT ( 'NONE', #13224 ) ;
#14622=ORIENTED_EDGE ( 'NONE', *, *, #2965, .T. ) ;
#14624=DIRECTION ( 'NONE',  ( 1.000000000000000000, 0.000000000000000000, 0.000000000000000000 ) ) ;
#14625=EDGE_CURVE ( 'NONE', #13141, #8687, #3400, .T. ) ;
#14626=CARTESIAN_POINT ( 'NONE',  ( 0.000000000000000000, 0.000000000000000000, -8.000000000000000000 ) ) ;
#14627=EDGE_CURVE ( 'NONE', #14878, #8252, #3648, .T. ) ;
#14628=CARTESIAN_POINT ( 'NONE',  ( -100.0000000000000000, 1.090307039623097308E-12, -8.000000000000000000 ) ) ;
#14629=DIRECTION ( 'NONE',  ( 1.000000000000000000, 0.000000000000000000, 0.000000000000000000 ) ) ;
#14632=ORIENTED_EDGE ( 'NONE', *, *, #9078, .T. ) ;
#14633=AXIS2_PLACEMENT_3D ( 'NONE', #3076, #13539, #10044 ) ;
#14634=CARTESIAN_POINT ( 'NONE',  ( -37.53686968382306333, -89.89283556784496909, -10.50000000000000000 ) ) ;
#14636=CYLINDRICAL_SURFACE ( 'NONE', #11736, 57.00000000000000000 ) ;
#14638=VECTOR ( 'NONE', #749, 1000.000000000000000 ) ;
#14639=ORIENTED_EDGE ( 'NONE', *, *, #8696, .F. ) ;
#14640=ORIENTED_EDGE ( 'NONE', *, *, #2642, .F. ) ;
#14644=( LENGTH_UNIT ( ) NAMED_UNIT ( * ) SI_UNIT ( .MILLI., .METRE. ) );
#14645=DIRECTION ( 'NONE',  ( 1.000000000000000000, 0.000000000000000000, 0.000000000000000000 ) ) ;
#14646=CARTESIAN_POINT ( 'NONE',  ( 0.000000000000000000, 0.000000000000000000, -8.000000000000000000 ) ) ;
#14647=CARTESIAN_POINT ( 'NONE',  ( -26.49999999999971578, -45.89934640057541060, 10.49999999999999822 ) ) ;
#14648=EDGE_CURVE ( 'NONE', #13160, #13122, #11400, .T. ) ;
#14650=PLANE ( 'NONE',  #12605 ) ;
#14651=EDGE_LOOP ( 'NONE', ( #11901, #10517, #11060, #7901, #2157 ) ) ;
#14653=EDGE_LOOP ( 'NONE', ( #8105, #4282, #523, #8354 ) ) ;
#14654=ORIENTED_EDGE ( 'NONE', *, *, #10182, .F. ) ;
#14656=VECTOR ( 'NONE', #547, 1000.000000000000000 ) ;
#14658=ADVANCED_FACE ( 'NONE', ( #6067 ), #2660, .T. ) ;
#14661=PLANE ( 'NONE',  #8370 ) ;
#14662=CARTESIAN_POINT ( 'NONE',  ( 37.71449950291050612, -86.67575032682090352, -8.000000000000000000 ) ) ;
#14663=EDGE_CURVE ( 'NONE', #4331, #7416, #737, .T. ) ;
#14664=DIRECTION ( 'NONE',  ( 1.000000000000000000, 0.000000000000000000, 0.000000000000000000 ) ) ;
#14666=ORIENTED_EDGE ( 'NONE', *, *, #7637, .T. ) ;
#14667=AXIS2_PLACEMENT_3D ( 'NONE', #3009, #11908, #1500 ) ;
#14668=AXIS2_PLACEMENT_3D ( 'NONE', #12669, #12587, #8101 ) ;
#14670=AXIS2_PLACEMENT_3D ( 'NONE', #968, #12512, #10519 ) ;
#14671=CARTESIAN_POINT ( 'NONE',  ( 3.000000000000004885, -97.00000000000000000, -13.00000000000000178 ) ) ;
#14672=FACE_OUTER_BOUND ( 'NONE', #856, .T. ) ;
#14673=ORIENTED_EDGE ( 'NONE', *, *, #7753, .F. ) ;
#14674=( NAMED_UNIT ( * ) SI_UNIT ( $, .STERADIAN. ) SOLID_ANGLE_UNIT ( ) );
#14676=AXIS2_PLACEMENT_3D ( 'NONE', #436, #5064, #4364 ) ;
#14678=VERTEX_POINT ( 'NONE', #10629 ) ;
#14679=CIRCLE ( 'NONE', #10548, 3.000000000000002665 ) ;
#14681=AXIS2_PLACEMENT_3D ( 'NONE', #7518, #12172, #14022 ) ;
#14682=EDGE_LOOP ( 'NONE', ( #12483, #10803, #3399, #10977, #8814, #472 ) ) ;
#14683=ORIENTED_EDGE ( 'NONE', *, *, #3943, .T. ) ;
#14684=DIRECTION ( 'NONE',  ( -0.000000000000000000, -0.000000000000000000, -1.000000000000000000 ) ) ;
#14685=CYLINDRICAL_SURFACE ( 'NONE', #10668, 60.50000000000000000 ) ;
#14686=DIRECTION ( 'NONE',  ( 0.000000000000000000, 0.000000000000000000, 1.000000000000000000 ) ) ;
#14687=DIRECTION ( 'NONE',  ( 1.000000000000000000, 0.000000000000000000, 0.000000000000000000 ) ) ;
#14689=DIRECTION ( 'NONE',  ( 0.000000000000000000, 0.000000000000000000, 1.000000000000000000 ) ) ;
#14690=CIRCLE ( 'NONE', #13466, 0.5000000000000004441 ) ;
#14692=LINE ( 'NONE', #7527, #9591 ) ;
#14693=CYLINDRICAL_SURFACE ( 'NONE', #838, 0.5000000000000004441 ) ;
#14694=CIRCLE ( 'NONE', #11299, 56.99999999999998579 ) ;
#14695=DIRECTION ( 'NONE',  ( 0.000000000000000000, 0.000000000000000000, 1.000000000000000000 ) ) ;
#14698=CARTESIAN_POINT ( 'NONE',  ( 26.49999999999971578, 45.89934640057541060, -10.50000000000000000 ) ) ;
#14699=AXIS2_PLACEMENT_3D ( 'NONE', #2955, #12077, #5305 ) ;
#14700=EDGE_LOOP ( 'NONE', ( #1242, #4681, #4199, #7572, #8244, #7644 ) ) ;
#14702=CARTESIAN_POINT ( 'NONE',  ( -20.00000000000000000, 0.000000000000000000, 13.00000000000000178 ) ) ;
#14704=DIRECTION ( 'NONE',  ( 1.000000000000000000, 0.000000000000000000, 0.000000000000000000 ) ) ;
#14705=DIRECTION ( 'NONE',  ( 1.000000000000000000, 0.000000000000000000, 0.000000000000000000 ) ) ;
#14707=ORIENTED_EDGE ( 'NONE', *, *, #5739, .T. ) ;
#14708=ORIENTED_EDGE ( 'NONE', *, *, #3721, .F. ) ;
#14709=ORIENTED_EDGE ( 'NONE', *, *, #3799, .F. ) ;
#14710=AXIS2_PLACEMENT_3D ( 'NONE', #13719, #7932, #15006 ) ;
#14711=DIRECTION ( 'NONE',  ( 1.000000000000000000, 0.000000000000000000, 0.000000000000000000 ) ) ;
#14712=FACE_OUTER_BOUND ( 'NONE', #4606, .T. ) ;
#14713=EDGE_CURVE ( 'NONE', #8537, #14933, #3738, .T. ) ;
#14714=DIRECTION ( 'NONE',  ( 0.000000000000000000, 0.000000000000000000, 1.000000000000000000 ) ) ;
#14716=EDGE_CURVE ( 'NONE', #9289, #8417, #5246, .T. ) ;
#14717=EDGE_LOOP ( 'NONE', ( #14338, #9275, #2158, #14573 ) ) ;
#14718=VERTEX_POINT ( 'NONE', #7730 ) ;
#14719=ORIENTED_EDGE ( 'NONE', *, *, #2626, .T. ) ;
#14720=AXIS2_PLACEMENT_3D ( 'NONE', #2300, #13773, #5638 ) ;
#14723=CARTESIAN_POINT ( 'NONE',  ( 91.27544013909738396, -39.61975340586589311, -8.000000000000000000 ) ) ;
#14726=CARTESIAN_POINT ( 'NONE',  ( 49.00442420935993226, -30.80502811811213704, -10.50000000000000000 ) ) ;
#14732=EDGE_LOOP ( 'NONE', ( #10031, #14420, #10717, #13281, #4378 ) ) ;
#14733=EDGE_LOOP ( 'NONE', ( #6428, #13129, #13170, #14769, #4564, #3474, #7709, #12560, #1281, #1375 ) ) ;
#14735=EDGE_CURVE ( 'NONE', #9586, #14514, #11322, .T. ) ;
#14736=DIRECTION ( 'NONE',  ( 0.000000000000000000, 0.000000000000000000, -1.000000000000000000 ) ) ;
#14737=UNCERTAINTY_MEASURE_WITH_UNIT (LENGTH_MEASURE( 1.000000000000000082E-05 ), #3058, 'distance_accuracy_value', 'NONE');
#14739=CARTESIAN_POINT ( 'NONE',  ( -71.53347797788819662, -69.16568774265570596, -13.00000000000000178 ) ) ;
#14742=FACE_OUTER_BOUND ( 'NONE', #3105, .T. ) ;
#14745=ORIENTED_EDGE ( 'NONE', *, *, #7488, .T. ) ;
#14746=CARTESIAN_POINT ( 'NONE',  ( 0.000000000000000000, 0.000000000000000000, -10.50000000000000000 ) ) ;
#14747=ORIENTED_EDGE ( 'NONE', *, *, #11866, .F. ) ;
#14748=EDGE_CURVE ( 'NONE', #5824, #9024, #2178, .T. ) ;
#14749=DIRECTION ( 'NONE',  ( 0.000000000000000000, 0.000000000000000000, -1.000000000000000000 ) ) ;
#14750=ADVANCED_FACE ( 'NONE', ( #4266 ), #1750, .T. ) ;
#14751=ORIENTED_EDGE ( 'NONE', *, *, #1309, .T. ) ;
#14752=CARTESIAN_POINT ( 'NONE',  ( 1.674280531759317014, -94.51066581171355097, -8.000000000000000000 ) ) ;
#14753=DIRECTION ( 'NONE',  ( 0.000000000000000000, 0.000000000000000000, 1.000000000000000000 ) ) ;
#14755=CARTESIAN_POINT ( 'NONE',  ( -57.06275842387042729, 9.706953719246069312, -13.00000000000000178 ) ) ;
#14756=DIRECTION ( 'NONE',  ( 0.000000000000000000, 0.000000000000000000, 1.000000000000000000 ) ) ;
#14757=CARTESIAN_POINT ( 'NONE',  ( 9.706953719245472456, 57.06275842387054098, -10.50000000000000000 ) ) ;
#14758=EDGE_CURVE ( 'NONE', #13178, #9373, #4127, .T. ) ;
#14759=CARTESIAN_POINT ( 'NONE',  ( -13.71740939043329277, 51.19406879332069593, 10.49999999999999822 ) ) ;
#14760=ORIENTED_EDGE ( 'NONE', *, *, #1396, .T. ) ;
#14761=LINE ( 'NONE', #10348, #2591 ) ;
#14763=DIRECTION ( 'NONE',  ( 0.000000000000000000, 0.000000000000000000, -1.000000000000000000 ) ) ;
#14764=AXIS2_PLACEMENT_3D ( 'NONE', #14895, #1218, #8046 ) ;
#14765=DIRECTION ( 'NONE',  ( 0.000000000000000000, 0.000000000000000000, 1.000000000000000000 ) ) ;
#14766=ADVANCED_FACE ( 'NONE', ( #12156 ), #14588, .F. ) ;
#14769=ORIENTED_EDGE ( 'NONE', *, *, #6467, .T. ) ;
#14770=CARTESIAN_POINT ( 'NONE',  ( -68.68541276968778675, 69.08004447556137961, 10.49999999999999822 ) ) ;
#14771=DIRECTION ( 'NONE',  ( 0.000000000000000000, 0.000000000000000000, -1.000000000000000000 ) ) ;
#14773=CARTESIAN_POINT ( 'NONE',  ( 0.000000000000000000, 0.000000000000000000, -10.50000000000000000 ) ) ;
#14775=ORIENTED_EDGE ( 'NONE', *, *, #5632, .F. ) ;
#14776=ORIENTED_EDGE ( 'NONE', *, *, #3505, .F. ) ;
#14778=DIRECTION ( 'NONE',  ( -1.000000000000000000, 0.000000000000000000, 0.000000000000000000 ) ) ;
#14780=VERTEX_POINT ( 'NONE', #8717 ) ;
#14782=ORIENTED_EDGE ( 'NONE', *, *, #2830, .T. ) ;
#14783=EDGE_LOOP ( 'NONE', ( #10969, #3313, #13972, #3377, #8605 ) ) ;
#14784=FACE_OUTER_BOUND ( 'NONE', #13006, .T. ) ;
#14786=DIRECTION ( 'NONE',  ( 1.000000000000000000, 0.000000000000000000, 0.000000000000000000 ) ) ;
#14789=EDGE_CURVE ( 'NONE', #6138, #1696, #4620, .T. ) ;
#14790=CARTESIAN_POINT ( 'NONE',  ( -29.49928053175900899, -45.83364790889059037, -13.00000000000000178 ) ) ;
#14791=CIRCLE ( 'NONE', #12357, 50.00000000000000000 ) ;
#14792=EDGE_CURVE ( 'NONE', #6859, #1107, #2962, .T. ) ;
#14793=CARTESIAN_POINT ( 'NONE',  ( 89.33979373934423052, -36.70371619500547666, -10.50000000000000000 ) ) ;
#14794=DIRECTION ( 'NONE',  ( 1.000000000000000000, 8.521448653921158262E-16, 0.000000000000000000 ) ) ;
#14795=VERTEX_POINT ( 'NONE', #14662 ) ;
#14796=ORIENTED_EDGE ( 'NONE', *, *, #5737, .T. ) ;
#14799=CIRCLE ( 'NONE', #9927, 100.0000000000000000 ) ;
#14800=ORIENTED_EDGE ( 'NONE', *, *, #3671, .F. ) ;
#14801=CARTESIAN_POINT ( 'NONE',  ( 0.000000000000000000, 0.000000000000000000, 8.000000000000000000 ) ) ;
#14802=AXIS2_PLACEMENT_3D ( 'NONE', #3308, #7700, #9141 ) ;
#14803=AXIS2_PLACEMENT_3D ( 'NONE', #6010, #250, #9505 ) ;
#14804=CIRCLE ( 'NONE', #1705, 59.49999999999999289 ) ;
#14805=EDGE_CURVE ( 'NONE', #1282, #13160, #13830, .T. ) ;
#14806=DIRECTION ( 'NONE',  ( 1.000000000000000000, 0.000000000000000000, 0.000000000000000000 ) ) ;
#14807=CARTESIAN_POINT ( 'NONE',  ( -69.08004447556112382, -68.68541276968802833, 10.49999999999999822 ) ) ;
#14808=CARTESIAN_POINT ( 'NONE',  ( -3.492805317593278058, 46.55633131742322917, -13.00000000000000178 ) ) ;
#14809=DIRECTION ( 'NONE',  ( -1.000000000000000000, 0.000000000000000000, 0.000000000000000000 ) ) ;
#14810=EDGE_CURVE ( 'NONE', #12421, #8030, #13576, .T. ) ;
#14811=VECTOR ( 'NONE', #5023, 1000.000000000000000 ) ;
#14813=ORIENTED_EDGE ( 'NONE', *, *, #11022, .F. ) ;
#14814=CARTESIAN_POINT ( 'NONE',  ( 70.71067811865438557, -70.71067811865511032, 8.000000000000000000 ) ) ;
#14815=AXIS2_PLACEMENT_3D ( 'NONE', #696, #3123, #626 ) ;
#14816=CIRCLE ( 'NONE', #9452, 52.50000000000000711 ) ;
#14817=CARTESIAN_POINT ( 'NONE',  ( 32.46576781417953583, -41.59008834022656487, 10.49999999999999822 ) ) ;
#14821=AXIS2_PLACEMENT_3D ( 'NONE', #2499, #4786, #7117 ) ;
#14823=CARTESIAN_POINT ( 'NONE',  ( -36.14014761921588104, 11.74264578624790190, -25.50000000000000355 ) ) ;
#14824=DIRECTION ( 'NONE',  ( 1.000000000000000000, 0.000000000000000000, 0.000000000000000000 ) ) ;
#14825=VECTOR ( 'NONE', #12805, 1000.000000000000000 ) ;
#14826=AXIS2_PLACEMENT_3D ( 'NONE', #5012, #442, #3866 ) ;
#14828=CARTESIAN_POINT ( 'NONE',  ( -33.48561063518626923, 47.21331623427104063, -13.00000000000000178 ) ) ;
#14829=CARTESIAN_POINT ( 'NONE',  ( 53.63365512954693770, -9.714003807513686084, 8.000000000000000000 ) ) ;
#14830=DIRECTION ( 'NONE',  ( -0.000000000000000000, -0.000000000000000000, -1.000000000000000000 ) ) ;
#14832=DIRECTION ( 'NONE',  ( 1.000000000000000000, -1.826024711554534012E-15, 0.000000000000000000 ) ) ;
#14833=EDGE_CURVE ( 'NONE', #9386, #1607, #6438, .T. ) ;
#14834=AXIS2_PLACEMENT_3D ( 'NONE', #8670, #5114, #10958 ) ;
#14836=EDGE_CURVE ( 'NONE', #13552, #3890, #11090, .T. ) ;
#14837=CARTESIAN_POINT ( 'NONE',  ( 13.71740939043365337, -51.19406879332061067, 8.000000000000000000 ) ) ;
#14838=DIRECTION ( 'NONE',  ( 0.000000000000000000, 0.000000000000000000, 1.000000000000000000 ) ) ;
#14839=AXIS2_PLACEMENT_3D ( 'NONE', #4663, #4810, #14148 ) ;
#14840=CARTESIAN_POINT ( 'NONE',  ( -89.61631465359441506, 37.12029293941468211, -8.000000000000000000 ) ) ;
#14842=DIRECTION ( 'NONE',  ( 1.000000000000000000, 0.000000000000000000, 0.000000000000000000 ) ) ;
#14844=EDGE_CURVE ( 'NONE', #10355, #4159, #9931, .T. ) ;
#14845=CARTESIAN_POINT ( 'NONE',  ( 29.49928053175900899, 45.83364790889059037, 8.000000000000000000 ) ) ;
#14846=ORIENTED_EDGE ( 'NONE', *, *, #10049, .T. ) ;
#14847=AXIS2_PLACEMENT_3D ( 'NONE', #871, #14689, #6534 ) ;
#14848=DIRECTION ( 'NONE',  ( 1.000000000000000000, 0.000000000000000000, 0.000000000000000000 ) ) ;
#14849=DIRECTION ( 'NONE',  ( 0.000000000000000000, 0.000000000000000000, -1.000000000000000000 ) ) ;
#14850=DIRECTION ( 'NONE',  ( 0.000000000000000000, 0.000000000000000000, 1.000000000000000000 ) ) ;
#14851=AXIS2_PLACEMENT_3D ( 'NONE', #13545, #6626, #10201 ) ;
#14852=CARTESIAN_POINT ( 'NONE',  ( -37.12029293941441210, -89.61631465359452875, -10.50000000000000000 ) ) ;
#14854=ORIENTED_EDGE ( 'NONE', *, *, #11259, .T. ) ;
#14856=EDGE_CURVE ( 'NONE', #1115, #13227, #767, .T. ) ;
#14859=CIRCLE ( 'NONE', #8297, 0.5000000000000004441 ) ;
#14860=DIRECTION ( 'NONE',  ( 1.000000000000000000, 0.000000000000000000, 0.000000000000000000 ) ) ;
#14865=AXIS2_PLACEMENT_3D ( 'NONE', #14001, #12784, #3595 ) ;
#14866=DIRECTION ( 'NONE',  ( -1.000000000000000000, 0.000000000000000000, 0.000000000000000000 ) ) ;
#14871=ORIENTED_EDGE ( 'NONE', *, *, #363, .F. ) ;
#14875=AXIS2_PLACEMENT_3D ( 'NONE', #10304, #9083, #1132 ) ;
#14876=ORIENTED_EDGE ( 'NONE', *, *, #13497, .F. ) ;
#14877=CIRCLE ( 'NONE', #9768, 0.5000000000000004441 ) ;
#14878=VERTEX_POINT ( 'NONE', #3191 ) ;
#14879=CARTESIAN_POINT ( 'NONE',  ( 9.917888187663120192, 52.54657765281190507, 8.000000000000000000 ) ) ;
#14882=ORIENTED_EDGE ( 'NONE', *, *, #13042, .F. ) ;
#14883=CARTESIAN_POINT ( 'NONE',  ( -37.02125851216292318, 90.10640870805768543, -13.00000000000000178 ) ) ;
#14884=DIRECTION ( 'NONE',  ( 1.000000000000000000, 0.000000000000000000, 0.000000000000000000 ) ) ;
#14886=DIRECTION ( 'NONE',  ( 0.000000000000000000, 0.000000000000000000, 1.000000000000000000 ) ) ;
#14887=CYLINDRICAL_SURFACE ( 'NONE', #12, 0.5000000000000004441 ) ;
#14888=CARTESIAN_POINT ( 'NONE',  ( 45.88839665196118744, -26.99988008862642630, 10.49999999999999822 ) ) ;
#14889=AXIS2_PLACEMENT_3D ( 'NONE', #8690, #8775, #10069 ) ;
#14890=ORIENTED_EDGE ( 'NONE', *, *, #5567, .T. ) ;
#14892=ORIENTED_EDGE ( 'NONE', *, *, #2845, .F. ) ;
#14893=AXIS2_PLACEMENT_3D ( 'NONE', #9337, #3430, #12546 ) ;
#14895=CARTESIAN_POINT ( 'NONE',  ( 0.000000000000000000, 0.000000000000000000, 10.50000000000000000 ) ) ;
#14896=CIRCLE ( 'NONE', #13434, 0.5000000000000022204 ) ;
#14897=ADVANCED_FACE ( 'NONE', ( #618 ), #5830, .T. ) ;
#14898=VERTEX_POINT ( 'NONE', #8187 ) ;
#14901=EDGE_CURVE ( 'NONE', #14021, #12633, #12624, .T. ) ;
#14904=AXIS2_PLACEMENT_3D ( 'NONE', #1100, #5779, #170 ) ;
#14905=CARTESIAN_POINT ( 'NONE',  ( -27.00670028307162340, -46.24878538001323136, -10.50000000000000000 ) ) ;
#14906=DIRECTION ( 'NONE',  ( 0.000000000000000000, 0.000000000000000000, -1.000000000000000000 ) ) ;
#14908=AXIS2_PLACEMENT_3D ( 'NONE', #8353, #1301, #10706 ) ;
#14912=ORIENTED_EDGE ( 'NONE', *, *, #7118, .F. ) ;
#14914=CARTESIAN_POINT ( 'NONE',  ( -53.26842454702436669, -11.55014193876159645, -13.00000000000000178 ) ) ;
#14915=CIRCLE ( 'NONE', #3741, 0.5000000000000004441 ) ;
#14916=CARTESIAN_POINT ( 'NONE',  ( 9.706953719245472456, 57.06275842387054098, 10.49999999999999822 ) ) ;
#14917=CIRCLE ( 'NONE', #8360, 3.000000000000002665 ) ;
#14919=AXIS2_PLACEMENT_3D ( 'NONE', #6106, #554, #8235 ) ;
#14920=CARTESIAN_POINT ( 'NONE',  ( -6.917888187662729393, -52.54657765281195481, 10.49999999999999822 ) ) ;
#14921=ORIENTED_EDGE ( 'NONE', *, *, #142, .F. ) ;
#14922=DIRECTION ( 'NONE',  ( 0.000000000000000000, 0.000000000000000000, 1.000000000000000000 ) ) ;
#14923=EDGE_LOOP ( 'NONE', ( #3689, #5880, #14548, #1973, #8659, #13727, #13014, #13968, #4456 ) ) ;
#14924=ADVANCED_FACE ( 'NONE', ( #9252 ), #14887, .F. ) ;
#14925=CARTESIAN_POINT ( 'NONE',  ( -42.04772703543551415, -32.26435573746212526, -13.00000000000000178 ) ) ;
#14927=CIRCLE ( 'NONE', #13967, 59.50000000000000000 ) ;
#14928=ADVANCED_FACE ( 'NONE', ( #11392 ), #9693, .T. ) ;
#14929=CYLINDRICAL_SURFACE ( 'NONE', #4613, 59.50000000000000000 ) ;
#14930=CARTESIAN_POINT ( 'NONE',  ( -36.52608637591512775, 92.55687898036946137, -8.000000000000000000 ) ) ;
#14931=VERTEX_POINT ( 'NONE', #11623 ) ;
#14933=VERTEX_POINT ( 'NONE', #11475 ) ;
#14935=CARTESIAN_POINT ( 'NONE',  ( -32.46576781417928714, 41.59008834022678514, 10.49999999999999822 ) ) ;
#14936=DIRECTION ( 'NONE',  ( 0.000000000000000000, 0.000000000000000000, 1.000000000000000000 ) ) ;
#14937=DIRECTION ( 'NONE',  ( 0.000000000000000000, 0.000000000000000000, -1.000000000000000000 ) ) ;
#14938=AXIS2_PLACEMENT_3D ( 'NONE', #3008, #814, #14711 ) ;
#14940=VERTEX_POINT ( 'NONE', #1148 ) ;
#14941=ADVANCED_FACE ( 'NONE', ( #9106 ), #6894, .F. ) ;
#14942=EDGE_LOOP ( 'NONE', ( #6029, #11944, #435, #10461 ) ) ;
#14944=DIRECTION ( 'NONE',  ( -1.000000000000000000, 0.000000000000000000, 0.000000000000000000 ) ) ;
#14945=DIRECTION ( 'NONE',  ( -1.000000000000000000, 0.000000000000000000, 0.000000000000000000 ) ) ;
#14947=DIRECTION ( 'NONE',  ( -0.000000000000000000, -0.000000000000000000, -1.000000000000000000 ) ) ;
#14949=ORIENTED_EDGE ( 'NONE', *, *, #7350, .T. ) ;
#14950=FACE_OUTER_BOUND ( 'NONE', #3321, .T. ) ;
#14951=ORIENTED_EDGE ( 'NONE', *, *, #125, .F. ) ;
#14952=EDGE_CURVE ( 'NONE', #5997, #11991, #8724, .T. ) ;
#14953=LINE ( 'NONE', #4549, #5200 ) ;
#14959=EDGE_LOOP ( 'NONE', ( #9925, #10814, #6373, #1313, #14654 ) ) ;
#14960=EDGE_CURVE ( 'NONE', #669, #215, #8257, .T. ) ;
#14962=CARTESIAN_POINT ( 'NONE',  ( -69.16568774265545017, 71.53347797788843820, 8.000000000000000000 ) ) ;
#14963=DIRECTION ( 'NONE',  ( -1.000000000000000000, 0.000000000000000000, 0.000000000000000000 ) ) ;
#14964=DIRECTION ( 'NONE',  ( 1.000000000000000000, 0.000000000000000000, 0.000000000000000000 ) ) ;
#14965=DIRECTION ( 'NONE',  ( -0.000000000000000000, -0.000000000000000000, 1.000000000000000000 ) ) ;
#14966=VECTOR ( 'NONE', #4321, 1000.000000000000000 ) ;
#14967=CARTESIAN_POINT ( 'NONE',  ( 0.000000000000000000, 0.000000000000000000, -25.50000000000000355 ) ) ;
#14969=AXIS2_PLACEMENT_3D ( 'NONE', #1758, #8655, #2826 ) ;
#14970=DIRECTION ( 'NONE',  ( -0.000000000000000000, -0.000000000000000000, -1.000000000000000000 ) ) ;
#14972=FACE_OUTER_BOUND ( 'NONE', #13747, .T. ) ;
#14973=ORIENTED_EDGE ( 'NONE', *, *, #11937, .F. ) ;
#14974=DIRECTION ( 'NONE',  ( 0.000000000000000000, 0.000000000000000000, 1.000000000000000000 ) ) ;
#14975=DIRECTION ( 'NONE',  ( 1.000000000000000000, 0.000000000000000000, 0.000000000000000000 ) ) ;
#14976=ORIENTED_EDGE ( 'NONE', *, *, #7922, .F. ) ;
#14977=DIRECTION ( 'NONE',  ( -0.000000000000000000, -0.000000000000000000, -1.000000000000000000 ) ) ;
#14978=CYLINDRICAL_SURFACE ( 'NONE', #13957, 59.50000000000000000 ) ;
#14979=LINE ( 'NONE', #12620, #13354 ) ;
#14980=DIRECTION ( 'NONE',  ( 0.000000000000000000, 0.000000000000000000, 1.000000000000000000 ) ) ;
#14981=ADVANCED_FACE ( 'NONE', ( #6736 ), #10841, .F. ) ;
#14983=ADVANCED_FACE ( 'NONE', ( #7339 ), #14566, .F. ) ;
#14985=FACE_OUTER_BOUND ( 'NONE', #1175, .T. ) ;
#14986=ORIENTED_EDGE ( 'NONE', *, *, #9427, .F. ) ;
#14989=CIRCLE ( 'NONE', #8428, 100.0000000000000000 ) ;
#14990=PLANE ( 'NONE',  #11967 ) ;
#14991=EDGE_CURVE ( 'NONE', #12263, #11561, #8416, .T. ) ;
#14992=DIRECTION ( 'NONE',  ( 1.000000000000000000, 0.000000000000000000, -0.000000000000000000 ) ) ;
#14993=ORIENTED_EDGE ( 'NONE', *, *, #14960, .F. ) ;
#14994=CARTESIAN_POINT ( 'NONE',  ( -57.06275842387042729, 9.706953719246069312, -13.00000000000000178 ) ) ;
#14995=ORIENTED_EDGE ( 'NONE', *, *, #1110, .F. ) ;
#14996=ADVANCED_FACE ( 'NONE', ( #3863 ), #8480, .T. ) ;
#14997=CARTESIAN_POINT ( 'NONE',  ( 97.00000000000000000, -3.384287605079545030E-13, 10.49999999999999822 ) ) ;
#14999=AXIS2_PLACEMENT_3D ( 'NONE', #13330, #8773, #10983 ) ;
#15000=CARTESIAN_POINT ( 'NONE',  ( 0.000000000000000000, 0.000000000000000000, -10.50000000000000000 ) ) ;
#15001=CARTESIAN_POINT ( 'NONE',  ( 100.0000000000000000, -1.224646799147353217E-14, -13.00000000000000178 ) ) ;
#15002=ORIENTED_EDGE ( 'NONE', *, *, #12141, .F. ) ;
#15003=EDGE_CURVE ( 'NONE', #9892, #2714, #14816, .T. ) ;
#15004=ORIENTED_EDGE ( 'NONE', *, *, #6971, .T. ) ;
#15005=ORIENTED_EDGE ( 'NONE', *, *, #10424, .F. ) ;
#15006=DIRECTION ( 'NONE',  ( 1.000000000000000000, 0.000000000000000000, 0.000000000000000000 ) ) ;
#15008=DIRECTION ( 'NONE',  ( 0.000000000000000000, 0.000000000000000000, 1.000000000000000000 ) ) ;
#15009=ORIENTED_EDGE ( 'NONE', *, *, #12386, .F. ) ;
#15010=EDGE_LOOP ( 'NONE', ( #752, #11481, #7344, #4868 ) ) ;
#15015=CYLINDRICAL_SURFACE ( 'NONE', #13492, 0.5000000000000073275 ) ;
#15016=DIRECTION ( 'NONE',  ( -0.000000000000000000, -0.000000000000000000, -1.000000000000000000 ) ) ;
#15017=ORIENTED_EDGE ( 'NONE', *, *, #12606, .T. ) ;
#15018=DIRECTION ( 'NONE',  ( 0.000000000000000000, 0.000000000000000000, 1.000000000000000000 ) ) ;
#15019=AXIS2_PLACEMENT_3D ( 'NONE', #10410, #166, #12778 ) ;
#15023=ORIENTED_EDGE ( 'NONE', *, *, #8905, .T. ) ;
#15024=VERTEX_POINT ( 'NONE', #2643 ) ;
#15029=DIRECTION ( 'NONE',  ( 0.000000000000000000, 0.000000000000000000, 1.000000000000000000 ) ) ;
ENDSEC;
END-ISO-10303-21;
